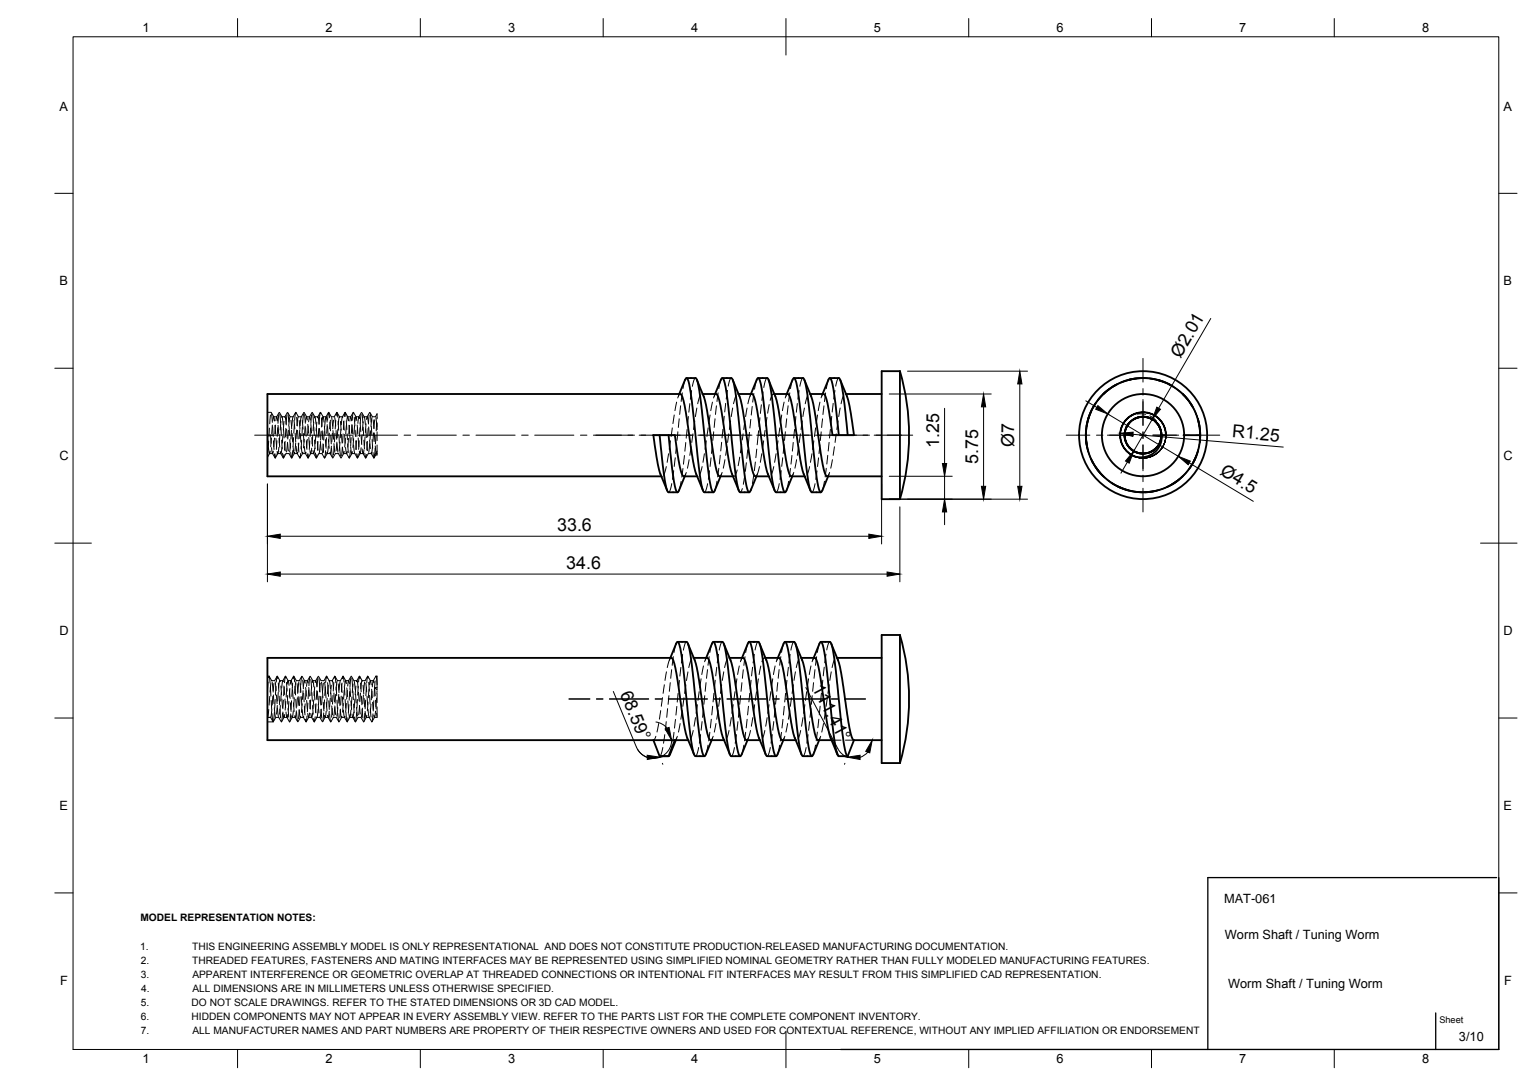
ISO-10303-21;
HEADER;
/* Generated by software containing ST-Developer
 * from STEP Tools, Inc. (www.steptools.com) 
 */

FILE_DESCRIPTION(
/* description */ ('', 'CAx-IF Rec.Pracs.---Representation and Presentation of Product Manufa
cturing Information (PMI)---4.0---2014-10-13'),
/* implementation_level */ '2;1');

FILE_NAME(
/* name */ 'Worm Shaft _ Tuning Worm.step',
/* time_stamp */ '2026-10-28T14:45:12+01:00',
/* author */ (''),
/* organization */ (''),
/* preprocessor_version */ 'ST-DEVELOPER v20.2',
/* originating_system */ 'Autodesk Translation Framework v15.17.0.0',
/* authorisation */ '');

FILE_SCHEMA (('AP242_MANAGED_MODEL_BASED_3D_ENGINEERING_MIM_LF { 1 0 10303 442 2 1 4 }'));
ENDSEC;

DATA;
#10=MECHANICAL_DESIGN_GEOMETRIC_PRESENTATION_REPRESENTATION('',(#258),#52164);
#232=SHAPE_REPRESENTATION_RELATIONSHIP('SRR','None',#52211,#245);
#245=ADVANCED_BREP_SHAPE_REPRESENTATION('',(#271),#52151);
#258=STYLED_ITEM('',(#52318),#271);
#271=MANIFOLD_SOLID_BREP('Body1',#9118);
#284=SPHERICAL_SURFACE('',#9300,12.5);
#288=FACE_BOUND('',#1072,.T.);
#289=FACE_BOUND('',#1091,.T.);
#323=B_SPLINE_SURFACE_WITH_KNOTS('',3,3,((#13144,#13145,#13146,#13147,#13148,
#13149,#13150,#13151,#13152,#13153,#13154,#13155,#13156,#13157,#13158,#13159,
#13160,#13161,#13162,#13163,#13164,#13165,#13166,#13167,#13168,#13169,#13170,
#13171,#13172,#13173,#13174,#13175,#13176,#13177,#13178),(#13179,#13180,
#13181,#13182,#13183,#13184,#13185,#13186,#13187,#13188,#13189,#13190,#13191,
#13192,#13193,#13194,#13195,#13196,#13197,#13198,#13199,#13200,#13201,#13202,
#13203,#13204,#13205,#13206,#13207,#13208,#13209,#13210,#13211,#13212,#13213),
(#13214,#13215,#13216,#13217,#13218,#13219,#13220,#13221,#13222,#13223,
#13224,#13225,#13226,#13227,#13228,#13229,#13230,#13231,#13232,#13233,#13234,
#13235,#13236,#13237,#13238,#13239,#13240,#13241,#13242,#13243,#13244,#13245,
#13246,#13247,#13248),(#13249,#13250,#13251,#13252,#13253,#13254,#13255,
#13256,#13257,#13258,#13259,#13260,#13261,#13262,#13263,#13264,#13265,#13266,
#13267,#13268,#13269,#13270,#13271,#13272,#13273,#13274,#13275,#13276,#13277,
#13278,#13279,#13280,#13281,#13282,#13283)),.UNSPECIFIED.,.F.,.F.,.F.,(4,
4),(4,1,1,1,1,1,1,1,1,1,1,1,1,1,1,1,1,1,1,1,1,1,1,1,1,1,1,1,1,1,1,1,4),
(0.3338579451982,1.029778418438),(-0.02,0.0125,0.045,0.0775,0.11,0.1425,
0.175,0.2075,0.24,0.2725,0.305,0.3375,0.37,0.4025,0.435,0.4675,0.5,0.5325,
0.565,0.5975,0.63,0.6625,0.695,0.7275,0.76,0.7925,0.825,0.8575,0.89,0.9225,
0.955,0.9875,1.02),.UNSPECIFIED.);
#324=B_SPLINE_SURFACE_WITH_KNOTS('',3,3,((#13372,#13373,#13374,#13375,#13376,
#13377,#13378,#13379,#13380,#13381,#13382,#13383,#13384,#13385,#13386,#13387,
#13388,#13389,#13390,#13391,#13392,#13393,#13394,#13395,#13396,#13397,#13398,
#13399,#13400,#13401,#13402,#13403,#13404,#13405,#13406),(#13407,#13408,
#13409,#13410,#13411,#13412,#13413,#13414,#13415,#13416,#13417,#13418,#13419,
#13420,#13421,#13422,#13423,#13424,#13425,#13426,#13427,#13428,#13429,#13430,
#13431,#13432,#13433,#13434,#13435,#13436,#13437,#13438,#13439,#13440,#13441),
(#13442,#13443,#13444,#13445,#13446,#13447,#13448,#13449,#13450,#13451,
#13452,#13453,#13454,#13455,#13456,#13457,#13458,#13459,#13460,#13461,#13462,
#13463,#13464,#13465,#13466,#13467,#13468,#13469,#13470,#13471,#13472,#13473,
#13474,#13475,#13476),(#13477,#13478,#13479,#13480,#13481,#13482,#13483,
#13484,#13485,#13486,#13487,#13488,#13489,#13490,#13491,#13492,#13493,#13494,
#13495,#13496,#13497,#13498,#13499,#13500,#13501,#13502,#13503,#13504,#13505,
#13506,#13507,#13508,#13509,#13510,#13511)),.UNSPECIFIED.,.F.,.F.,.F.,(4,
4),(4,1,1,1,1,1,1,1,1,1,1,1,1,1,1,1,1,1,1,1,1,1,1,1,1,1,1,1,1,1,1,1,4),
(0.3338579451982,1.029778418438),(-0.02,0.0125,0.045,0.0775,0.11,0.1425,
0.175,0.2075,0.24,0.2725,0.305,0.3375,0.37,0.4025,0.435,0.4675,0.5,0.5325,
0.565,0.5975,0.63,0.6625,0.695,0.7275,0.76,0.7925,0.825,0.8575,0.89,0.9225,
0.955,0.9875,1.02),.UNSPECIFIED.);
#325=B_SPLINE_SURFACE_WITH_KNOTS('',3,3,((#13626,#13627,#13628,#13629,#13630,
#13631,#13632,#13633,#13634,#13635,#13636,#13637,#13638,#13639,#13640,#13641,
#13642,#13643,#13644,#13645,#13646,#13647,#13648,#13649,#13650,#13651,#13652,
#13653,#13654,#13655,#13656,#13657,#13658,#13659,#13660),(#13661,#13662,
#13663,#13664,#13665,#13666,#13667,#13668,#13669,#13670,#13671,#13672,#13673,
#13674,#13675,#13676,#13677,#13678,#13679,#13680,#13681,#13682,#13683,#13684,
#13685,#13686,#13687,#13688,#13689,#13690,#13691,#13692,#13693,#13694,#13695),
(#13696,#13697,#13698,#13699,#13700,#13701,#13702,#13703,#13704,#13705,
#13706,#13707,#13708,#13709,#13710,#13711,#13712,#13713,#13714,#13715,#13716,
#13717,#13718,#13719,#13720,#13721,#13722,#13723,#13724,#13725,#13726,#13727,
#13728,#13729,#13730),(#13731,#13732,#13733,#13734,#13735,#13736,#13737,
#13738,#13739,#13740,#13741,#13742,#13743,#13744,#13745,#13746,#13747,#13748,
#13749,#13750,#13751,#13752,#13753,#13754,#13755,#13756,#13757,#13758,#13759,
#13760,#13761,#13762,#13763,#13764,#13765)),.UNSPECIFIED.,.F.,.F.,.F.,(4,
4),(4,1,1,1,1,1,1,1,1,1,1,1,1,1,1,1,1,1,1,1,1,1,1,1,1,1,1,1,1,1,1,1,4),
(-0.02977841843818,0.6661420548018),(-0.02,0.0125,0.045,0.0775,0.11,0.1425,
0.175,0.2075,0.24,0.2725,0.305,0.3375,0.37,0.4025,0.435,0.4675,0.5,0.5325,
0.565,0.5975,0.63,0.6625,0.695,0.7275,0.76,0.7925,0.825,0.8575,0.89,0.9225,
0.955,0.9875,1.02),.UNSPECIFIED.);
#326=B_SPLINE_SURFACE_WITH_KNOTS('',3,3,((#13854,#13855,#13856,#13857,#13858,
#13859,#13860,#13861,#13862,#13863,#13864,#13865,#13866,#13867,#13868,#13869,
#13870,#13871,#13872,#13873,#13874,#13875,#13876,#13877,#13878,#13879,#13880,
#13881,#13882,#13883,#13884,#13885,#13886,#13887,#13888),(#13889,#13890,
#13891,#13892,#13893,#13894,#13895,#13896,#13897,#13898,#13899,#13900,#13901,
#13902,#13903,#13904,#13905,#13906,#13907,#13908,#13909,#13910,#13911,#13912,
#13913,#13914,#13915,#13916,#13917,#13918,#13919,#13920,#13921,#13922,#13923),
(#13924,#13925,#13926,#13927,#13928,#13929,#13930,#13931,#13932,#13933,
#13934,#13935,#13936,#13937,#13938,#13939,#13940,#13941,#13942,#13943,#13944,
#13945,#13946,#13947,#13948,#13949,#13950,#13951,#13952,#13953,#13954,#13955,
#13956,#13957,#13958),(#13959,#13960,#13961,#13962,#13963,#13964,#13965,
#13966,#13967,#13968,#13969,#13970,#13971,#13972,#13973,#13974,#13975,#13976,
#13977,#13978,#13979,#13980,#13981,#13982,#13983,#13984,#13985,#13986,#13987,
#13988,#13989,#13990,#13991,#13992,#13993)),.UNSPECIFIED.,.F.,.F.,.F.,(4,
4),(4,1,1,1,1,1,1,1,1,1,1,1,1,1,1,1,1,1,1,1,1,1,1,1,1,1,1,1,1,1,1,1,4),
(-0.02977841843818,0.6661420548018),(-0.02,0.0125,0.045,0.0775,0.11,0.1425,
0.175,0.2075,0.24,0.2725,0.305,0.3375,0.37,0.4025,0.435,0.4675,0.5,0.5325,
0.565,0.5975,0.63,0.6625,0.695,0.7275,0.76,0.7925,0.825,0.8575,0.89,0.9225,
0.955,0.9875,1.02),.UNSPECIFIED.);
#327=B_SPLINE_SURFACE_WITH_KNOTS('',3,3,((#14080,#14081,#14082,#14083,#14084,
#14085,#14086,#14087,#14088,#14089,#14090,#14091,#14092,#14093,#14094,#14095,
#14096,#14097,#14098,#14099,#14100,#14101,#14102,#14103,#14104,#14105,#14106,
#14107,#14108,#14109,#14110,#14111,#14112,#14113,#14114),(#14115,#14116,
#14117,#14118,#14119,#14120,#14121,#14122,#14123,#14124,#14125,#14126,#14127,
#14128,#14129,#14130,#14131,#14132,#14133,#14134,#14135,#14136,#14137,#14138,
#14139,#14140,#14141,#14142,#14143,#14144,#14145,#14146,#14147,#14148,#14149),
(#14150,#14151,#14152,#14153,#14154,#14155,#14156,#14157,#14158,#14159,
#14160,#14161,#14162,#14163,#14164,#14165,#14166,#14167,#14168,#14169,#14170,
#14171,#14172,#14173,#14174,#14175,#14176,#14177,#14178,#14179,#14180,#14181,
#14182,#14183,#14184),(#14185,#14186,#14187,#14188,#14189,#14190,#14191,
#14192,#14193,#14194,#14195,#14196,#14197,#14198,#14199,#14200,#14201,#14202,
#14203,#14204,#14205,#14206,#14207,#14208,#14209,#14210,#14211,#14212,#14213,
#14214,#14215,#14216,#14217,#14218,#14219)),.UNSPECIFIED.,.F.,.F.,.F.,(4,
4),(4,1,1,1,1,1,1,1,1,1,1,1,1,1,1,1,1,1,1,1,1,1,1,1,1,1,1,1,1,1,1,1,4),
(-0.1795055630679,1.179505563068),(-0.02,0.0125,0.045,0.0775,0.11,0.1425,
0.175,0.2075,0.24,0.2725,0.305,0.3375,0.37,0.4025,0.435,0.4675,0.5,0.5325,
0.565,0.5975,0.63,0.6625,0.695,0.7275,0.76,0.7925,0.825,0.8575,0.89,0.9225,
0.955,0.9875,1.02),.UNSPECIFIED.);
#328=B_SPLINE_SURFACE_WITH_KNOTS('',3,3,((#14625,#14626,#14627,#14628,#14629,
#14630,#14631,#14632,#14633,#14634,#14635,#14636,#14637,#14638,#14639,#14640,
#14641,#14642,#14643,#14644,#14645,#14646,#14647,#14648,#14649,#14650,#14651,
#14652,#14653,#14654,#14655,#14656,#14657,#14658,#14659),(#14660,#14661,
#14662,#14663,#14664,#14665,#14666,#14667,#14668,#14669,#14670,#14671,#14672,
#14673,#14674,#14675,#14676,#14677,#14678,#14679,#14680,#14681,#14682,#14683,
#14684,#14685,#14686,#14687,#14688,#14689,#14690,#14691,#14692,#14693,#14694),
(#14695,#14696,#14697,#14698,#14699,#14700,#14701,#14702,#14703,#14704,
#14705,#14706,#14707,#14708,#14709,#14710,#14711,#14712,#14713,#14714,#14715,
#14716,#14717,#14718,#14719,#14720,#14721,#14722,#14723,#14724,#14725,#14726,
#14727,#14728,#14729),(#14730,#14731,#14732,#14733,#14734,#14735,#14736,
#14737,#14738,#14739,#14740,#14741,#14742,#14743,#14744,#14745,#14746,#14747,
#14748,#14749,#14750,#14751,#14752,#14753,#14754,#14755,#14756,#14757,#14758,
#14759,#14760,#14761,#14762,#14763,#14764)),.UNSPECIFIED.,.F.,.F.,.F.,(4,
4),(4,1,1,1,1,1,1,1,1,1,1,1,1,1,1,1,1,1,1,1,1,1,1,1,1,1,1,1,1,1,1,1,4),
(-0.1795055630679,1.179505563068),(-0.02,0.0125,0.045,0.0775,0.11,0.1425,
0.175,0.2075,0.24,0.2725,0.305,0.3375,0.37,0.4025,0.435,0.4675,0.5,0.5325,
0.565,0.5975,0.63,0.6625,0.695,0.7275,0.76,0.7925,0.825,0.8575,0.89,0.9225,
0.955,0.9875,1.02),.UNSPECIFIED.);
#329=B_SPLINE_SURFACE_WITH_KNOTS('',3,3,((#14766,#14767,#14768,#14769,#14770,
#14771,#14772,#14773,#14774,#14775,#14776,#14777,#14778,#14779,#14780,#14781,
#14782,#14783,#14784,#14785,#14786,#14787,#14788,#14789,#14790,#14791,#14792,
#14793,#14794,#14795,#14796,#14797,#14798,#14799,#14800),(#14801,#14802,
#14803,#14804,#14805,#14806,#14807,#14808,#14809,#14810,#14811,#14812,#14813,
#14814,#14815,#14816,#14817,#14818,#14819,#14820,#14821,#14822,#14823,#14824,
#14825,#14826,#14827,#14828,#14829,#14830,#14831,#14832,#14833,#14834,#14835),
(#14836,#14837,#14838,#14839,#14840,#14841,#14842,#14843,#14844,#14845,
#14846,#14847,#14848,#14849,#14850,#14851,#14852,#14853,#14854,#14855,#14856,
#14857,#14858,#14859,#14860,#14861,#14862,#14863,#14864,#14865,#14866,#14867,
#14868,#14869,#14870),(#14871,#14872,#14873,#14874,#14875,#14876,#14877,
#14878,#14879,#14880,#14881,#14882,#14883,#14884,#14885,#14886,#14887,#14888,
#14889,#14890,#14891,#14892,#14893,#14894,#14895,#14896,#14897,#14898,#14899,
#14900,#14901,#14902,#14903,#14904,#14905)),.UNSPECIFIED.,.F.,.F.,.F.,(4,
4),(4,1,1,1,1,1,1,1,1,1,1,1,1,1,1,1,1,1,1,1,1,1,1,1,1,1,1,1,1,1,1,1,4),
(-0.1795055630679,1.179505563068),(-0.02,0.0125,0.045,0.0775,0.11,0.1425,
0.175,0.2075,0.24,0.2725,0.305,0.3375,0.37,0.4025,0.435,0.4675,0.5,0.5325,
0.565,0.5975,0.63,0.6625,0.695,0.7275,0.76,0.7925,0.825,0.8575,0.89,0.9225,
0.955,0.9875,1.02),.UNSPECIFIED.);
#330=B_SPLINE_SURFACE_WITH_KNOTS('',3,3,((#15309,#15310,#15311,#15312,#15313,
#15314,#15315,#15316,#15317,#15318,#15319,#15320,#15321,#15322,#15323,#15324,
#15325,#15326,#15327,#15328,#15329,#15330,#15331,#15332,#15333,#15334,#15335,
#15336,#15337,#15338,#15339,#15340,#15341,#15342,#15343),(#15344,#15345,
#15346,#15347,#15348,#15349,#15350,#15351,#15352,#15353,#15354,#15355,#15356,
#15357,#15358,#15359,#15360,#15361,#15362,#15363,#15364,#15365,#15366,#15367,
#15368,#15369,#15370,#15371,#15372,#15373,#15374,#15375,#15376,#15377,#15378),
(#15379,#15380,#15381,#15382,#15383,#15384,#15385,#15386,#15387,#15388,
#15389,#15390,#15391,#15392,#15393,#15394,#15395,#15396,#15397,#15398,#15399,
#15400,#15401,#15402,#15403,#15404,#15405,#15406,#15407,#15408,#15409,#15410,
#15411,#15412,#15413),(#15414,#15415,#15416,#15417,#15418,#15419,#15420,
#15421,#15422,#15423,#15424,#15425,#15426,#15427,#15428,#15429,#15430,#15431,
#15432,#15433,#15434,#15435,#15436,#15437,#15438,#15439,#15440,#15441,#15442,
#15443,#15444,#15445,#15446,#15447,#15448)),.UNSPECIFIED.,.F.,.F.,.F.,(4,
4),(4,1,1,1,1,1,1,1,1,1,1,1,1,1,1,1,1,1,1,1,1,1,1,1,1,1,1,1,1,1,1,1,4),
(-0.1795055630679,1.179505563068),(-0.02,0.0125,0.045,0.0775,0.11,0.1425,
0.175,0.2075,0.24,0.2725,0.305,0.3375,0.37,0.4025,0.435,0.4675,0.5,0.5325,
0.565,0.5975,0.63,0.6625,0.695,0.7275,0.76,0.7925,0.825,0.8575,0.89,0.9225,
0.955,0.9875,1.02),.UNSPECIFIED.);
#331=B_SPLINE_SURFACE_WITH_KNOTS('',3,3,((#15538,#15539,#15540,#15541,#15542,
#15543,#15544,#15545,#15546,#15547,#15548,#15549,#15550,#15551,#15552,#15553,
#15554,#15555,#15556,#15557,#15558,#15559,#15560,#15561,#15562,#15563,#15564,
#15565,#15566,#15567,#15568,#15569,#15570,#15571,#15572),(#15573,#15574,
#15575,#15576,#15577,#15578,#15579,#15580,#15581,#15582,#15583,#15584,#15585,
#15586,#15587,#15588,#15589,#15590,#15591,#15592,#15593,#15594,#15595,#15596,
#15597,#15598,#15599,#15600,#15601,#15602,#15603,#15604,#15605,#15606,#15607),
(#15608,#15609,#15610,#15611,#15612,#15613,#15614,#15615,#15616,#15617,
#15618,#15619,#15620,#15621,#15622,#15623,#15624,#15625,#15626,#15627,#15628,
#15629,#15630,#15631,#15632,#15633,#15634,#15635,#15636,#15637,#15638,#15639,
#15640,#15641,#15642),(#15643,#15644,#15645,#15646,#15647,#15648,#15649,
#15650,#15651,#15652,#15653,#15654,#15655,#15656,#15657,#15658,#15659,#15660,
#15661,#15662,#15663,#15664,#15665,#15666,#15667,#15668,#15669,#15670,#15671,
#15672,#15673,#15674,#15675,#15676,#15677)),.UNSPECIFIED.,.F.,.F.,.F.,(4,
4),(4,1,1,1,1,1,1,1,1,1,1,1,1,1,1,1,1,1,1,1,1,1,1,1,1,1,1,1,1,1,1,1,4),
(-0.1560934940397,1.15609349404),(-0.02,0.0125,0.045,0.0775,0.11,0.1425,
0.175,0.2075,0.24,0.2725,0.305,0.3375,0.37,0.4025,0.435,0.4675,0.5,0.5325,
0.565,0.5975,0.63,0.6625,0.695,0.7275,0.76,0.7925,0.825,0.8575,0.89,0.9225,
0.955,0.9875,1.02),.UNSPECIFIED.);
#332=B_SPLINE_SURFACE_WITH_KNOTS('',3,3,((#15921,#15922,#15923,#15924,#15925,
#15926,#15927,#15928,#15929,#15930,#15931,#15932,#15933,#15934,#15935,#15936,
#15937,#15938,#15939,#15940,#15941,#15942,#15943,#15944,#15945,#15946,#15947,
#15948,#15949,#15950,#15951,#15952,#15953,#15954,#15955),(#15956,#15957,
#15958,#15959,#15960,#15961,#15962,#15963,#15964,#15965,#15966,#15967,#15968,
#15969,#15970,#15971,#15972,#15973,#15974,#15975,#15976,#15977,#15978,#15979,
#15980,#15981,#15982,#15983,#15984,#15985,#15986,#15987,#15988,#15989,#15990),
(#15991,#15992,#15993,#15994,#15995,#15996,#15997,#15998,#15999,#16000,
#16001,#16002,#16003,#16004,#16005,#16006,#16007,#16008,#16009,#16010,#16011,
#16012,#16013,#16014,#16015,#16016,#16017,#16018,#16019,#16020,#16021,#16022,
#16023,#16024,#16025),(#16026,#16027,#16028,#16029,#16030,#16031,#16032,
#16033,#16034,#16035,#16036,#16037,#16038,#16039,#16040,#16041,#16042,#16043,
#16044,#16045,#16046,#16047,#16048,#16049,#16050,#16051,#16052,#16053,#16054,
#16055,#16056,#16057,#16058,#16059,#16060)),.UNSPECIFIED.,.F.,.F.,.F.,(4,
4),(4,1,1,1,1,1,1,1,1,1,1,1,1,1,1,1,1,1,1,1,1,1,1,1,1,1,1,1,1,1,1,1,4),
(-0.1560934940397,1.15609349404),(-0.02,0.0125,0.045,0.0775,0.11,0.1425,
0.175,0.2075,0.24,0.2725,0.305,0.3375,0.37,0.4025,0.435,0.4675,0.5,0.5325,
0.565,0.5975,0.63,0.6625,0.695,0.7275,0.76,0.7925,0.825,0.8575,0.89,0.9225,
0.955,0.9875,1.02),.UNSPECIFIED.);
#333=B_SPLINE_SURFACE_WITH_KNOTS('',3,3,((#16228,#16229,#16230,#16231,#16232,
#16233,#16234,#16235,#16236,#16237,#16238,#16239,#16240,#16241,#16242,#16243,
#16244,#16245,#16246,#16247,#16248,#16249,#16250,#16251,#16252,#16253,#16254,
#16255,#16256,#16257,#16258,#16259,#16260,#16261,#16262),(#16263,#16264,
#16265,#16266,#16267,#16268,#16269,#16270,#16271,#16272,#16273,#16274,#16275,
#16276,#16277,#16278,#16279,#16280,#16281,#16282,#16283,#16284,#16285,#16286,
#16287,#16288,#16289,#16290,#16291,#16292,#16293,#16294,#16295,#16296,#16297),
(#16298,#16299,#16300,#16301,#16302,#16303,#16304,#16305,#16306,#16307,
#16308,#16309,#16310,#16311,#16312,#16313,#16314,#16315,#16316,#16317,#16318,
#16319,#16320,#16321,#16322,#16323,#16324,#16325,#16326,#16327,#16328,#16329,
#16330,#16331,#16332),(#16333,#16334,#16335,#16336,#16337,#16338,#16339,
#16340,#16341,#16342,#16343,#16344,#16345,#16346,#16347,#16348,#16349,#16350,
#16351,#16352,#16353,#16354,#16355,#16356,#16357,#16358,#16359,#16360,#16361,
#16362,#16363,#16364,#16365,#16366,#16367)),.UNSPECIFIED.,.F.,.F.,.F.,(4,
4),(4,1,1,1,1,1,1,1,1,1,1,1,1,1,1,1,1,1,1,1,1,1,1,1,1,1,1,1,1,1,1,1,4),
(-0.2613852056804,1.26138520568),(-0.02,0.0125,0.045,0.0775,0.11,0.1425,
0.175,0.2075,0.24,0.2725,0.305,0.3375,0.37,0.4025,0.435,0.4675,0.5,0.5325,
0.565,0.5975,0.63,0.6625,0.695,0.7275,0.76,0.7925,0.825,0.8575,0.89,0.9225,
0.955,0.9875,1.02),.UNSPECIFIED.);
#334=B_SPLINE_SURFACE_WITH_KNOTS('',3,3,((#16369,#16370,#16371,#16372,#16373,
#16374,#16375,#16376,#16377,#16378,#16379,#16380,#16381,#16382,#16383,#16384,
#16385,#16386,#16387,#16388,#16389,#16390,#16391,#16392,#16393,#16394,#16395,
#16396,#16397,#16398,#16399,#16400,#16401,#16402,#16403),(#16404,#16405,
#16406,#16407,#16408,#16409,#16410,#16411,#16412,#16413,#16414,#16415,#16416,
#16417,#16418,#16419,#16420,#16421,#16422,#16423,#16424,#16425,#16426,#16427,
#16428,#16429,#16430,#16431,#16432,#16433,#16434,#16435,#16436,#16437,#16438),
(#16439,#16440,#16441,#16442,#16443,#16444,#16445,#16446,#16447,#16448,
#16449,#16450,#16451,#16452,#16453,#16454,#16455,#16456,#16457,#16458,#16459,
#16460,#16461,#16462,#16463,#16464,#16465,#16466,#16467,#16468,#16469,#16470,
#16471,#16472,#16473),(#16474,#16475,#16476,#16477,#16478,#16479,#16480,
#16481,#16482,#16483,#16484,#16485,#16486,#16487,#16488,#16489,#16490,#16491,
#16492,#16493,#16494,#16495,#16496,#16497,#16498,#16499,#16500,#16501,#16502,
#16503,#16504,#16505,#16506,#16507,#16508)),.UNSPECIFIED.,.F.,.F.,.F.,(4,
4),(4,1,1,1,1,1,1,1,1,1,1,1,1,1,1,1,1,1,1,1,1,1,1,1,1,1,1,1,1,1,1,1,4),
(-0.2613852056804,1.26138520568),(-0.02,0.0125,0.045,0.0775,0.11,0.1425,
0.175,0.2075,0.24,0.2725,0.305,0.3375,0.37,0.4025,0.435,0.4675,0.5,0.5325,
0.565,0.5975,0.63,0.6625,0.695,0.7275,0.76,0.7925,0.825,0.8575,0.89,0.9225,
0.955,0.9875,1.02),.UNSPECIFIED.);
#335=B_SPLINE_SURFACE_WITH_KNOTS('',3,3,((#16732,#16733,#16734,#16735,#16736,
#16737,#16738,#16739,#16740,#16741,#16742,#16743,#16744,#16745,#16746,#16747,
#16748,#16749,#16750,#16751,#16752,#16753,#16754,#16755,#16756,#16757,#16758,
#16759,#16760,#16761,#16762,#16763,#16764,#16765,#16766),(#16767,#16768,
#16769,#16770,#16771,#16772,#16773,#16774,#16775,#16776,#16777,#16778,#16779,
#16780,#16781,#16782,#16783,#16784,#16785,#16786,#16787,#16788,#16789,#16790,
#16791,#16792,#16793,#16794,#16795,#16796,#16797,#16798,#16799,#16800,#16801),
(#16802,#16803,#16804,#16805,#16806,#16807,#16808,#16809,#16810,#16811,
#16812,#16813,#16814,#16815,#16816,#16817,#16818,#16819,#16820,#16821,#16822,
#16823,#16824,#16825,#16826,#16827,#16828,#16829,#16830,#16831,#16832,#16833,
#16834,#16835,#16836),(#16837,#16838,#16839,#16840,#16841,#16842,#16843,
#16844,#16845,#16846,#16847,#16848,#16849,#16850,#16851,#16852,#16853,#16854,
#16855,#16856,#16857,#16858,#16859,#16860,#16861,#16862,#16863,#16864,#16865,
#16866,#16867,#16868,#16869,#16870,#16871)),.UNSPECIFIED.,.F.,.F.,.F.,(4,
4),(4,1,1,1,1,1,1,1,1,1,1,1,1,1,1,1,1,1,1,1,1,1,1,1,1,1,1,1,1,1,1,1,4),
(-0.1560934940397,1.15609349404),(-0.02,0.0125,0.045,0.0775,0.11,0.1425,
0.175,0.2075,0.24,0.2725,0.305,0.3375,0.37,0.4025,0.435,0.4675,0.5,0.5325,
0.565,0.5975,0.63,0.6625,0.695,0.7275,0.76,0.7925,0.825,0.8575,0.89,0.9225,
0.955,0.9875,1.02),.UNSPECIFIED.);
#336=B_SPLINE_SURFACE_WITH_KNOTS('',3,3,((#17004,#17005,#17006,#17007,#17008,
#17009,#17010,#17011,#17012,#17013,#17014,#17015,#17016,#17017,#17018,#17019,
#17020,#17021,#17022,#17023,#17024,#17025,#17026,#17027,#17028,#17029,#17030,
#17031,#17032,#17033,#17034,#17035,#17036,#17037,#17038),(#17039,#17040,
#17041,#17042,#17043,#17044,#17045,#17046,#17047,#17048,#17049,#17050,#17051,
#17052,#17053,#17054,#17055,#17056,#17057,#17058,#17059,#17060,#17061,#17062,
#17063,#17064,#17065,#17066,#17067,#17068,#17069,#17070,#17071,#17072,#17073),
(#17074,#17075,#17076,#17077,#17078,#17079,#17080,#17081,#17082,#17083,
#17084,#17085,#17086,#17087,#17088,#17089,#17090,#17091,#17092,#17093,#17094,
#17095,#17096,#17097,#17098,#17099,#17100,#17101,#17102,#17103,#17104,#17105,
#17106,#17107,#17108),(#17109,#17110,#17111,#17112,#17113,#17114,#17115,
#17116,#17117,#17118,#17119,#17120,#17121,#17122,#17123,#17124,#17125,#17126,
#17127,#17128,#17129,#17130,#17131,#17132,#17133,#17134,#17135,#17136,#17137,
#17138,#17139,#17140,#17141,#17142,#17143)),.UNSPECIFIED.,.F.,.F.,.F.,(4,
4),(4,1,1,1,1,1,1,1,1,1,1,1,1,1,1,1,1,1,1,1,1,1,1,1,1,1,1,1,1,1,1,1,4),
(-0.1560934940397,1.15609349404),(-0.02,0.0125,0.045,0.0775,0.11,0.1425,
0.175,0.2075,0.24,0.2725,0.305,0.3375,0.37,0.4025,0.435,0.4675,0.5,0.5325,
0.565,0.5975,0.63,0.6625,0.695,0.7275,0.76,0.7925,0.825,0.8575,0.89,0.9225,
0.955,0.9875,1.02),.UNSPECIFIED.);
#337=B_SPLINE_SURFACE_WITH_KNOTS('',3,3,((#17202,#17203,#17204,#17205,#17206,
#17207,#17208,#17209,#17210,#17211,#17212,#17213,#17214,#17215,#17216,#17217,
#17218,#17219,#17220,#17221,#17222,#17223,#17224,#17225,#17226,#17227,#17228,
#17229,#17230,#17231,#17232,#17233,#17234,#17235,#17236),(#17237,#17238,
#17239,#17240,#17241,#17242,#17243,#17244,#17245,#17246,#17247,#17248,#17249,
#17250,#17251,#17252,#17253,#17254,#17255,#17256,#17257,#17258,#17259,#17260,
#17261,#17262,#17263,#17264,#17265,#17266,#17267,#17268,#17269,#17270,#17271),
(#17272,#17273,#17274,#17275,#17276,#17277,#17278,#17279,#17280,#17281,
#17282,#17283,#17284,#17285,#17286,#17287,#17288,#17289,#17290,#17291,#17292,
#17293,#17294,#17295,#17296,#17297,#17298,#17299,#17300,#17301,#17302,#17303,
#17304,#17305,#17306),(#17307,#17308,#17309,#17310,#17311,#17312,#17313,
#17314,#17315,#17316,#17317,#17318,#17319,#17320,#17321,#17322,#17323,#17324,
#17325,#17326,#17327,#17328,#17329,#17330,#17331,#17332,#17333,#17334,#17335,
#17336,#17337,#17338,#17339,#17340,#17341)),.UNSPECIFIED.,.F.,.F.,.F.,(4,
4),(4,1,1,1,1,1,1,1,1,1,1,1,1,1,1,1,1,1,1,1,1,1,1,1,1,1,1,1,1,1,1,1,4),
(-0.1560934940397,1.15609349404),(-0.02,0.0125,0.045,0.0775,0.11,0.1425,
0.175,0.2075,0.24,0.2725,0.305,0.3375,0.37,0.4025,0.435,0.4675,0.5,0.5325,
0.565,0.5975,0.63,0.6625,0.695,0.7275,0.76,0.7925,0.825,0.8575,0.89,0.9225,
0.955,0.9875,1.02),.UNSPECIFIED.);
#338=B_SPLINE_SURFACE_WITH_KNOTS('',3,3,((#17618,#17619,#17620,#17621,#17622,
#17623,#17624,#17625,#17626,#17627,#17628,#17629,#17630,#17631,#17632,#17633,
#17634,#17635,#17636,#17637,#17638,#17639,#17640,#17641,#17642,#17643,#17644,
#17645,#17646,#17647,#17648,#17649,#17650,#17651,#17652),(#17653,#17654,
#17655,#17656,#17657,#17658,#17659,#17660,#17661,#17662,#17663,#17664,#17665,
#17666,#17667,#17668,#17669,#17670,#17671,#17672,#17673,#17674,#17675,#17676,
#17677,#17678,#17679,#17680,#17681,#17682,#17683,#17684,#17685,#17686,#17687),
(#17688,#17689,#17690,#17691,#17692,#17693,#17694,#17695,#17696,#17697,
#17698,#17699,#17700,#17701,#17702,#17703,#17704,#17705,#17706,#17707,#17708,
#17709,#17710,#17711,#17712,#17713,#17714,#17715,#17716,#17717,#17718,#17719,
#17720,#17721,#17722),(#17723,#17724,#17725,#17726,#17727,#17728,#17729,
#17730,#17731,#17732,#17733,#17734,#17735,#17736,#17737,#17738,#17739,#17740,
#17741,#17742,#17743,#17744,#17745,#17746,#17747,#17748,#17749,#17750,#17751,
#17752,#17753,#17754,#17755,#17756,#17757)),.UNSPECIFIED.,.F.,.F.,.F.,(4,
4),(4,1,1,1,1,1,1,1,1,1,1,1,1,1,1,1,1,1,1,1,1,1,1,1,1,1,1,1,1,1,1,1,4),
(-0.1560934940397,1.15609349404),(-0.02,0.0125,0.045,0.0775,0.11,0.1425,
0.175,0.2075,0.24,0.2725,0.305,0.3375,0.37,0.4025,0.435,0.4675,0.5,0.5325,
0.565,0.5975,0.63,0.6625,0.695,0.7275,0.76,0.7925,0.825,0.8575,0.89,0.9225,
0.955,0.9875,1.02),.UNSPECIFIED.);
#339=B_SPLINE_SURFACE_WITH_KNOTS('',3,3,((#17870,#17871,#17872,#17873,#17874,
#17875,#17876,#17877,#17878,#17879,#17880,#17881,#17882,#17883,#17884,#17885,
#17886,#17887,#17888,#17889,#17890,#17891,#17892,#17893,#17894,#17895,#17896,
#17897,#17898,#17899,#17900,#17901,#17902,#17903,#17904),(#17905,#17906,
#17907,#17908,#17909,#17910,#17911,#17912,#17913,#17914,#17915,#17916,#17917,
#17918,#17919,#17920,#17921,#17922,#17923,#17924,#17925,#17926,#17927,#17928,
#17929,#17930,#17931,#17932,#17933,#17934,#17935,#17936,#17937,#17938,#17939),
(#17940,#17941,#17942,#17943,#17944,#17945,#17946,#17947,#17948,#17949,
#17950,#17951,#17952,#17953,#17954,#17955,#17956,#17957,#17958,#17959,#17960,
#17961,#17962,#17963,#17964,#17965,#17966,#17967,#17968,#17969,#17970,#17971,
#17972,#17973,#17974),(#17975,#17976,#17977,#17978,#17979,#17980,#17981,
#17982,#17983,#17984,#17985,#17986,#17987,#17988,#17989,#17990,#17991,#17992,
#17993,#17994,#17995,#17996,#17997,#17998,#17999,#18000,#18001,#18002,#18003,
#18004,#18005,#18006,#18007,#18008,#18009)),.UNSPECIFIED.,.F.,.F.,.F.,(4,
4),(4,1,1,1,1,1,1,1,1,1,1,1,1,1,1,1,1,1,1,1,1,1,1,1,1,1,1,1,1,1,1,1,4),
(-0.1560934940397,1.15609349404),(-0.02,0.0125,0.045,0.0775,0.11,0.1425,
0.175,0.2075,0.24,0.2725,0.305,0.3375,0.37,0.4025,0.435,0.4675,0.5,0.5325,
0.565,0.5975,0.63,0.6625,0.695,0.7275,0.76,0.7925,0.825,0.8575,0.89,0.9225,
0.955,0.9875,1.02),.UNSPECIFIED.);
#340=B_SPLINE_SURFACE_WITH_KNOTS('',3,3,((#18261,#18262,#18263,#18264,#18265,
#18266,#18267,#18268,#18269,#18270,#18271,#18272,#18273,#18274,#18275,#18276,
#18277,#18278,#18279,#18280,#18281,#18282,#18283,#18284,#18285,#18286,#18287,
#18288,#18289,#18290,#18291,#18292,#18293,#18294,#18295),(#18296,#18297,
#18298,#18299,#18300,#18301,#18302,#18303,#18304,#18305,#18306,#18307,#18308,
#18309,#18310,#18311,#18312,#18313,#18314,#18315,#18316,#18317,#18318,#18319,
#18320,#18321,#18322,#18323,#18324,#18325,#18326,#18327,#18328,#18329,#18330),
(#18331,#18332,#18333,#18334,#18335,#18336,#18337,#18338,#18339,#18340,
#18341,#18342,#18343,#18344,#18345,#18346,#18347,#18348,#18349,#18350,#18351,
#18352,#18353,#18354,#18355,#18356,#18357,#18358,#18359,#18360,#18361,#18362,
#18363,#18364,#18365),(#18366,#18367,#18368,#18369,#18370,#18371,#18372,
#18373,#18374,#18375,#18376,#18377,#18378,#18379,#18380,#18381,#18382,#18383,
#18384,#18385,#18386,#18387,#18388,#18389,#18390,#18391,#18392,#18393,#18394,
#18395,#18396,#18397,#18398,#18399,#18400)),.UNSPECIFIED.,.F.,.F.,.F.,(4,
4),(4,1,1,1,1,1,1,1,1,1,1,1,1,1,1,1,1,1,1,1,1,1,1,1,1,1,1,1,1,1,1,1,4),
(-0.1560934940397,1.15609349404),(-0.0177116462091,0.01106977888069,0.03985120397047,
0.06863262906025,0.09741405415003,0.1261954792398,0.1549769043296,0.1837583294194,
0.2125397545092,0.2413211795989,0.2701026046887,0.2988840297785,0.3276654548683,
0.3564468799581,0.3852283050479,0.4140097301376,0.4427911552274,0.4715725803172,
0.500354005407,0.5291354304968,0.5579168555866,0.5866982806763,0.6154797057661,
0.6442611308559,0.6730425559457,0.7018239810355,0.7306054061252,0.759386831215,
0.7881682563048,0.8169496813946,0.8457311064844,0.8745125315742,0.9032939566639),
 .UNSPECIFIED.);
#341=B_SPLINE_SURFACE_WITH_KNOTS('',3,3,((#18688,#18689,#18690,#18691,#18692,
#18693,#18694,#18695,#18696,#18697,#18698,#18699,#18700,#18701,#18702,#18703,
#18704,#18705,#18706,#18707,#18708,#18709,#18710,#18711,#18712,#18713,#18714,
#18715,#18716,#18717,#18718,#18719,#18720,#18721,#18722),(#18723,#18724,
#18725,#18726,#18727,#18728,#18729,#18730,#18731,#18732,#18733,#18734,#18735,
#18736,#18737,#18738,#18739,#18740,#18741,#18742,#18743,#18744,#18745,#18746,
#18747,#18748,#18749,#18750,#18751,#18752,#18753,#18754,#18755,#18756,#18757),
(#18758,#18759,#18760,#18761,#18762,#18763,#18764,#18765,#18766,#18767,
#18768,#18769,#18770,#18771,#18772,#18773,#18774,#18775,#18776,#18777,#18778,
#18779,#18780,#18781,#18782,#18783,#18784,#18785,#18786,#18787,#18788,#18789,
#18790,#18791,#18792),(#18793,#18794,#18795,#18796,#18797,#18798,#18799,
#18800,#18801,#18802,#18803,#18804,#18805,#18806,#18807,#18808,#18809,#18810,
#18811,#18812,#18813,#18814,#18815,#18816,#18817,#18818,#18819,#18820,#18821,
#18822,#18823,#18824,#18825,#18826,#18827)),.UNSPECIFIED.,.F.,.F.,.F.,(4,
4),(4,1,1,1,1,1,1,1,1,1,1,1,1,1,1,1,1,1,1,1,1,1,1,1,1,1,1,1,1,1,1,1,4),
(-0.2613852056804,1.26138520568),(-0.01995502045757,0.01247188778598,0.04489879602953,
0.07732570427308,0.1097526125166,0.1421795207602,0.1746064290037,0.2070333372473,
0.2394602454908,0.2718871537344,0.3043140619779,0.3367409702215,0.369167878465,
0.4015947867086,0.4340216949521,0.4664486031957,0.4988755114392,0.5313024196828,
0.5637293279263,0.5961562361699,0.6285831444134,0.661010052657,0.6934369609005,
0.7258638691441,0.7582907773876,0.7907176856312,0.8231445938748,0.8555715021183,
0.8879984103619,0.9204253186054,0.952852226849,0.9852791350925,1.017706043336),
 .UNSPECIFIED.);
#342=B_SPLINE_SURFACE_WITH_KNOTS('',3,3,((#18829,#18830,#18831,#18832,#18833,
#18834,#18835,#18836,#18837,#18838,#18839,#18840,#18841,#18842,#18843,#18844,
#18845,#18846,#18847,#18848,#18849,#18850,#18851,#18852,#18853,#18854,#18855,
#18856,#18857,#18858,#18859,#18860,#18861,#18862,#18863),(#18864,#18865,
#18866,#18867,#18868,#18869,#18870,#18871,#18872,#18873,#18874,#18875,#18876,
#18877,#18878,#18879,#18880,#18881,#18882,#18883,#18884,#18885,#18886,#18887,
#18888,#18889,#18890,#18891,#18892,#18893,#18894,#18895,#18896,#18897,#18898),
(#18899,#18900,#18901,#18902,#18903,#18904,#18905,#18906,#18907,#18908,
#18909,#18910,#18911,#18912,#18913,#18914,#18915,#18916,#18917,#18918,#18919,
#18920,#18921,#18922,#18923,#18924,#18925,#18926,#18927,#18928,#18929,#18930,
#18931,#18932,#18933),(#18934,#18935,#18936,#18937,#18938,#18939,#18940,
#18941,#18942,#18943,#18944,#18945,#18946,#18947,#18948,#18949,#18950,#18951,
#18952,#18953,#18954,#18955,#18956,#18957,#18958,#18959,#18960,#18961,#18962,
#18963,#18964,#18965,#18966,#18967,#18968)),.UNSPECIFIED.,.F.,.F.,.F.,(4,
4),(4,1,1,1,1,1,1,1,1,1,1,1,1,1,1,1,1,1,1,1,1,1,1,1,1,1,1,1,1,1,1,1,4),
(-0.2613852056804,1.26138520568),(-0.02,0.0125,0.045,0.0775,0.11,0.1425,
0.175,0.2075,0.24,0.2725,0.305,0.3375,0.37,0.4025,0.435,0.4675,0.5,0.5325,
0.565,0.5975,0.63,0.6625,0.695,0.7275,0.76,0.7925,0.825,0.8575,0.89,0.9225,
0.955,0.9875,1.02),.UNSPECIFIED.);
#409=PLANE('',#9283);
#410=PLANE('',#9286);
#411=PLANE('',#9287);
#412=PLANE('',#9290);
#413=PLANE('',#9291);
#414=PLANE('',#9293);
#415=PLANE('',#9295);
#518=FACE_OUTER_BOUND('',#1055,.T.);
#519=FACE_OUTER_BOUND('',#1056,.T.);
#520=FACE_OUTER_BOUND('',#1057,.T.);
#521=FACE_OUTER_BOUND('',#1058,.T.);
#522=FACE_OUTER_BOUND('',#1059,.T.);
#523=FACE_OUTER_BOUND('',#1060,.T.);
#524=FACE_OUTER_BOUND('',#1061,.T.);
#525=FACE_OUTER_BOUND('',#1062,.T.);
#526=FACE_OUTER_BOUND('',#1063,.T.);
#527=FACE_OUTER_BOUND('',#1064,.T.);
#528=FACE_OUTER_BOUND('',#1065,.T.);
#529=FACE_OUTER_BOUND('',#1066,.T.);
#530=FACE_OUTER_BOUND('',#1067,.T.);
#531=FACE_OUTER_BOUND('',#1068,.T.);
#532=FACE_OUTER_BOUND('',#1069,.T.);
#533=FACE_OUTER_BOUND('',#1070,.T.);
#534=FACE_OUTER_BOUND('',#1071,.T.);
#535=FACE_OUTER_BOUND('',#1073,.T.);
#536=FACE_OUTER_BOUND('',#1074,.T.);
#537=FACE_OUTER_BOUND('',#1075,.T.);
#538=FACE_OUTER_BOUND('',#1076,.T.);
#539=FACE_OUTER_BOUND('',#1077,.T.);
#540=FACE_OUTER_BOUND('',#1078,.T.);
#541=FACE_OUTER_BOUND('',#1079,.T.);
#542=FACE_OUTER_BOUND('',#1080,.T.);
#543=FACE_OUTER_BOUND('',#1081,.T.);
#544=FACE_OUTER_BOUND('',#1082,.T.);
#545=FACE_OUTER_BOUND('',#1083,.T.);
#546=FACE_OUTER_BOUND('',#1084,.T.);
#547=FACE_OUTER_BOUND('',#1085,.T.);
#548=FACE_OUTER_BOUND('',#1086,.T.);
#549=FACE_OUTER_BOUND('',#1087,.T.);
#550=FACE_OUTER_BOUND('',#1088,.T.);
#551=FACE_OUTER_BOUND('',#1089,.T.);
#552=FACE_OUTER_BOUND('',#1090,.T.);
#553=FACE_OUTER_BOUND('',#1092,.T.);
#554=FACE_OUTER_BOUND('',#1093,.T.);
#1055=EDGE_LOOP('',(#5620,#5621,#5622,#5623,#5624,#5625));
#1056=EDGE_LOOP('',(#5626,#5627,#5628,#5629));
#1057=EDGE_LOOP('',(#5630,#5631,#5632,#5633,#5634));
#1058=EDGE_LOOP('',(#5635,#5636,#5637,#5638,#5639));
#1059=EDGE_LOOP('',(#5640,#5641,#5642,#5643));
#1060=EDGE_LOOP('',(#5644,#5645,#5646,#5647,#5648));
#1061=EDGE_LOOP('',(#5649,#5650,#5651,#5652,#5653,#5654));
#1062=EDGE_LOOP('',(#5655,#5656,#5657,#5658,#5659,#5660));
#1063=EDGE_LOOP('',(#5661,#5662,#5663,#5664,#5665,#5666));
#1064=EDGE_LOOP('',(#5667,#5668,#5669,#5670,#5671));
#1065=EDGE_LOOP('',(#5672,#5673,#5674,#5675,#5676,#5677));
#1066=EDGE_LOOP('',(#5678,#5679,#5680,#5681,#5682,#5683));
#1067=EDGE_LOOP('',(#5684,#5685,#5686,#5687));
#1068=EDGE_LOOP('',(#5688,#5689,#5690,#5691));
#1069=EDGE_LOOP('',(#5692,#5693,#5694,#5695));
#1070=EDGE_LOOP('',(#5696,#5697,#5698,#5699));
#1071=EDGE_LOOP('',(#5700));
#1072=EDGE_LOOP('',(#5701,#5702,#5703,#5704));
#1073=EDGE_LOOP('',(#5705,#5706,#5707));
#1074=EDGE_LOOP('',(#5708,#5709,#5710,#5711,#5712));
#1075=EDGE_LOOP('',(#5713,#5714,#5715,#5716,#5717,#5718,#5719));
#1076=EDGE_LOOP('',(#5720,#5721,#5722,#5723,#5724));
#1077=EDGE_LOOP('',(#5725,#5726,#5727,#5728));
#1078=EDGE_LOOP('',(#5729,#5730,#5731,#5732));
#1079=EDGE_LOOP('',(#5733,#5734,#5735,#5736,#5737));
#1080=EDGE_LOOP('',(#5738,#5739,#5740,#5741,#5742));
#1081=EDGE_LOOP('',(#5743,#5744,#5745,#5746,#5747));
#1082=EDGE_LOOP('',(#5748,#5749,#5750,#5751,#5752));
#1083=EDGE_LOOP('',(#5753,#5754,#5755,#5756,#5757,#5758));
#1084=EDGE_LOOP('',(#5759,#5760,#5761,#5762,#5763));
#1085=EDGE_LOOP('',(#5764,#5765,#5766,#5767,#5768,#5769));
#1086=EDGE_LOOP('',(#5770,#5771,#5772));
#1087=EDGE_LOOP('',(#5773,#5774,#5775));
#1088=EDGE_LOOP('',(#5776,#5777,#5778,#5779,#5780));
#1089=EDGE_LOOP('',(#5781,#5782,#5783,#5784));
#1090=EDGE_LOOP('',(#5785));
#1091=EDGE_LOOP('',(#5786));
#1092=EDGE_LOOP('',(#5787,#5788,#5789,#5790,#5791));
#1093=EDGE_LOOP('',(#5792,#5793,#5794,#5795));
#1627=CIRCLE('',#9278,2.25);
#1628=CIRCLE('',#9285,2.25);
#1629=CIRCLE('',#9288,1.25);
#1630=CIRCLE('',#9292,1.25);
#1631=CIRCLE('',#9296,3.5);
#1632=CIRCLE('',#9298,3.5);
#1633=CIRCLE('',#9299,3.5);
#1634=CIRCLE('',#9301,12.5);
#2094=B_SPLINE_CURVE_WITH_KNOTS('',3,(#12552,#12553,#12554,#12555,#12556,
#12557,#12558,#12559,#12560,#12561,#12562,#12563,#12564,#12565,#12566,#12567,
#12568,#12569,#12570,#12571,#12572,#12573,#12574,#12575,#12576,#12577,#12578,
#12579,#12580,#12581,#12582,#12583,#12584,#12585,#12586,#12587,#12588,#12589,
#12590,#12591,#12592,#12593,#12594,#12595,#12596,#12597,#12598,#12599,#12600,
#12601,#12602,#12603),.UNSPECIFIED.,.F.,.F.,(4,2,2,2,2,2,2,2,2,2,2,2,2,
2,2,2,2,2,2,2,2,2,2,2,2,4),(2.14502562436384,2.18712156060152,2.27622566969401,
2.32089041959239,2.36538765547986,2.45376151983945,2.4982791356259,2.54277391955066,
2.58737028222014,2.67694633287528,2.72140315755377,2.76570334662978,2.85489268765083,
2.89952573822096,2.94404144281776,3.03280270260246,3.07729710502769,3.12175138462939,
3.16636646470874,3.25602651891706,3.30048521246139,3.34474880671133,3.43400504589525,
3.46917173238361,3.52205339439103,3.57498321837689),.UNSPECIFIED.);
#2095=B_SPLINE_CURVE_WITH_KNOTS('',3,(#12612,#12613,#12614,#12615,#12616,
#12617,#12618,#12619,#12620,#12621,#12622,#12623,#12624,#12625,#12626,#12627,
#12628,#12629,#12630,#12631,#12632,#12633,#12634,#12635,#12636,#12637,#12638,
#12639,#12640,#12641,#12642,#12643,#12644,#12645,#12646,#12647,#12648,#12649,
#12650,#12651,#12652,#12653,#12654,#12655,#12656,#12657,#12658,#12659,#12660,
#12661,#12662,#12663,#12664,#12665),.UNSPECIFIED.,.F.,.F.,(4,2,2,2,2,2,
2,2,2,2,2,2,2,2,2,2,2,2,2,2,2,2,2,2,2,2,4),(0.714866971049495,0.72011528738726,
0.809316049507178,0.853618221320616,0.898069747103448,0.987629225690559,
1.03222343976808,1.07672364266554,1.12123519646787,1.2096051565493,1.25409829695009,
1.29876912997362,1.3878844113741,1.43223900550291,1.47669632479167,1.56609535939874,
1.61066571850577,1.65521605463951,1.69976297657141,1.78749336285472,1.87522704043972,
1.91977971115659,1.96432372106055,2.00889621585214,2.09830830202093,2.14277057212069,
2.14502562436384),.UNSPECIFIED.);
#2096=B_SPLINE_CURVE_WITH_KNOTS('',3,(#12666,#12667,#12668,#12669,#12670,
#12671,#12672,#12673,#12674,#12675,#12676,#12677,#12678,#12679,#12680,#12681,
#12682,#12683,#12684,#12685,#12686,#12687,#12688,#12689,#12690,#12691,#12692,
#12693,#12694,#12695,#12696,#12697,#12698,#12699,#12700,#12701,#12702,#12703,
#12704,#12705,#12706,#12707,#12708,#12709,#12710,#12711,#12712,#12713,#12714,
#12715,#12716,#12717),.UNSPECIFIED.,.F.,.F.,(4,2,2,2,2,2,2,2,2,2,2,2,2,
2,2,2,2,2,2,2,2,2,2,2,2,4),(1.0000000638874E-6,0.0529432525790578,0.105836830109484,
0.141014199970554,0.230281459970461,0.274545373941572,0.318998103364306,
0.408638735078214,0.453251377644336,0.497709833041615,0.542197575952712,
0.630949700434586,0.675460895509643,0.720099378845943,0.809300087921693,
0.853602222275693,0.898053716322623,0.98761314604962,1.03220733122512,1.07670749657416,
1.12121901503127,1.20958897541431,1.25408208681528,1.29875288369215,1.3878681140945,
1.4299206384854),.UNSPECIFIED.);
#2097=B_SPLINE_CURVE_WITH_KNOTS('',3,(#12723,#12724,#12725,#12726,#12727,
#12728,#12729,#12730,#12731,#12732,#12733,#12734,#12735,#12736,#12737,#12738,
#12739,#12740,#12741,#12742,#12743,#12744,#12745,#12746,#12747,#12748,#12749,
#12750),.UNSPECIFIED.,.F.,.F.,(4,2,2,2,2,2,2,2,2,2,2,2,2,4),(2.86008561622508,
2.89952817344818,2.94404372203974,3.03280213002521,3.0772967112602,3.12175133798389,
3.1663662648552,3.25602576693473,3.30048442341296,3.34474833908933,3.4340039704133,
3.46917521608883,3.52206341792462,3.57496743915675),.UNSPECIFIED.);
#2098=B_SPLINE_CURVE_WITH_KNOTS('',3,(#12751,#12752,#12753,#12754,#12755,
#12756,#12757,#12758,#12759,#12760,#12761,#12762,#12763,#12764,#12765,#12766,
#12767,#12768,#12769,#12770,#12771,#12772,#12773,#12774,#12775,#12776,#12777,
#12778),.UNSPECIFIED.,.F.,.F.,(4,2,2,2,2,2,2,2,2,2,2,2,2,4),(1.94943175665867E-5,
0.0529485196822737,0.105848261883074,0.141029742242418,0.230297056939625,
0.274561007064076,0.319013767542678,0.408654455292159,0.453267127336578,
0.497725619328092,0.542213396377112,0.630965543886577,0.675476768340537,
0.714866971049495),.UNSPECIFIED.);
#2099=B_SPLINE_CURVE_WITH_KNOTS('',3,(#12779,#12780,#12781,#12782,#12783,
#12784,#12785,#12786,#12787,#12788,#12789,#12790,#12791,#12792,#12793,#12794,
#12795,#12796,#12797,#12798,#12799,#12800,#12801,#12802,#12803,#12804,#12805,
#12806,#12807,#12808,#12809,#12810,#12811,#12812,#12813,#12814,#12815,#12816,
#12817,#12818,#12819,#12820,#12821,#12822,#12823,#12824,#12825,#12826,#12827,
#12828,#12829,#12830,#12831,#12832),.UNSPECIFIED.,.F.,.F.,(4,2,2,2,2,2,
2,2,2,2,2,2,2,2,2,2,2,2,2,2,2,2,2,2,2,2,4),(1.4299206384854,1.43222267048901,
1.47667998786036,1.56607905094836,1.61064941319619,1.65519974160521,1.69974665739337,
1.78747715470346,1.87521086672082,1.91976354413251,1.96430756284278,2.0088800513862,
2.09829209315722,2.1427543640379,2.18710539147204,2.27620954348202,2.3208743295338,
2.36537159165582,2.45374542602367,2.49826307689474,2.54275789886887,2.58735428763111,
2.67693037733929,2.72138723206035,2.76568745901495,2.85487684558239,2.86008592505616),
 .UNSPECIFIED.);
#2100=B_SPLINE_CURVE_WITH_KNOTS('',3,(#12837,#12838,#12839,#12840,#12841,
#12842,#12843,#12844,#12845,#12846,#12847,#12848,#12849,#12850,#12851,#12852,
#12853,#12854,#12855,#12856,#12857,#12858,#12859,#12860,#12861,#12862,#12863,
#12864,#12865,#12866,#12867,#12868,#12869,#12870,#12871,#12872,#12873,#12874,
#12875,#12876,#12877,#12878,#12879,#12880,#12881,#12882,#12883,#12884,#12885,
#12886,#12887,#12888,#12889,#12890),.UNSPECIFIED.,.F.,.F.,(4,2,2,2,2,2,
2,2,2,2,2,2,2,2,2,2,2,2,2,2,2,2,2,2,2,2,4),(1.42992065923686,1.43223977969029,
1.47669703588382,1.56609757048888,1.61066812124717,1.65521810141441,1.69976474727003,
1.787500783217,1.87523625403487,1.91978929642496,1.9643337839075,2.00890599824737,
2.09831591280814,2.14277825682906,2.18712978796684,2.27623305258158,2.32089811540851,
2.36539517067194,2.45376453680926,2.49828241705732,2.54277761521628,2.58737378670215,
2.67694877874516,2.72140561612856,2.76570621753569,2.85489484220979,2.86008561622508),
 .UNSPECIFIED.);
#2101=B_SPLINE_CURVE_WITH_KNOTS('',3,(#12892,#12893,#12894,#12895,#12896,
#12897,#12898,#12899,#12900,#12901,#12902,#12903,#12904,#12905,#12906,#12907,
#12908,#12909,#12910,#12911,#12912,#12913,#12914,#12915,#12916,#12917,#12918,
#12919),.UNSPECIFIED.,.F.,.F.,(4,2,2,2,2,2,2,2,2,2,2,2,2,4),(2.86008592505616,
2.89950993164355,2.94402566297617,3.03278692566152,3.07728136145645,3.1217356777481,
3.16635078468632,3.2560108880428,3.30046961064402,3.3447332409437,3.43398952787311,
3.46916115583476,3.52205022597488,3.5749680558315),.UNSPECIFIED.);
#2102=B_SPLINE_CURVE_WITH_KNOTS('',3,(#12920,#12921,#12922,#12923,#12924,
#12925,#12926,#12927,#12928,#12929,#12930,#12931,#12932,#12933,#12934,#12935,
#12936,#12937,#12938,#12939,#12940,#12941,#12942,#12943,#12944,#12945,#12946,
#12947),.UNSPECIFIED.,.F.,.F.,(4,2,2,2,2,2,2,2,2,2,2,2,2,4),(3.26034835787405E-5,
0.0529536178204587,0.105858380107734,0.141043201484947,0.23031053022423,
0.274574474417073,0.319027236436972,0.408667936702993,0.453280612706133,
0.497739098337324,0.542226872563317,0.630979078799732,0.675490307249623,
0.714880126578297),.UNSPECIFIED.);
#2103=B_SPLINE_CURVE_WITH_KNOTS('',3,(#12952,#12953,#12954,#12955,#12956,
#12957,#12958,#12959,#12960,#12961,#12962,#12963,#12964,#12965,#12966,#12967,
#12968,#12969,#12970,#12971,#12972,#12973,#12974,#12975,#12976,#12977,#12978,
#12979,#12980,#12981,#12982,#12983,#12984,#12985,#12986,#12987,#12988,#12989,
#12990,#12991,#12992,#12993,#12994,#12995,#12996,#12997,#12998,#12999,#13000,
#13001,#13002,#13003),.UNSPECIFIED.,.F.,.F.,(4,2,2,2,2,2,2,2,2,2,2,2,2,
2,2,2,2,2,2,2,2,2,2,2,2,4),(1.00000006295758E-6,0.0529473084571401,0.105845005097466,
0.141024979753782,0.230292688622603,0.274556378984213,0.319009143379118,
0.408650170385479,0.453262931403543,0.497721148223992,0.542208775050986,
0.630962893371619,0.675474208251199,0.720112502998726,0.809313740248424,
0.853615587847759,0.898067083267914,0.987627259379836,1.03222159080723,
1.07672147192959,1.12123281554438,1.20960590707816,1.25409915637214,1.29876974423772,
1.38788560124205,1.42992065923686),.UNSPECIFIED.);
#2104=B_SPLINE_CURVE_WITH_KNOTS('',3,(#13004,#13005,#13006,#13007,#13008,
#13009,#13010,#13011,#13012,#13013,#13014,#13015,#13016,#13017,#13018,#13019,
#13020,#13021,#13022,#13023,#13024,#13025,#13026,#13027,#13028,#13029,#13030,
#13031,#13032,#13033,#13034,#13035,#13036,#13037,#13038,#13039,#13040,#13041,
#13042,#13043,#13044,#13045,#13046,#13047,#13048,#13049,#13050,#13051,#13052,
#13053,#13054,#13055,#13056,#13057),.UNSPECIFIED.,.F.,.F.,(4,2,2,2,2,2,
2,2,2,2,2,2,2,2,2,2,2,2,2,2,2,2,2,2,2,2,4),(0.714880126578297,0.720128821383708,
0.809329599837282,0.853631763893768,0.898083290245698,0.987642791510278,
1.03223701035026,1.0767372055681,1.12124875484821,1.20961880657035,1.25411195148966,
1.29878277901107,1.38789807957833,1.43225266331332,1.47670998136068,1.56610905963984,
1.61067942473116,1.65522975133509,1.69977666599439,1.78750721371321,1.87524094334269,
1.91979362512494,1.96433764910848,2.0089101364871,2.09832216229164,2.14278443501037,
2.14503879498624),.UNSPECIFIED.);
#2105=B_SPLINE_CURVE_WITH_KNOTS('',3,(#13060,#13061,#13062,#13063,#13064,
#13065),.UNSPECIFIED.,.F.,.F.,(4,2,4),(-0.0939490999539409,-0.0470050902016758,
-1.84510844862747E-5),.UNSPECIFIED.);
#2106=B_SPLINE_CURVE_WITH_KNOTS('',3,(#13067,#13068,#13069,#13070,#13071,
#13072),.UNSPECIFIED.,.F.,.F.,(4,2,4),(-0.0245511647397311,-0.012301164739731,
-4.98173261989365E-5),.UNSPECIFIED.);
#2107=B_SPLINE_CURVE_WITH_KNOTS('',3,(#13074,#13075,#13076,#13077,#13078,
#13079),.UNSPECIFIED.,.F.,.F.,(4,2,4),(-0.024549949138571,-0.0123012966393727,
-5.12966393727537E-5),.UNSPECIFIED.);
#2108=B_SPLINE_CURVE_WITH_KNOTS('',3,(#13080,#13081,#13082,#13083,#13084,
#13085),.UNSPECIFIED.,.F.,.F.,(4,2,4),(-0.0940281721018956,-0.0470425165176012,
-9.75232268322135E-5),.UNSPECIFIED.);
#2109=B_SPLINE_CURVE_WITH_KNOTS('',3,(#13088,#13089,#13090,#13091,#13092,
#13093,#13094,#13095,#13096,#13097,#13098,#13099,#13100,#13101,#13102,#13103,
#13104,#13105,#13106,#13107,#13108,#13109,#13110,#13111,#13112,#13113,#13114,
#13115,#13116,#13117,#13118,#13119,#13120,#13121,#13122,#13123,#13124,#13125,
#13126,#13127,#13128,#13129,#13130,#13131,#13132,#13133,#13134,#13135,#13136,
#13137,#13138,#13139),.UNSPECIFIED.,.F.,.F.,(4,2,2,2,2,2,2,2,2,2,2,2,2,
2,2,2,2,2,2,2,2,2,2,2,2,4),(2.14503879498624,2.1871354385732,2.27623952298521,
2.32090428141422,2.36540151183267,2.45377524812087,2.49829287105407,2.54278766638035,
2.58738402328276,2.67696004328402,2.72141686796932,2.76571706839078,2.85490638840218,
2.89953944658785,2.9440551464135,3.03281632471489,3.07731073186083,3.12176502096226,
3.16638009635026,3.25604013423686,3.30049882637889,3.3447624293985,3.43401865064795,
3.46918523193177,3.52206672757312,3.5749963877086),.UNSPECIFIED.);
#2110=B_SPLINE_CURVE_WITH_KNOTS('',3,(#13285,#13286,#13287,#13288,#13289,
#13290,#13291,#13292,#13293,#13294,#13295,#13296,#13297,#13298,#13299,#13300,
#13301,#13302,#13303,#13304,#13305,#13306,#13307,#13308,#13309,#13310,#13311,
#13312,#13313,#13314,#13315,#13316,#13317,#13318,#13319,#13320,#13321,#13322,
#13323,#13324,#13325,#13326,#13327,#13328,#13329,#13330,#13331,#13332,#13333,
#13334,#13335,#13336,#13337,#13338,#13339,#13340,#13341,#13342,#13343,#13344,
#13345,#13346,#13347,#13348,#13349,#13350,#13351,#13352,#13353,#13354,#13355,
#13356,#13357,#13358,#13359,#13360,#13361,#13362,#13363,#13364,#13365,#13366,
#13367,#13368,#13369,#13370),.UNSPECIFIED.,.F.,.F.,(4,2,2,2,2,2,2,2,2,2,
2,2,2,2,2,2,2,2,2,2,2,2,2,2,2,2,2,2,2,2,2,2,2,2,2,2,2,2,2,2,2,2,4),(-3.85123506044155,
-3.78487541403508,-3.71861843740112,-3.63108565202321,-3.56307062788875,
-3.48955351073223,-3.39011116153264,-3.28756064765323,-3.21142501850155,
-3.13819263854922,-3.04447171553351,-2.91317755199343,-2.82034930299588,
-2.74581519796329,-2.6482372951938,-2.50362504362689,-2.40302458529268,
-2.32466081344229,-2.23654291442963,-2.1160510015302,-2.00788420853694,
-1.92564309108704,-1.84340197363715,-1.73523518064389,-1.61474326774443,
-1.52662536873178,-1.44826159688142,-1.34766113854725,-1.20304888698038,
-1.10547098421093,-1.03093687917837,-0.938108630180896,-0.806814466640977,
-0.713093543625373,-0.63986116367313,-0.563725534521538,-0.461175020642281,
-0.361732671442888,-0.288215554286479,-0.220200530152141,-0.132667744774381,
-0.0664107174211822,-5.07026194194161E-5),.UNSPECIFIED.);
#2111=B_SPLINE_CURVE_WITH_KNOTS('',3,(#13513,#13514,#13515,#13516,#13517,
#13518,#13519,#13520,#13521,#13522,#13523,#13524,#13525,#13526,#13527,#13528,
#13529,#13530,#13531,#13532,#13533,#13534,#13535,#13536,#13537,#13538,#13539,
#13540,#13541,#13542,#13543,#13544,#13545,#13546,#13547,#13548,#13549,#13550,
#13551,#13552,#13553,#13554,#13555,#13556,#13557,#13558,#13559,#13560,#13561,
#13562,#13563,#13564,#13565,#13566,#13567,#13568,#13569,#13570,#13571,#13572,
#13573,#13574,#13575,#13576,#13577,#13578,#13579,#13580,#13581,#13582,#13583,
#13584,#13585,#13586,#13587,#13588,#13589,#13590,#13591,#13592,#13593,#13594,
#13595,#13596,#13597,#13598),.UNSPECIFIED.,.F.,.F.,(4,2,2,2,2,2,2,2,2,2,
2,2,2,2,2,2,2,2,2,2,2,2,2,2,2,2,2,2,2,2,2,2,2,2,2,2,2,2,2,2,2,2,4),(-3.85123405850883,
-3.78487517864781,-3.71861815415721,-3.63108537256124,-3.56307035136544,
-3.48955323738529,-3.39011089248222,-3.28756038303362,-3.21142475717148,
-3.13819238038325,-3.04447146141686,-2.91317730354951,-2.82034905856273,
-2.74581495675049,-2.64823705819698,-2.50362481287822,-2.40302435889057,
-2.32466059042599,-2.23654269522057,-2.11605078752714,-2.00788399920737,
-1.9256428853108,-1.84340177141424,-1.73523498309445,-1.61474307540097,
-1.52662518019554,-1.44826141173097,-1.34766095774334,-1.2030487124246,
-1.10547081387111,-1.03093671205888,-0.938108467072148,-0.806814309204971,
-0.713093390238713,-0.639861013450582,-0.563725387588521,-0.461174878140013,
-0.361732533237043,-0.288215419256955,-0.220200398061198,-0.132667616465267,
-0.066410653998432,-5.0998807349829E-5),.UNSPECIFIED.);
#2112=B_SPLINE_CURVE_WITH_KNOTS('',3,(#13599,#13600,#13601,#13602,#13603,
#13604),.UNSPECIFIED.,.F.,.F.,(4,2,4),(-0.0940291329153355,-0.0470424937982037,
-9.84840459302137E-5),.UNSPECIFIED.);
#2113=B_SPLINE_CURVE_WITH_KNOTS('',3,(#13607,#13608,#13609,#13610,#13611,
#13612),.UNSPECIFIED.,.F.,.F.,(4,2,4),(-0.024552644052882,-0.0123012966393732,
-5.12966393733071E-5),.UNSPECIFIED.);
#2114=B_SPLINE_CURVE_WITH_KNOTS('',3,(#13614,#13615,#13616,#13617,#13618,
#13619),.UNSPECIFIED.,.F.,.F.,(4,2,4),(-0.0245511874584252,-0.0123011874584247,
-5.25349590649871E-5),.UNSPECIFIED.);
#2115=B_SPLINE_CURVE_WITH_KNOTS('',3,(#13620,#13621,#13622,#13623,#13624,
#13625),.UNSPECIFIED.,.F.,.F.,(4,2,4),(-0.0939527595126648,-0.0470077662219547,
-2.21106376590829E-5),.UNSPECIFIED.);
#2116=B_SPLINE_CURVE_WITH_KNOTS('',3,(#13767,#13768,#13769,#13770,#13771,
#13772,#13773,#13774,#13775,#13776,#13777,#13778,#13779,#13780,#13781,#13782,
#13783,#13784,#13785,#13786,#13787,#13788,#13789,#13790,#13791,#13792,#13793,
#13794,#13795,#13796,#13797,#13798,#13799,#13800,#13801,#13802,#13803,#13804,
#13805,#13806,#13807,#13808,#13809,#13810,#13811,#13812,#13813,#13814,#13815,
#13816,#13817,#13818,#13819,#13820,#13821,#13822,#13823,#13824,#13825,#13826,
#13827,#13828,#13829,#13830,#13831,#13832,#13833,#13834,#13835,#13836,#13837,
#13838,#13839,#13840,#13841,#13842,#13843,#13844,#13845,#13846,#13847,#13848,
#13849,#13850,#13851,#13852),.UNSPECIFIED.,.F.,.F.,(4,2,2,2,2,2,2,2,2,2,
2,2,2,2,2,2,2,2,2,2,2,2,2,2,2,2,2,2,2,2,2,2,2,2,2,2,2,2,2,2,2,2,4),(5.07026194164673E-5,
0.0664107174211822,0.13266774477438,0.220200530152142,0.288215554286479,
0.361732671442871,0.461175020642267,0.563725534521481,0.639861163673004,
0.713093543625183,0.806814466640702,0.938108630180502,1.03093687917782,
1.10547098421022,1.20304888697946,1.34766113854594,1.44826159687985,1.52662536873,
1.61474326774239,1.73523518064143,1.84340197363434,1.92564309108396,2.00788420853358,
2.11605100152649,2.23654291442556,2.32466081343793,2.40302458528804,2.5036250436219,
2.64823729518831,2.74581519795744,2.82034930298975,2.91317755198693,3.04447171552645,
3.13819263854176,3.21142501849377,3.28756064764512,3.39011116152411,3.48955351072329,
3.56307062787951,3.63108565201366,3.71861843739117,3.78487541402478,3.85123506043089),
 .UNSPECIFIED.);
#2117=B_SPLINE_CURVE_WITH_KNOTS('',3,(#13994,#13995,#13996,#13997,#13998,
#13999,#14000,#14001,#14002,#14003,#14004,#14005,#14006,#14007,#14008,#14009,
#14010,#14011,#14012,#14013,#14014,#14015,#14016,#14017,#14018,#14019,#14020,
#14021,#14022,#14023,#14024,#14025,#14026,#14027,#14028,#14029,#14030,#14031,
#14032,#14033,#14034,#14035,#14036,#14037,#14038,#14039,#14040,#14041,#14042,
#14043,#14044,#14045,#14046,#14047,#14048,#14049,#14050,#14051,#14052,#14053,
#14054,#14055,#14056,#14057,#14058,#14059,#14060,#14061,#14062,#14063,#14064,
#14065,#14066,#14067,#14068,#14069,#14070,#14071,#14072,#14073,#14074,#14075,
#14076,#14077,#14078,#14079),.UNSPECIFIED.,.F.,.F.,(4,2,2,2,2,2,2,2,2,2,
2,2,2,2,2,2,2,2,2,2,2,2,2,2,2,2,2,2,2,2,2,2,2,2,2,2,2,2,2,2,2,2,4),(5.09988073474043E-5,
0.0664106539984153,0.132667616465238,0.220200398061176,0.288215419256946,
0.361732533237061,0.461174878140088,0.563725387588608,0.639861013450696,
0.713093390238879,0.806814309205198,0.938108467072451,1.03093671205917,
1.10547081387137,1.20304871242481,1.34766095774345,1.448261411731,1.52662518019551,
1.61474307540084,1.73523498309413,1.84340177141377,1.92564288531024,2.0078839992067,
2.11605078752635,2.23654269521968,2.324660590425,2.40302435888947,2.50362481287698,
2.64823705819555,2.74581495674892,2.82034905856104,2.91317730354766,3.04447146141472,
3.13819238038091,3.21142475716898,3.28756038303095,3.39011089247928,3.48955323738204,
3.56307035136197,3.63108537255756,3.71861815415326,3.78487517864366,3.85123405850448),
 .UNSPECIFIED.);
#2118=B_SPLINE_CURVE_WITH_KNOTS('',3,(#14222,#14223,#14224,#14225,#14226,
#14227,#14228,#14229,#14230,#14231,#14232,#14233,#14234,#14235,#14236,#14237,
#14238,#14239,#14240,#14241,#14242,#14243,#14244,#14245,#14246,#14247,#14248,
#14249,#14250,#14251,#14252,#14253,#14254,#14255,#14256,#14257,#14258,#14259,
#14260,#14261,#14262,#14263,#14264,#14265,#14266,#14267,#14268,#14269,#14270,
#14271,#14272,#14273,#14274,#14275,#14276,#14277,#14278,#14279,#14280,#14281,
#14282,#14283,#14284,#14285,#14286,#14287,#14288,#14289,#14290,#14291,#14292,
#14293,#14294,#14295,#14296,#14297,#14298,#14299,#14300,#14301,#14302,#14303,
#14304,#14305,#14306,#14307,#14308,#14309,#14310,#14311,#14312,#14313,#14314,
#14315,#14316,#14317,#14318,#14319,#14320,#14321,#14322,#14323,#14324,#14325,
#14326,#14327,#14328,#14329,#14330,#14331,#14332,#14333,#14334,#14335,#14336,
#14337,#14338,#14339,#14340,#14341,#14342,#14343,#14344,#14345,#14346,#14347,
#14348,#14349,#14350,#14351,#14352,#14353,#14354,#14355,#14356,#14357,#14358,
#14359,#14360,#14361,#14362,#14363,#14364,#14365,#14366,#14367,#14368,#14369,
#14370,#14371,#14372,#14373,#14374,#14375,#14376,#14377,#14378,#14379,#14380,
#14381,#14382,#14383,#14384,#14385,#14386,#14387,#14388,#14389,#14390,#14391,
#14392,#14393,#14394,#14395,#14396,#14397,#14398,#14399,#14400,#14401,#14402,
#14403,#14404,#14405,#14406,#14407,#14408,#14409,#14410,#14411,#14412,#14413,
#14414,#14415,#14416,#14417,#14418,#14419,#14420,#14421,#14422,#14423,#14424,
#14425,#14426,#14427,#14428,#14429,#14430,#14431,#14432,#14433,#14434,#14435,
#14436,#14437,#14438,#14439,#14440,#14441,#14442,#14443,#14444,#14445,#14446,
#14447,#14448,#14449,#14450,#14451,#14452,#14453,#14454,#14455,#14456,#14457,
#14458,#14459,#14460,#14461,#14462,#14463,#14464,#14465,#14466,#14467,#14468,
#14469,#14470,#14471,#14472,#14473,#14474,#14475,#14476,#14477,#14478,#14479,
#14480,#14481,#14482,#14483,#14484,#14485,#14486,#14487,#14488,#14489,#14490,
#14491,#14492,#14493,#14494,#14495,#14496,#14497,#14498,#14499,#14500,#14501,
#14502,#14503,#14504,#14505,#14506,#14507,#14508,#14509,#14510,#14511,#14512,
#14513,#14514,#14515,#14516,#14517,#14518,#14519,#14520,#14521,#14522,#14523,
#14524,#14525,#14526,#14527,#14528,#14529,#14530,#14531,#14532,#14533,#14534,
#14535,#14536,#14537,#14538,#14539,#14540,#14541,#14542,#14543,#14544,#14545,
#14546,#14547,#14548,#14549,#14550,#14551,#14552,#14553,#14554,#14555,#14556,
#14557,#14558,#14559,#14560,#14561,#14562,#14563,#14564,#14565,#14566,#14567,
#14568,#14569,#14570,#14571,#14572,#14573,#14574,#14575,#14576,#14577,#14578,
#14579,#14580,#14581,#14582,#14583,#14584,#14585,#14586,#14587,#14588,#14589,
#14590,#14591,#14592,#14593,#14594,#14595,#14596,#14597,#14598,#14599,#14600,
#14601,#14602,#14603,#14604,#14605,#14606,#14607,#14608,#14609,#14610,#14611,
#14612,#14613,#14614,#14615,#14616,#14617,#14618,#14619,#14620,#14621,#14622,
#14623,#14624),.UNSPECIFIED.,.F.,.F.,(4,3,3,3,3,3,3,3,3,3,3,3,3,3,3,3,3,
3,3,3,3,3,3,3,3,3,3,3,3,3,3,3,3,3,3,3,3,3,3,3,3,3,3,3,3,3,3,3,3,3,3,3,3,
3,3,3,3,3,3,3,3,3,3,3,3,3,3,3,3,3,3,3,3,3,3,3,3,3,3,3,3,3,3,3,3,3,3,3,3,
3,3,3,3,3,3,3,3,3,3,3,3,3,3,3,3,3,3,3,3,3,3,3,3,3,3,3,3,3,3,3,3,3,3,3,3,
3,3,3,3,3,3,3,3,3,4),(0.,0.009615384615385,0.0125000395761689,0.01923076923077,
0.02884615384615,0.03846153846154,0.0449999664041082,0.04807692307692,0.05769230769231,
0.06730769230769,0.07692307692308,0.0775000049929539,0.08653846153846,0.09615384615385,
0.1057692307692,0.110000014413493,0.1153846153846,0.125,0.1346153846154,
0.1424999755863,0.1442307692308,0.1538461538462,0.1634615384615,0.1730769230769,
0.175000027234005,0.1826923076923,0.1923076923077,0.2019230769231,0.207499981369673,
0.2115384615385,0.2211538461538,0.2307692307692,0.239999997337637,0.2403846153846,
0.25,0.2596153846154,0.2692307692308,0.272500030849891,0.2788461538462,
0.2884615384615,0.2980769230769,0.304999966725719,0.3076923076923,0.3173076923077,
0.3269230769231,0.3365384615385,0.337500011015578,0.3461538461538,0.3557692307692,
0.3653846153846,0.370000004926624,0.375,0.3846153846154,0.3942307692308,
0.402499982129091,0.4038461538462,0.4134615384615,0.4230769230769,0.4326923076923,
0.435000031453539,0.4423076923077,0.4519230769231,0.4615384615385,0.467499974129879,
0.4711538461538,0.4807692307692,0.4903846153846,0.5,0.5096153846154,0.5192307692308,
0.5288461538462,0.532500025870121,0.5384615384615,0.5480769230769,0.5576923076923,
0.564999968546461,0.5673076923077,0.5769230769231,0.5865384615385,0.5961538461538,
0.597500017870908,0.6057692307692,0.6153846153846,0.625,0.629999995073376,
0.6346153846154,0.6442307692308,0.6538461538462,0.662499988984422,0.6634615384615,
0.6730769230769,0.6826923076923,0.6923076923077,0.695000033274281,0.7019230769231,
0.7115384615385,0.7211538461538,0.727499969150109,0.7307692307692,0.7403846153846,
0.75,0.7596153846154,0.760000002662363,0.7692307692308,0.7788461538462,
0.7884615384615,0.792500018630328,0.7980769230769,0.8076923076923,0.8173076923077,
0.824999972765995,0.8269230769231,0.8365384615385,0.8461538461538,0.8557692307692,
0.8575000244137,0.8653846153846,0.875,0.8846153846154,0.889999985586514,
0.8942307692308,0.9038461538462,0.9134615384615,0.922499995007029,0.9230769230769,
0.9326923076923,0.9423076923077,0.9519230769231,0.955000033595907,0.9615384615385,
0.9711538461538,0.9807692307692,0.987499960423811,0.9903846153846,1.),
 .UNSPECIFIED.);
#2119=B_SPLINE_CURVE_WITH_KNOTS('',3,(#14906,#14907,#14908,#14909,#14910,
#14911,#14912,#14913,#14914,#14915,#14916,#14917,#14918,#14919,#14920,#14921,
#14922,#14923,#14924,#14925,#14926,#14927,#14928,#14929,#14930,#14931,#14932,
#14933,#14934,#14935,#14936,#14937,#14938,#14939,#14940,#14941,#14942,#14943,
#14944,#14945,#14946,#14947,#14948,#14949,#14950,#14951,#14952,#14953,#14954,
#14955,#14956,#14957,#14958,#14959,#14960,#14961,#14962,#14963,#14964,#14965,
#14966,#14967,#14968,#14969,#14970,#14971,#14972,#14973,#14974,#14975,#14976,
#14977,#14978,#14979,#14980,#14981,#14982,#14983,#14984,#14985,#14986,#14987,
#14988,#14989,#14990,#14991,#14992,#14993,#14994,#14995,#14996,#14997,#14998,
#14999,#15000,#15001,#15002,#15003,#15004,#15005,#15006,#15007,#15008,#15009,
#15010,#15011,#15012,#15013,#15014,#15015,#15016,#15017,#15018,#15019,#15020,
#15021,#15022,#15023,#15024,#15025,#15026,#15027,#15028,#15029,#15030,#15031,
#15032,#15033,#15034,#15035,#15036,#15037,#15038,#15039,#15040,#15041,#15042,
#15043,#15044,#15045,#15046,#15047,#15048,#15049,#15050,#15051,#15052,#15053,
#15054,#15055,#15056,#15057,#15058,#15059,#15060,#15061,#15062,#15063,#15064,
#15065,#15066,#15067,#15068,#15069,#15070,#15071,#15072,#15073,#15074,#15075,
#15076,#15077,#15078,#15079,#15080,#15081,#15082,#15083,#15084,#15085,#15086,
#15087,#15088,#15089,#15090,#15091,#15092,#15093,#15094,#15095,#15096,#15097,
#15098,#15099,#15100,#15101,#15102,#15103,#15104,#15105,#15106,#15107,#15108,
#15109,#15110,#15111,#15112,#15113,#15114,#15115,#15116,#15117,#15118,#15119,
#15120,#15121,#15122,#15123,#15124,#15125,#15126,#15127,#15128,#15129,#15130,
#15131,#15132,#15133,#15134,#15135,#15136,#15137,#15138,#15139,#15140,#15141,
#15142,#15143,#15144,#15145,#15146,#15147,#15148,#15149,#15150,#15151,#15152,
#15153,#15154,#15155,#15156,#15157,#15158,#15159,#15160,#15161,#15162,#15163,
#15164,#15165,#15166,#15167,#15168,#15169,#15170,#15171,#15172,#15173,#15174,
#15175,#15176,#15177,#15178,#15179,#15180,#15181,#15182,#15183,#15184,#15185,
#15186,#15187,#15188,#15189,#15190,#15191,#15192,#15193,#15194,#15195,#15196,
#15197,#15198,#15199,#15200,#15201,#15202,#15203,#15204,#15205,#15206,#15207,
#15208,#15209,#15210,#15211,#15212,#15213,#15214,#15215,#15216,#15217,#15218,
#15219,#15220,#15221,#15222,#15223,#15224,#15225,#15226,#15227,#15228,#15229,
#15230,#15231,#15232,#15233,#15234,#15235,#15236,#15237,#15238,#15239,#15240,
#15241,#15242,#15243,#15244,#15245,#15246,#15247,#15248,#15249,#15250,#15251,
#15252,#15253,#15254,#15255,#15256,#15257,#15258,#15259,#15260,#15261,#15262,
#15263,#15264,#15265,#15266,#15267,#15268,#15269,#15270,#15271,#15272,#15273,
#15274,#15275,#15276,#15277,#15278,#15279,#15280,#15281,#15282,#15283,#15284,
#15285,#15286,#15287,#15288,#15289,#15290,#15291,#15292,#15293,#15294,#15295,
#15296,#15297,#15298,#15299,#15300,#15301,#15302,#15303,#15304,#15305,#15306,
#15307,#15308),.UNSPECIFIED.,.F.,.F.,(4,3,3,3,3,3,3,3,3,3,3,3,3,3,3,3,3,
3,3,3,3,3,3,3,3,3,3,3,3,3,3,3,3,3,3,3,3,3,3,3,3,3,3,3,3,3,3,3,3,3,3,3,3,
3,3,3,3,3,3,3,3,3,3,3,3,3,3,3,3,3,3,3,3,3,3,3,3,3,3,3,3,3,3,3,3,3,3,3,3,
3,3,3,3,3,3,3,3,3,3,3,3,3,3,3,3,3,3,3,3,3,3,3,3,3,3,3,3,3,3,3,3,3,3,3,3,
3,3,3,3,3,3,3,3,3,4),(0.,0.009615384615385,0.0125000395761689,0.01923076923077,
0.02884615384615,0.03846153846154,0.0449999664041082,0.04807692307692,0.05769230769231,
0.06730769230769,0.07692307692308,0.0775000049929539,0.08653846153846,0.09615384615385,
0.1057692307692,0.110000014413493,0.1153846153846,0.125,0.1346153846154,
0.1424999755863,0.1442307692308,0.1538461538462,0.1634615384615,0.1730769230769,
0.175000027234005,0.1826923076923,0.1923076923077,0.2019230769231,0.207499981369672,
0.2115384615385,0.2211538461538,0.2307692307692,0.239999997337637,0.2403846153846,
0.25,0.2596153846154,0.2692307692308,0.272500030849891,0.2788461538462,
0.2884615384615,0.2980769230769,0.304999966725719,0.3076923076923,0.3173076923077,
0.3269230769231,0.3365384615385,0.337500011015578,0.3461538461538,0.3557692307692,
0.3653846153846,0.370000004926624,0.375,0.3846153846154,0.3942307692308,
0.402499982129091,0.4038461538462,0.4134615384615,0.4230769230769,0.4326923076923,
0.435000031453539,0.4423076923077,0.4519230769231,0.4615384615385,0.467499974129879,
0.4711538461538,0.4807692307692,0.4903846153846,0.5,0.5096153846154,0.5192307692308,
0.5288461538462,0.532500025870121,0.5384615384615,0.5480769230769,0.5576923076923,
0.564999968546461,0.5673076923077,0.5769230769231,0.5865384615385,0.5961538461538,
0.597500017870908,0.6057692307692,0.6153846153846,0.625,0.629999995073376,
0.6346153846154,0.6442307692308,0.6538461538462,0.662499988984422,0.6634615384615,
0.6730769230769,0.6826923076923,0.6923076923077,0.695000033274281,0.7019230769231,
0.7115384615385,0.7211538461538,0.727499969150109,0.7307692307692,0.7403846153846,
0.75,0.7596153846154,0.760000002662363,0.7692307692308,0.7788461538462,
0.7884615384615,0.792500018630328,0.7980769230769,0.8076923076923,0.8173076923077,
0.824999972765995,0.8269230769231,0.8365384615385,0.8461538461538,0.8557692307692,
0.8575000244137,0.8653846153846,0.875,0.8846153846154,0.889999985586515,
0.8942307692308,0.9038461538462,0.9134615384615,0.922499995007029,0.9230769230769,
0.9326923076923,0.9423076923077,0.9519230769231,0.955000033595907,0.9615384615385,
0.9711538461538,0.9807692307692,0.987499960423811,0.9903846153846,1.),
 .UNSPECIFIED.);
#2120=B_SPLINE_CURVE_WITH_KNOTS('',3,(#15456,#15457,#15458,#15459,#15460,
#15461,#15462,#15463,#15464,#15465,#15466,#15467,#15468,#15469),
 .UNSPECIFIED.,.F.,.F.,(4,2,2,2,2,2,4),(0.,0.0355906395315414,0.0702494491909799,
0.11384356616058,0.162348717043925,0.207260502710314,0.250804429192007),
 .UNSPECIFIED.);
#2121=B_SPLINE_CURVE_WITH_KNOTS('',3,(#15470,#15471,#15472,#15473),
 .UNSPECIFIED.,.F.,.F.,(4,4),(-0.00591028098960205,0.),.UNSPECIFIED.);
#2122=B_SPLINE_CURVE_WITH_KNOTS('',3,(#15476,#15477,#15478,#15479,#15480,
#15481,#15482,#15483,#15484,#15485,#15486,#15487,#15488,#15489,#15490,#15491,
#15492,#15493,#15494,#15495,#15496,#15497,#15498,#15499,#15500,#15501,#15502,
#15503,#15504,#15505,#15506,#15507,#15508,#15509,#15510,#15511,#15512,#15513,
#15514,#15515),.UNSPECIFIED.,.F.,.F.,(4,2,2,2,2,2,2,2,2,2,2,2,2,2,2,2,2,
2,2,4),(2.29225165853828E-5,0.0305122189456786,0.0532101150017384,0.0754571497564381,
0.104584917568519,0.142377147502123,0.162368429143501,0.191693310195574,
0.235517239689987,0.256050511622218,0.273508318076584,0.309278902134493,
0.335525645153663,0.379178507747342,0.40831102858237,0.429059497093713,
0.466876471116825,0.496068764353867,0.519112614876548,0.546227663897249),
 .UNSPECIFIED.);
#2123=B_SPLINE_CURVE_WITH_KNOTS('',3,(#15519,#15520,#15521,#15522,#15523,
#15524),.UNSPECIFIED.,.F.,.F.,(4,2,4),(-0.02824401145014,-0.0141111268813085,
-3.50485731018317E-5),.UNSPECIFIED.);
#2124=B_SPLINE_CURVE_WITH_KNOTS('',3,(#15526,#15527,#15528,#15529,#15530,
#15531),.UNSPECIFIED.,.F.,.F.,(4,2,4),(-0.0168790919016364,-0.00846513155472639,
-5.37848794413334E-5),.UNSPECIFIED.);
#2125=B_SPLINE_CURVE_WITH_KNOTS('',3,(#15532,#15533,#15534,#15535,#15536,
#15537),.UNSPECIFIED.,.F.,.F.,(4,2,4),(-0.000680132893780016,-0.00038988449192367,
-8.31318019695661E-6),.UNSPECIFIED.);
#2126=B_SPLINE_CURVE_WITH_KNOTS('',3,(#15679,#15680,#15681,#15682,#15683,
#15684,#15685,#15686,#15687,#15688,#15689,#15690,#15691,#15692,#15693,#15694,
#15695,#15696,#15697,#15698,#15699,#15700,#15701,#15702,#15703,#15704,#15705,
#15706,#15707,#15708,#15709,#15710,#15711,#15712,#15713,#15714,#15715,#15716,
#15717,#15718,#15719,#15720,#15721,#15722,#15723,#15724,#15725,#15726,#15727,
#15728,#15729,#15730,#15731,#15732,#15733,#15734,#15735,#15736,#15737,#15738,
#15739,#15740,#15741,#15742,#15743,#15744,#15745,#15746,#15747,#15748,#15749,
#15750,#15751,#15752,#15753,#15754,#15755,#15756,#15757,#15758,#15759,#15760,
#15761,#15762,#15763,#15764,#15765,#15766,#15767,#15768,#15769,#15770,#15771,
#15772,#15773,#15774,#15775,#15776,#15777,#15778,#15779,#15780,#15781,#15782,
#15783,#15784,#15785,#15786,#15787,#15788),.UNSPECIFIED.,.F.,.F.,(4,2,2,
2,2,2,2,2,2,2,2,2,2,2,2,2,2,2,2,2,2,2,2,2,2,2,2,2,2,2,2,2,2,2,2,2,2,2,2,
2,2,2,2,2,2,2,2,2,2,2,2,2,2,2,4),(-2.00382109951475,-1.97201129963151,-1.94433184367343,
-1.91464419504192,-1.88574115922005,-1.8514353042413,-1.81215756543003,
-1.76810090312334,-1.73023771802479,-1.69702662693861,-1.66354234713588,
-1.63101628430078,-1.59227967169984,-1.54786154099023,-1.50076256763616,
-1.46248270955476,-1.42893305519558,-1.39502934556627,-1.36214098153558,
-1.32284042358914,-1.27770158583834,-1.22982980708018,-1.19078386840074,
-1.1565906087955,-1.12196725706052,-1.08841938389405,-1.04820281978587,
-1.00193682403998,-0.955670828294093,-0.915454264185968,-0.881906391019558,
-0.847283039284548,-0.813089779679285,-0.774043840999812,-0.726172062241663,
-0.681033224490963,-0.641732666544431,-0.608844302513661,-0.574940592884397,
-0.541390938525295,-0.503111080443882,-0.456012107089795,-0.411593976380191,
-0.372857363779306,-0.340331300944244,-0.306847021141525,-0.27363593005535,
-0.235772744956746,-0.191716082650139,-0.152438343839065,-0.118132488860489,
-0.0892294530387735,-0.0595418044073706,-0.0318622560493046,-5.2727048378802E-5),
 .UNSPECIFIED.);
#2127=B_SPLINE_CURVE_WITH_KNOTS('',3,(#15791,#15792,#15793,#15794,#15795,
#15796,#15797,#15798,#15799,#15800,#15801,#15802,#15803,#15804,#15805,#15806,
#15807,#15808,#15809,#15810,#15811,#15812,#15813,#15814,#15815,#15816,#15817,
#15818,#15819,#15820,#15821,#15822,#15823,#15824,#15825,#15826,#15827,#15828,
#15829,#15830,#15831,#15832,#15833,#15834,#15835,#15836,#15837,#15838,#15839,
#15840,#15841,#15842,#15843,#15844,#15845,#15846,#15847,#15848,#15849,#15850,
#15851,#15852,#15853,#15854,#15855,#15856,#15857,#15858,#15859,#15860,#15861,
#15862,#15863,#15864,#15865,#15866,#15867,#15868,#15869,#15870,#15871,#15872,
#15873,#15874,#15875,#15876,#15877,#15878,#15879,#15880,#15881,#15882,#15883,
#15884,#15885,#15886,#15887,#15888,#15889,#15890,#15891,#15892,#15893,#15894,
#15895,#15896,#15897,#15898,#15899,#15900,#15901,#15902,#15903,#15904,#15905,
#15906,#15907,#15908,#15909,#15910,#15911,#15912,#15913,#15914,#15915,#15916,
#15917,#15918,#15919,#15920),.UNSPECIFIED.,.F.,.F.,(4,2,2,2,2,2,2,2,2,2,
2,2,2,2,2,2,2,2,2,2,2,2,2,2,2,2,2,2,2,2,2,2,2,2,2,2,2,2,2,2,2,2,2,2,2,2,
2,2,2,2,2,2,2,2,2,2,2,2,2,2,2,2,2,2,4),(-1.83625218848691,-1.80296123674716,
-1.77086825671766,-1.74211560059189,-1.71132774506505,-1.68640831841803,
-1.65714693616734,-1.62573150567781,-1.6008288419873,-1.57169238758313,
-1.54043408083162,-1.51554173836869,-1.48641103644225,-1.45515341445188,
-1.43027181930539,-1.40114891263515,-1.36990016990591,-1.34502960035837,
-1.31592204656361,-1.28468995316566,-1.25983025562054,-1.23073475026148,
-1.19951547514314,-1.17466668644213,-1.1455840541214,-1.11437869335724,
-1.08954080030501,-1.06047089597884,-1.02928577264449,-1.00445860133142,
-0.975398493160497,-0.943872179557161,-0.919064909412312,-0.894330101305452,
-0.861223437174857,-0.831260641947789,-0.806445883428347,-0.776752862964708,
-0.74718293112293,-0.722378895769069,-0.69153771031895,-0.661875784697552,
-0.637052233202022,-0.606408673955306,-0.576747969275706,-0.551910624025682,
-0.521194048999722,-0.491511324641091,-0.46665874037071,-0.435933945603862,
-0.406231981669284,-0.381364362589519,-0.350625227764694,-0.320911832012579,
-0.296029475423969,-0.265274334711648,-0.235538639512187,-0.210641308945321,
-0.179751853223789,-0.149928219526715,-0.125011810480556,-0.0947418078748108,
-0.0653387434889213,-0.0333024489493881,-2.53469989805008E-5),
 .UNSPECIFIED.);
#2128=B_SPLINE_CURVE_WITH_KNOTS('',3,(#16062,#16063,#16064,#16065,#16066,
#16067,#16068,#16069,#16070,#16071,#16072,#16073,#16074,#16075,#16076,#16077,
#16078,#16079,#16080,#16081,#16082,#16083,#16084,#16085,#16086,#16087,#16088,
#16089,#16090,#16091,#16092,#16093,#16094,#16095,#16096,#16097,#16098,#16099,
#16100,#16101,#16102,#16103,#16104,#16105,#16106,#16107,#16108,#16109,#16110,
#16111,#16112,#16113,#16114,#16115),.UNSPECIFIED.,.F.,.F.,(4,2,2,2,2,2,
2,2,2,2,2,2,2,2,2,2,2,2,2,2,2,2,2,2,2,2,4),(-0.750965113696085,-0.730368370240615,
-0.71363612769438,-0.694601232270837,-0.678242635614603,-0.66697556480159,
-0.637553682137494,-0.598436505921655,-0.565880747199001,-0.537592228302624,
-0.513432405865943,-0.480425777050235,-0.453424707065712,-0.437641522032812,
-0.41506346284529,-0.392734840588027,-0.340675533275673,-0.299351930108356,
-0.266313368147915,-0.237984909868301,-0.204824868419376,-0.16592819889631,
-0.137532920243293,-0.104590291383952,-0.0681247457833163,-0.0142696103655463,
-3.42971879727152E-5),.UNSPECIFIED.);
#2129=B_SPLINE_CURVE_WITH_KNOTS('',3,(#16118,#16119,#16120,#16121,#16122,
#16123,#16124,#16125,#16126,#16127,#16128,#16129,#16130,#16131,#16132,#16133,
#16134,#16135,#16136,#16137,#16138,#16139,#16140,#16141,#16142,#16143,#16144,
#16145,#16146,#16147,#16148,#16149,#16150,#16151,#16152,#16153,#16154,#16155,
#16156,#16157,#16158,#16159,#16160,#16161,#16162,#16163,#16164,#16165,#16166,
#16167,#16168,#16169,#16170,#16171,#16172,#16173,#16174,#16175,#16176,#16177,
#16178,#16179,#16180,#16181,#16182,#16183,#16184,#16185,#16186,#16187,#16188,
#16189,#16190,#16191,#16192,#16193,#16194,#16195,#16196,#16197,#16198,#16199,
#16200,#16201,#16202,#16203,#16204,#16205,#16206,#16207,#16208,#16209,#16210,
#16211,#16212,#16213,#16214,#16215,#16216,#16217,#16218,#16219,#16220,#16221,
#16222,#16223,#16224,#16225,#16226,#16227),.UNSPECIFIED.,.F.,.F.,(4,2,2,
2,2,2,2,2,2,2,2,2,2,2,2,2,2,2,2,2,2,2,2,2,2,2,2,2,2,2,2,2,2,2,2,2,2,2,2,
2,2,2,2,2,2,2,2,2,2,2,2,2,2,2,4),(5.22888875136238E-5,0.0318621331467355,
0.0595415760152274,0.0892292343844242,0.118132279686624,0.152438145917861,
0.191715897612406,0.235772574369891,0.273635771887746,0.306846873867313,
0.34033116465303,0.372857238156833,0.411593863463561,0.456012008742521,
0.503110997545273,0.541390868182636,0.574940533546252,0.608844254296138,
0.641732629114365,0.681033199951567,0.726172052508122,0.774043846968444,
0.813089798455132,0.847283069275912,0.881906432367515,0.915454316537837,
0.955670893837234,1.00193690475858,1.04820291567993,1.08841949297927,1.12196737714953,
1.15659074024116,1.19078401106196,1.22982996254868,1.27770175700899,1.32284060956542,
1.36214118040271,1.39502955522101,1.42893327597085,1.46248294133439,1.50076281197177,
1.54786180077453,1.59227994605348,1.63101657136015,1.6635426448639,1.69702693564962,
1.73023803762918,1.76810123514708,1.81215791190446,1.8514356635988,1.88574152982984,
1.91464457513187,1.94433223350095,1.97201179093797,2.00382132191843),
 .UNSPECIFIED.);
#2130=B_SPLINE_CURVE_WITH_KNOTS('',3,(#16510,#16511,#16512,#16513,#16514,
#16515,#16516,#16517,#16518,#16519,#16520,#16521,#16522,#16523,#16524,#16525,
#16526,#16527,#16528,#16529,#16530,#16531,#16532,#16533,#16534,#16535,#16536,
#16537,#16538,#16539,#16540,#16541,#16542,#16543,#16544,#16545,#16546,#16547,
#16548,#16549,#16550,#16551,#16552,#16553,#16554,#16555,#16556,#16557,#16558,
#16559,#16560,#16561,#16562,#16563,#16564,#16565,#16566,#16567,#16568,#16569,
#16570,#16571,#16572,#16573,#16574,#16575,#16576,#16577,#16578,#16579,#16580,
#16581,#16582,#16583,#16584,#16585,#16586,#16587,#16588,#16589,#16590,#16591,
#16592,#16593,#16594,#16595,#16596,#16597,#16598,#16599,#16600,#16601,#16602,
#16603,#16604,#16605,#16606,#16607,#16608,#16609,#16610,#16611,#16612,#16613,
#16614,#16615,#16616,#16617,#16618,#16619),.UNSPECIFIED.,.F.,.F.,(4,2,2,
2,2,2,2,2,2,2,2,2,2,2,2,2,2,2,2,2,2,2,2,2,2,2,2,2,2,2,2,2,2,2,2,2,2,2,2,
2,2,2,2,2,2,2,2,2,2,2,2,2,2,2,4),(5.27270482666441E-5,0.0318622560492564,
0.0595418044072771,0.0892294530387053,0.118132488860395,0.152438343838929,
0.191716082650089,0.235772744956499,0.273635930054719,0.306847021140621,
0.340331300943069,0.37285736377788,0.411593976378467,0.456012107087719,
0.503111080441407,0.541390938522476,0.574940592881332,0.608844302510329,
0.641732666540797,0.68103322448698,0.726172062237338,0.774043840995097,
0.813089779674242,0.847283039279203,0.881906391013914,0.91545426418006,
0.955670828287863,1.0019368240334,1.04820281977893,1.08841938388673,1.12196725705288,
1.15659060878759,1.19078386839256,1.22982980707169,1.27770158582945,1.32284042357981,
1.36214098152599,1.39502934555647,1.42893305518547,1.46248270954433,1.50076256762539,
1.54786154097908,1.59227967168835,1.63101628428893,1.66354234712375,1.6970266269262,
1.73023771801211,1.76810090311033,1.81215756541673,1.85143530422787,1.88574115920639,
1.91464419502807,1.94433184365948,1.97201139201748,2.00382091256426),
 .UNSPECIFIED.);
#2131=B_SPLINE_CURVE_WITH_KNOTS('',3,(#16622,#16623,#16624,#16625,#16626,
#16627,#16628,#16629,#16630,#16631,#16632,#16633,#16634,#16635,#16636,#16637,
#16638,#16639,#16640,#16641,#16642,#16643,#16644,#16645,#16646,#16647,#16648,
#16649,#16650,#16651,#16652,#16653,#16654,#16655,#16656,#16657,#16658,#16659,
#16660,#16661,#16662,#16663,#16664,#16665,#16666,#16667,#16668,#16669,#16670,
#16671,#16672,#16673,#16674,#16675,#16676,#16677,#16678,#16679,#16680,#16681,
#16682,#16683,#16684,#16685,#16686,#16687,#16688,#16689,#16690,#16691,#16692,
#16693,#16694,#16695,#16696,#16697,#16698,#16699,#16700,#16701,#16702,#16703,
#16704,#16705,#16706,#16707,#16708,#16709,#16710,#16711,#16712,#16713,#16714,
#16715,#16716,#16717,#16718,#16719,#16720,#16721,#16722,#16723,#16724,#16725,
#16726,#16727,#16728,#16729,#16730,#16731),.UNSPECIFIED.,.F.,.F.,(4,2,2,
2,2,2,2,2,2,2,2,2,2,2,2,2,2,2,2,2,2,2,2,2,2,2,2,2,2,2,2,2,2,2,2,2,2,2,2,
2,2,2,2,2,2,2,2,2,2,2,2,2,2,2,4),(-2.00382091256489,-1.97201139201814,-1.94433184366008,
-1.91464419502864,-1.88574115920694,-1.85143530422839,-1.81215756541722,
-1.76810090311079,-1.73023771801257,-1.69702662692665,-1.6635423471242,
-1.63101628428938,-1.59227967168878,-1.54786154097952,-1.50076256762582,
-1.46248270954475,-1.42893305518588,-1.39502934555687,-1.3621409815264,
-1.3228404235802,-1.27770158582984,-1.22982980707207,-1.19078386839291,
-1.15659060878794,-1.12196725705323,-1.08841938388707,-1.04820281977926,
-1.00193682403371,-0.955670828288167,-0.915454264180356,-0.8819063910142,
-0.847283039279479,-0.813089779674504,-0.774043840995357,-0.726172062237589,
-0.681033224487208,-0.641732666541015,-0.608844302510536,-0.574940592881528,
-0.541390938522659,-0.503111080441583,-0.456012107087879,-0.4115939763786,
-0.372857363778004,-0.340331300943183,-0.306847021140722,-0.273635930054805,
-0.235772744956571,-0.191716082650154,-0.152438343838999,-0.11813248886047,
-0.0892294530387833,-0.0595418044073568,-0.0318622560492987,-5.27270483708445E-5),
 .UNSPECIFIED.);
#2132=B_SPLINE_CURVE_WITH_KNOTS('',3,(#16873,#16874,#16875,#16876,#16877,
#16878,#16879,#16880,#16881,#16882,#16883,#16884,#16885,#16886,#16887,#16888,
#16889,#16890,#16891,#16892,#16893,#16894,#16895,#16896,#16897,#16898,#16899,
#16900,#16901,#16902,#16903,#16904,#16905,#16906,#16907,#16908,#16909,#16910,
#16911,#16912,#16913,#16914,#16915,#16916,#16917,#16918,#16919,#16920,#16921,
#16922,#16923,#16924,#16925,#16926,#16927,#16928,#16929,#16930,#16931,#16932,
#16933,#16934,#16935,#16936,#16937,#16938,#16939,#16940,#16941,#16942,#16943,
#16944,#16945,#16946,#16947,#16948,#16949,#16950,#16951,#16952,#16953,#16954,
#16955,#16956,#16957,#16958,#16959,#16960,#16961,#16962,#16963,#16964,#16965,
#16966,#16967,#16968,#16969,#16970,#16971,#16972,#16973,#16974,#16975,#16976,
#16977,#16978,#16979,#16980,#16981,#16982,#16983,#16984,#16985,#16986,#16987,
#16988,#16989,#16990,#16991,#16992,#16993,#16994,#16995,#16996,#16997,#16998,
#16999,#17000,#17001,#17002),.UNSPECIFIED.,.F.,.F.,(4,2,2,2,2,2,2,2,2,2,
2,2,2,2,2,2,2,2,2,2,2,2,2,2,2,2,2,2,2,2,2,2,2,2,2,2,2,2,2,2,2,2,2,2,2,2,
2,2,2,2,2,2,2,2,2,2,2,2,2,2,2,2,2,2,4),(-1.83561951873259,-1.80235844975814,
-1.77029427716558,-1.74156743012038,-1.71080721051427,-1.68591015214814,
-1.65667503562308,-1.62528780438682,-1.60040749393025,-1.57129719311318,
-1.54006694457515,-1.51519694608158,-1.48609239257846,-1.45486282824274,
-1.43000356741716,-1.40090680214813,-1.36968611497522,-1.34483786969891,
-1.31575644088785,-1.28455297753445,-1.25971557915402,-1.23064592334211,
-1.19949870357013,-1.17467106965797,-1.1455947194486,-1.11507291396498,
-1.09023936697185,-1.06088794575343,-1.02660547905822,-1.00186644644199,
-0.973997323135063,-0.948862180594986,-0.920459596649707,-0.895744960446151,
-0.860670082843373,-0.830239044945616,-0.805393512545119,-0.776808789940427,
-0.747243163128625,-0.722439176252239,-0.691584141646649,-0.66192066238225,
-0.637096800111612,-0.606456628004131,-0.576795951846665,-0.551958393276278,
-0.521240644871582,-0.491557566857789,-0.466704745602487,-0.435979884286414,
-0.406277661599022,-0.381409811250468,-0.35067033454635,-0.320956656424519,
-0.296074066980763,-0.26531865226729,-0.235582680284637,-0.210685117079743,
-0.179795369294768,-0.149971456539647,-0.125054814588245,-0.0947845298923839,
-0.0653811907334665,-0.0333252066690533,-6.53684496053783E-5),
 .UNSPECIFIED.);
#2133=B_SPLINE_CURVE_WITH_KNOTS('',3,(#17145,#17146,#17147,#17148,#17149,
#17150,#17151,#17152,#17153,#17154,#17155,#17156,#17157,#17158,#17159,#17160,
#17161,#17162,#17163,#17164,#17165,#17166,#17167,#17168,#17169,#17170,#17171,
#17172,#17173,#17174,#17175,#17176,#17177,#17178,#17179,#17180,#17181,#17182,
#17183,#17184,#17185,#17186,#17187,#17188,#17189,#17190,#17191,#17192,#17193,
#17194,#17195,#17196,#17197,#17198,#17199,#17200),.UNSPECIFIED.,.F.,.F.,
(4,2,2,2,2,2,2,2,2,2,2,2,2,2,2,2,2,2,2,2,2,2,2,2,2,2,2,4),(-1.0462023949558,
-1.02770916434491,-0.963207867413976,-0.91312002222191,-0.88354318731338,
-0.842015496578868,-0.791686095343267,-0.76026436767404,-0.719495385836737,
-0.668995568553684,-0.638516311726255,-0.597094721113933,-0.54650375020668,
-0.514711112380782,-0.47382163868678,-0.432772015023298,-0.402277229521919,
-0.371443744672249,-0.323513899110614,-0.258717091288244,-0.237510669203495,
-0.206526557725729,-0.166517534835296,-0.138197809313294,-0.104591110020813,
-0.0681236581910849,-0.0142648413735641,-3.42971879826158E-5),
 .UNSPECIFIED.);
#2134=B_SPLINE_CURVE_WITH_KNOTS('',3,(#17343,#17344,#17345,#17346,#17347,
#17348,#17349,#17350,#17351,#17352,#17353,#17354,#17355,#17356,#17357,#17358,
#17359,#17360,#17361,#17362,#17363,#17364,#17365,#17366,#17367,#17368,#17369,
#17370,#17371,#17372,#17373,#17374,#17375,#17376,#17377,#17378,#17379,#17380,
#17381,#17382,#17383,#17384,#17385,#17386,#17387,#17388,#17389,#17390,#17391,
#17392,#17393,#17394,#17395,#17396,#17397,#17398,#17399,#17400,#17401,#17402,
#17403,#17404,#17405,#17406,#17407,#17408,#17409,#17410,#17411,#17412,#17413,
#17414,#17415,#17416,#17417,#17418,#17419,#17420,#17421,#17422,#17423,#17424,
#17425,#17426,#17427,#17428,#17429,#17430,#17431,#17432,#17433,#17434,#17435,
#17436,#17437,#17438,#17439,#17440,#17441,#17442,#17443,#17444,#17445,#17446,
#17447,#17448,#17449,#17450,#17451,#17452,#17453,#17454),.UNSPECIFIED.,
 .F.,.F.,(4,2,2,2,2,2,2,2,2,2,2,2,2,2,2,2,2,2,2,2,2,2,2,2,2,2,2,2,2,2,2,
2,2,2,2,2,2,2,2,2,2,2,2,2,2,2,2,2,2,2,2,2,2,2,2,4),(-1.74231738659323,-1.71272813854196,
-1.68417838271532,-1.65861170299748,-1.63123533686212,-1.60907714051855,
-1.58305810475277,-1.55512370293588,-1.53298041210706,-1.50707246139104,
-1.47927777300709,-1.45714365974848,-1.43124082409921,-1.40344674460942,
-1.38132218779627,-1.35542628363528,-1.32764010052686,-1.3055253475805,
-1.27964309465111,-1.2518718165722,-1.2297667283235,-1.20389514364682,-1.17614465541501,
-1.15404902253465,-1.12818466554023,-1.10070401616129,-1.07861121041395,
-1.05264017735879,-1.02306666941232,-1.0010322038119,-0.975921411019613,
-0.954332580969174,-0.932111573457994,-0.903636393356442,-0.883192092893937,
-0.838253102959002,-0.812582949517684,-0.781618122961311,-0.742546052526065,
-0.695158920459714,-0.657943517604473,-0.607098500578842,-0.569371545127974,
-0.518888680069456,-0.479979748859535,-0.43362258666965,-0.397223341127724,
-0.346657163261735,-0.310296328919488,-0.259971486866278,-0.223517021715003,
-0.173445822844544,-0.136570721100847,-0.086863575551722,-0.0496665678786331,
-6.53688914877267E-5),.UNSPECIFIED.);
#2135=B_SPLINE_CURVE_WITH_KNOTS('',3,(#17456,#17457,#17458,#17459,#17460,
#17461,#17462,#17463,#17464,#17465,#17466,#17467,#17468,#17469,#17470,#17471,
#17472,#17473,#17474,#17475,#17476,#17477,#17478,#17479,#17480,#17481,#17482,
#17483,#17484,#17485,#17486,#17487,#17488,#17489,#17490,#17491,#17492,#17493,
#17494,#17495,#17496,#17497,#17498,#17499,#17500,#17501,#17502,#17503,#17504,
#17505),.UNSPECIFIED.,.F.,.F.,(4,2,2,2,2,2,2,2,2,2,2,2,2,2,2,2,2,2,2,2,
2,2,2,2,4),(-1.15405318984419,-1.13700531982188,-1.07753998041418,-1.03134662925519,
-0.959427083652358,-0.903949051282896,-0.818092854923278,-0.752201951754484,
-0.710444097003286,-0.657297506880136,-0.591014894046436,-0.555925429665672,
-0.521099070865684,-0.46097016602311,-0.376614638147581,-0.324415207912168,
-0.262381146764866,-0.237997672332685,-0.203720015827636,-0.165639244416124,
-0.13727850827765,-0.104604576414893,-0.0681040508243425,-0.0141799990057525,
-3.4421973892809E-5),.UNSPECIFIED.);
#2136=B_SPLINE_CURVE_WITH_KNOTS('',3,(#17508,#17509,#17510,#17511,#17512,
#17513,#17514,#17515,#17516,#17517,#17518,#17519,#17520,#17521,#17522,#17523,
#17524,#17525,#17526,#17527,#17528,#17529,#17530,#17531,#17532,#17533,#17534,
#17535,#17536,#17537,#17538,#17539,#17540,#17541,#17542,#17543,#17544,#17545,
#17546,#17547,#17548,#17549,#17550,#17551,#17552,#17553,#17554,#17555,#17556,
#17557,#17558,#17559,#17560,#17561,#17562,#17563,#17564,#17565,#17566,#17567,
#17568,#17569,#17570,#17571,#17572,#17573,#17574,#17575,#17576,#17577,#17578,
#17579,#17580,#17581,#17582,#17583,#17584,#17585,#17586,#17587,#17588,#17589,
#17590,#17591,#17592,#17593,#17594,#17595,#17596,#17597,#17598,#17599,#17600,
#17601,#17602,#17603,#17604,#17605,#17606,#17607,#17608,#17609,#17610,#17611,
#17612,#17613,#17614,#17615,#17616,#17617),.UNSPECIFIED.,.F.,.F.,(4,2,2,
2,2,2,2,2,2,2,2,2,2,2,2,2,2,2,2,2,2,2,2,2,2,2,2,2,2,2,2,2,2,2,2,2,2,2,2,
2,2,2,2,2,2,2,2,2,2,2,2,2,2,2,4),(5.27270482716431E-5,0.0318622560492676,
0.0595418044073026,0.089229453038713,0.118132488860435,0.152438343839018,
0.191716082650095,0.235772744956718,0.273635930055335,0.306847021141509,
0.340331300944227,0.372857363779289,0.41159397638018,0.456012107089798,
0.503111080443886,0.541390938525302,0.574940592884411,0.608844302513673,
0.641732666544447,0.681033224490987,0.726172062241692,0.774043840999849,
0.813089779679324,0.847283039284585,0.881906391019603,0.915454264186023,
0.955670828294158,1.00193682404004,1.04820281978592,1.08841938389412,1.12196725706059,
1.15659060879558,1.19078386840081,1.22982980708026,1.27770158583843,1.32284042358924,
1.36214098153568,1.39502934556638,1.42893305519569,1.46248270955487,1.50076256763627,
1.54786154099035,1.59227967169997,1.63101628430091,1.66354234713601,1.69702662693874,
1.73023771802493,1.76810090312348,1.81215756543019,1.85143530424147,1.88574115922024,
1.91464419504213,1.94433184367366,1.97201140238705,2.00382079698849),
 .UNSPECIFIED.);
#2137=B_SPLINE_CURVE_WITH_KNOTS('',3,(#17759,#17760,#17761,#17762,#17763,
#17764,#17765,#17766,#17767,#17768,#17769,#17770,#17771,#17772,#17773,#17774,
#17775,#17776,#17777,#17778,#17779,#17780,#17781,#17782,#17783,#17784,#17785,
#17786,#17787,#17788,#17789,#17790,#17791,#17792,#17793,#17794,#17795,#17796,
#17797,#17798,#17799,#17800,#17801,#17802,#17803,#17804,#17805,#17806,#17807,
#17808,#17809,#17810,#17811,#17812,#17813,#17814,#17815,#17816,#17817,#17818,
#17819,#17820,#17821,#17822,#17823,#17824,#17825,#17826,#17827,#17828,#17829,
#17830,#17831,#17832,#17833,#17834,#17835,#17836,#17837,#17838,#17839,#17840,
#17841,#17842,#17843,#17844,#17845,#17846,#17847,#17848,#17849,#17850,#17851,
#17852,#17853,#17854,#17855,#17856,#17857,#17858,#17859,#17860,#17861,#17862,
#17863,#17864,#17865,#17866,#17867,#17868),.UNSPECIFIED.,.F.,.F.,(4,2,2,
2,2,2,2,2,2,2,2,2,2,2,2,2,2,2,2,2,2,2,2,2,2,2,2,2,2,2,2,2,2,2,2,2,2,2,2,
2,2,2,2,2,2,2,2,2,2,2,2,2,2,2,4),(-2.00382122385324,-1.97201169537238,-1.94433214011032,
-1.91464448407403,-1.88574144104314,-1.85143557750779,-1.81215782889982,
-1.76810115560431,-1.73023796106162,-1.69702686169173,-1.66354257353715,
-1.63101650258923,-1.59227988032641,-1.54786173853774,-1.50076275343594,
-1.46248288580652,-1.42893322307924,-1.3950295049935,-1.3621411327595,-1.32284056501037,
-1.27770171600086,-1.22982992530222,-1.19078397688366,-1.1565907087497,
-1.12196734837871,-1.08841946684456,-1.04820289270536,-1.00193688541952,
-0.955670878133678,-0.915454303994412,-0.881906422460213,-0.84728306208925,
-0.813089793955311,-0.774043845536778,-0.72617205483812,-0.681033205828492,
-0.641732638079455,-0.60884426584553,-0.57494054775973,-0.541390885032382,
-0.503111017402976,-0.456012032301171,-0.411593890512498,-0.372857268249625,
-0.340331197301665,-0.306846909147073,-0.273635809777168,-0.235772615234533,
-0.191715941938926,-0.152438193330733,-0.118132329795171,-0.0892292867641046,
-0.0595416307276913,-0.0318621625886586,-5.24944897148018E-5),
 .UNSPECIFIED.);
#2138=B_SPLINE_CURVE_WITH_KNOTS('',3,(#18011,#18012,#18013,#18014,#18015,
#18016,#18017,#18018,#18019,#18020,#18021,#18022,#18023,#18024,#18025,#18026,
#18027,#18028,#18029,#18030,#18031,#18032,#18033,#18034,#18035,#18036,#18037,
#18038,#18039,#18040,#18041,#18042,#18043,#18044,#18045,#18046,#18047,#18048,
#18049,#18050,#18051,#18052,#18053,#18054,#18055,#18056,#18057,#18058,#18059,
#18060,#18061,#18062,#18063,#18064,#18065,#18066,#18067,#18068,#18069,#18070,
#18071,#18072,#18073,#18074,#18075,#18076,#18077,#18078,#18079,#18080,#18081,
#18082,#18083,#18084,#18085,#18086,#18087,#18088,#18089,#18090,#18091,#18092,
#18093,#18094,#18095,#18096,#18097,#18098,#18099,#18100,#18101,#18102,#18103,
#18104,#18105,#18106,#18107,#18108,#18109,#18110,#18111,#18112,#18113,#18114,
#18115,#18116,#18117,#18118,#18119,#18120,#18121,#18122,#18123,#18124,#18125,
#18126,#18127,#18128,#18129,#18130,#18131,#18132,#18133,#18134,#18135,#18136,
#18137,#18138),.UNSPECIFIED.,.F.,.F.,(4,2,2,2,2,2,2,2,2,2,2,2,2,2,2,2,2,
2,2,2,2,2,2,2,2,2,2,2,2,2,2,2,2,2,2,2,2,2,2,2,2,2,2,2,2,2,2,2,2,2,2,2,2,
2,2,2,2,2,2,2,2,2,2,4),(-0.724209442048021,-0.712012419228065,-0.699774873077863,
-0.681616457852927,-0.657341985081789,-0.629929009821504,-0.605852526236518,
-0.588109932419774,-0.574000009703252,-0.567069686309773,-0.552823216848468,
-0.541467982710213,-0.532126067407773,-0.527510625181189,-0.518055019712594,
-0.508582461845211,-0.499343005773517,-0.494751846095525,-0.48537530451312,
-0.475940089247624,-0.46676365554951,-0.462178749472849,-0.452841775748094,
-0.443408651260855,-0.434256693627476,-0.429661699527251,-0.420326774943473,
-0.410864213717641,-0.40170027949673,-0.397080753977129,-0.392376911709479,
-0.383407884051634,-0.378959110293847,-0.36958100457871,-0.364962404238539,
-0.35576581741293,-0.346284065020516,-0.336915288463779,-0.332312667618732,
-0.32310011095919,-0.313621704271534,-0.304228734377309,-0.299627376680961,
-0.290366677380499,-0.280861125252255,-0.271412143331777,-0.266796755617985,
-0.257458230849559,-0.247894532506044,-0.238360581007524,-0.233717042817114,
-0.22427442650142,-0.212771689213361,-0.198340223892403,-0.19133056640038,
-0.177011525952808,-0.15915412450686,-0.135775818155052,-0.124447490718968,
-0.101217094808881,-0.0719670763949736,-0.0361476301246094,-0.0180607317449348,
-0.000136180809809842),.UNSPECIFIED.);
#2139=B_SPLINE_CURVE_WITH_KNOTS('',3,(#18140,#18141,#18142,#18143,#18144,
#18145),.UNSPECIFIED.,.F.,.F.,(4,2,4),(-0.00483247580106661,-0.00242691911098953,
-3.7601910332494E-5),.UNSPECIFIED.);
#2140=B_SPLINE_CURVE_WITH_KNOTS('',3,(#18147,#18148,#18149,#18150,#18151,
#18152),.UNSPECIFIED.,.F.,.F.,(4,2,4),(-0.0275281976707898,-0.0137825502036224,
0.),.UNSPECIFIED.);
#2141=B_SPLINE_CURVE_WITH_KNOTS('',3,(#18153,#18154,#18155,#18156,#18157,
#18158,#18159,#18160,#18161,#18162,#18163,#18164,#18165,#18166,#18167,#18168,
#18169,#18170,#18171,#18172,#18173,#18174,#18175,#18176,#18177,#18178,#18179,
#18180,#18181,#18182,#18183,#18184,#18185,#18186,#18187,#18188,#18189,#18190,
#18191,#18192,#18193,#18194,#18195,#18196,#18197,#18198,#18199,#18200,#18201,
#18202,#18203,#18204,#18205,#18206,#18207,#18208,#18209,#18210,#18211,#18212,
#18213,#18214,#18215,#18216,#18217,#18218,#18219,#18220,#18221,#18222,#18223,
#18224,#18225,#18226,#18227,#18228,#18229,#18230,#18231,#18232,#18233,#18234,
#18235,#18236,#18237,#18238,#18239,#18240,#18241,#18242,#18243,#18244,#18245,
#18246,#18247,#18248,#18249,#18250,#18251,#18252,#18253,#18254,#18255,#18256,
#18257,#18258,#18259,#18260),.UNSPECIFIED.,.F.,.F.,(4,2,2,2,2,2,2,2,2,2,
2,2,2,2,2,2,2,2,2,2,2,2,2,2,2,2,2,2,2,2,2,2,2,2,2,2,2,2,2,2,2,2,2,2,2,2,
2,2,2,2,2,2,2,4),(-1.57864048508544,-1.54446598849513,-1.51282058354209,
-1.45635482471215,-1.38848776585317,-1.34517905219782,-1.29525802411295,
-1.25847858725278,-1.1746608395351,-1.0883691385114,-1.04485089132505,-0.983145009409519,
-0.934695536189604,-0.909958056093548,-0.863794529076489,-0.815460471775503,
-0.772619307001527,-0.754454882157872,-0.734069641642063,-0.713058389711127,
-0.676589030490018,-0.661713978186576,-0.645311909159579,-0.625653759340365,
-0.609503546676276,-0.593095359946264,-0.573586468342252,-0.558552932808393,
-0.526799939615536,-0.511275497870786,-0.479962305397725,-0.455344123339125,
-0.435814495644388,-0.426321102519358,-0.411609772310643,-0.391569769342903,
-0.380083028459815,-0.358611529716761,-0.34905248340869,-0.337758942861699,
-0.327260348971232,-0.302583518122225,-0.286919863682097,-0.273277943945509,
-0.2599164773094,-0.240329742861226,-0.22649402828818,-0.212635850179124,
-0.185447274727583,-0.1507298160219,-0.125935120495647,-0.0766598253180761,
-0.0387520613078884,-5.9346581474212E-5),.UNSPECIFIED.);
#2142=B_SPLINE_CURVE_WITH_KNOTS('',3,(#18403,#18404,#18405,#18406,#18407,
#18408,#18409,#18410,#18411,#18412,#18413,#18414,#18415,#18416),
 .UNSPECIFIED.,.F.,.F.,(4,2,2,2,2,2,4),(-0.129888666319633,-0.110958901973454,
-0.0925929637960144,-0.0673725322659813,-0.0429943158352172,-0.0236944798609603,
-0.000230509019371229),.UNSPECIFIED.);
#2143=B_SPLINE_CURVE_WITH_KNOTS('',3,(#18417,#18418,#18419,#18420,#18421,
#18422,#18423,#18424,#18425,#18426,#18427,#18428,#18429,#18430,#18431,#18432,
#18433,#18434,#18435,#18436,#18437,#18438,#18439,#18440,#18441,#18442,#18443,
#18444,#18445,#18446,#18447,#18448,#18449,#18450,#18451,#18452,#18453,#18454,
#18455,#18456,#18457,#18458,#18459,#18460,#18461,#18462,#18463,#18464,#18465,
#18466,#18467,#18468,#18469,#18470,#18471,#18472,#18473,#18474,#18475,#18476,
#18477,#18478,#18479,#18480,#18481,#18482,#18483,#18484,#18485,#18486,#18487,
#18488,#18489,#18490,#18491,#18492,#18493,#18494,#18495,#18496,#18497,#18498,
#18499,#18500,#18501,#18502,#18503,#18504,#18505,#18506,#18507,#18508,#18509,
#18510,#18511,#18512,#18513,#18514,#18515,#18516,#18517,#18518,#18519,#18520,
#18521,#18522,#18523,#18524,#18525,#18526,#18527,#18528,#18529,#18530,#18531,
#18532,#18533,#18534,#18535,#18536,#18537,#18538,#18539,#18540,#18541,#18542,
#18543,#18544,#18545,#18546,#18547,#18548,#18549,#18550,#18551,#18552,#18553,
#18554,#18555,#18556,#18557,#18558,#18559,#18560),.UNSPECIFIED.,.F.,.F.,
(4,2,2,2,2,2,2,2,2,2,2,2,2,2,2,2,2,2,2,2,2,2,2,2,2,2,2,2,2,2,2,2,2,2,2,
2,2,2,2,2,2,2,2,2,2,2,2,2,2,2,2,2,2,2,2,2,2,2,2,2,2,2,2,2,2,2,2,2,2,2,2,
4),(5.26474022382527E-5,0.0318393369807604,0.0592980128182023,0.0792979431064048,
0.0957672433172796,0.118106620244403,0.138323222401668,0.159239151214813,
0.181746335419478,0.203560881592912,0.214840885573553,0.232910739511272,
0.244852133659171,0.266091583097692,0.28355229855556,0.302089976658252,
0.3294942454828,0.366122471577819,0.415668980781027,0.44123794526359,0.492927603854394,
0.517600256378281,0.568883400921198,0.605742580438842,0.635198909934618,
0.64697236331899,0.661501095163747,0.679780743311896,0.700525486353231,
0.711127765381697,0.725195329375971,0.73194061555702,0.737998800367963,
0.743454178372273,0.749017259543572,0.755225752700343,0.761418999200457,
0.77459256360018,0.795106074764413,0.815670757121667,0.826809833565304,
0.837650332183119,0.858417228122364,0.880166564725393,0.900193699045498,
0.909908247699591,0.919128297180291,0.928151730327303,0.935176718718845,
0.949204304985769,0.955159083922506,0.962270981377388,0.971310099577727,
0.9783604628954,0.985155774681686,0.992653618211583,1.0012163312926,1.01209394806449,
1.0197719145481,1.02746363271032,1.04274408783163,1.06201238916331,1.07561766958023,
1.09557471449015,1.11100247230759,1.11680896979578,1.12470779989893,1.13261955506168,
1.14211456831916,1.1509639127575,1.15980968395025,1.16911313657596),
 .UNSPECIFIED.);
#2144=B_SPLINE_CURVE_WITH_KNOTS('',3,(#18561,#18562,#18563,#18564,#18565,
#18566,#18567,#18568,#18569,#18570,#18571,#18572,#18573,#18574,#18575,#18576,
#18577,#18578),.UNSPECIFIED.,.F.,.F.,(4,2,2,2,2,2,2,2,4),(2.08074705752938E-5,
0.0299251342462279,0.0593388741588997,0.0818316849232177,0.12040051455881,
0.158340949255542,0.182369650545949,0.211471464162904,0.240621100987305),
 .UNSPECIFIED.);
#2145=B_SPLINE_CURVE_WITH_KNOTS('',3,(#18583,#18584,#18585,#18586,#18587,
#18588,#18589,#18590,#18591,#18592,#18593,#18594,#18595,#18596,#18597,#18598,
#18599,#18600,#18601,#18602,#18603,#18604,#18605,#18606,#18607,#18608,#18609,
#18610,#18611,#18612,#18613,#18614,#18615,#18616,#18617,#18618,#18619,#18620,
#18621,#18622,#18623,#18624,#18625,#18626,#18627,#18628,#18629,#18630,#18631,
#18632,#18633,#18634,#18635,#18636,#18637,#18638,#18639,#18640,#18641,#18642,
#18643,#18644,#18645,#18646,#18647,#18648,#18649,#18650,#18651,#18652,#18653,
#18654,#18655,#18656,#18657,#18658,#18659,#18660,#18661,#18662,#18663,#18664,
#18665,#18666,#18667,#18668,#18669,#18670,#18671,#18672,#18673,#18674,#18675,
#18676,#18677,#18678,#18679),.UNSPECIFIED.,.F.,.F.,(4,3,3,3,3,3,3,3,3,3,
3,3,3,3,3,3,3,3,3,3,3,3,3,3,3,3,3,3,3,3,3,3,4),(0.,0.0258201387254787,0.0629152472513321,
0.0875674000511779,0.113912785737008,0.153702165597873,0.188336926200019,
0.224722540734876,0.260495064077292,0.28070605024531,0.322581006932306,
0.358158673070872,0.383171365469391,0.419466953457704,0.445774356425421,
0.469641907940648,0.520771786653062,0.545004609088268,0.57335363416754,
0.607202336040835,0.630053107004349,0.649602042372964,0.691474446019008,
0.724334403640295,0.779068317023684,0.809490011109605,0.830155841963515,
0.866649489803741,0.891096251784872,0.910952203144824,0.944692325772077,
0.978832779385412,0.999625753900943),.UNSPECIFIED.);
#2146=B_SPLINE_CURVE_WITH_KNOTS('',3,(#18680,#18681,#18682,#18683),
 .UNSPECIFIED.,.F.,.F.,(4,4),(0.,0.000550666282709742),.UNSPECIFIED.);
#2462=LINE('',#12550,#2927);
#2463=LINE('',#12605,#2928);
#2464=LINE('',#12607,#2929);
#2465=LINE('',#12611,#2930);
#2466=LINE('',#12721,#2931);
#2467=LINE('',#12836,#2932);
#2468=LINE('',#12951,#2933);
#2469=LINE('',#13141,#2934);
#2470=LINE('',#13143,#2935);
#2471=LINE('',#13371,#2936);
#2472=LINE('',#13853,#2937);
#2473=LINE('',#14221,#2938);
#2474=LINE('',#14765,#2939);
#2475=LINE('',#15454,#2940);
#2476=LINE('',#15516,#2941);
#2477=LINE('',#15790,#2942);
#2478=LINE('',#16117,#2943);
#2479=LINE('',#16368,#2944);
#2480=LINE('',#16621,#2945);
#2481=LINE('',#17003,#2946);
#2482=LINE('',#17201,#2947);
#2483=LINE('',#17507,#2948);
#2484=LINE('',#17869,#2949);
#2485=LINE('',#18581,#2950);
#2486=LINE('',#18686,#2951);
#2487=LINE('',#18828,#2952);
#2488=LINE('',#18977,#2953);
#2927=VECTOR('',#10216,2.25);
#2928=VECTOR('',#10217,2.25);
#2929=VECTOR('',#10220,1.176);
#2930=VECTOR('',#10223,2.25);
#2931=VECTOR('',#10226,2.25);
#2932=VECTOR('',#10229,2.25);
#2933=VECTOR('',#10232,2.25);
#2934=VECTOR('',#10237,2.25);
#2935=VECTOR('',#10240,1.176);
#2936=VECTOR('',#10241,0.939826579747624);
#2937=VECTOR('',#10244,0.939826579747624);
#2938=VECTOR('',#10245,0.245);
#2939=VECTOR('',#10246,0.245);
#2940=VECTOR('',#10251,0.2381569860407);
#2941=VECTOR('',#10254,0.3125);
#2942=VECTOR('',#10257,0.281746931364498);
#2943=VECTOR('',#10258,0.281746931364498);
#2944=VECTOR('',#10259,0.1682530686355);
#2945=VECTOR('',#10260,0.1682530686355);
#2946=VECTOR('',#10261,0.281746931364498);
#2947=VECTOR('',#10262,0.281746931364498);
#2948=VECTOR('',#10263,0.281746931364491);
#2949=VECTOR('',#10264,0.281746931364491);
#2950=VECTOR('',#10267,0.238156986040692);
#2951=VECTOR('',#10272,0.1375);
#2952=VECTOR('',#10275,0.1682530686355);
#2953=VECTOR('',#10286,3.5);
#3392=VERTEX_POINT('',#12548);
#3393=VERTEX_POINT('',#12549);
#3394=VERTEX_POINT('',#12551);
#3395=VERTEX_POINT('',#12604);
#3396=VERTEX_POINT('',#12609);
#3397=VERTEX_POINT('',#12610);
#3398=VERTEX_POINT('',#12719);
#3399=VERTEX_POINT('',#12720);
#3400=VERTEX_POINT('',#12722);
#3401=VERTEX_POINT('',#12834);
#3402=VERTEX_POINT('',#12835);
#3403=VERTEX_POINT('',#12891);
#3404=VERTEX_POINT('',#12949);
#3405=VERTEX_POINT('',#12950);
#3406=VERTEX_POINT('',#13059);
#3407=VERTEX_POINT('',#13066);
#3408=VERTEX_POINT('',#13073);
#3409=VERTEX_POINT('',#13087);
#3410=VERTEX_POINT('',#13140);
#3411=VERTEX_POINT('',#13284);
#3412=VERTEX_POINT('',#13512);
#3413=VERTEX_POINT('',#13606);
#3414=VERTEX_POINT('',#13613);
#3415=VERTEX_POINT('',#13766);
#3416=VERTEX_POINT('',#14220);
#3417=VERTEX_POINT('',#15450);
#3418=VERTEX_POINT('',#15451);
#3419=VERTEX_POINT('',#15453);
#3420=VERTEX_POINT('',#15455);
#3421=VERTEX_POINT('',#15475);
#3422=VERTEX_POINT('',#15518);
#3423=VERTEX_POINT('',#15525);
#3424=VERTEX_POINT('',#15678);
#3425=VERTEX_POINT('',#15789);
#3426=VERTEX_POINT('',#16061);
#3427=VERTEX_POINT('',#16116);
#3428=VERTEX_POINT('',#16509);
#3429=VERTEX_POINT('',#16620);
#3430=VERTEX_POINT('',#16872);
#3431=VERTEX_POINT('',#17144);
#3432=VERTEX_POINT('',#17342);
#3433=VERTEX_POINT('',#17455);
#3434=VERTEX_POINT('',#17506);
#3435=VERTEX_POINT('',#17758);
#3436=VERTEX_POINT('',#18010);
#3437=VERTEX_POINT('',#18139);
#3438=VERTEX_POINT('',#18146);
#3439=VERTEX_POINT('',#18401);
#3440=VERTEX_POINT('',#18402);
#3441=VERTEX_POINT('',#18580);
#3442=VERTEX_POINT('',#18582);
#3443=VERTEX_POINT('',#18970);
#3444=VERTEX_POINT('',#18973);
#3445=VERTEX_POINT('',#18974);
#3446=VERTEX_POINT('',#18979);
#4256=EDGE_CURVE('',#3392,#3393,#2462,.T.);
#4257=EDGE_CURVE('',#3392,#3394,#2094,.T.);
#4258=EDGE_CURVE('',#3394,#3395,#2463,.T.);
#4259=EDGE_CURVE('',#3395,#3395,#1627,.T.);
#4260=EDGE_CURVE('',#3394,#3393,#2464,.T.);
#4261=EDGE_CURVE('',#3396,#3397,#2465,.T.);
#4262=EDGE_CURVE('',#3396,#3392,#2095,.T.);
#4263=EDGE_CURVE('',#3393,#3397,#2096,.T.);
#4264=EDGE_CURVE('',#3398,#3399,#2466,.T.);
#4265=EDGE_CURVE('',#3398,#3400,#2097,.T.);
#4266=EDGE_CURVE('',#3400,#3396,#2098,.T.);
#4267=EDGE_CURVE('',#3397,#3399,#2099,.T.);
#4268=EDGE_CURVE('',#3401,#3402,#2467,.T.);
#4269=EDGE_CURVE('',#3401,#3398,#2100,.T.);
#4270=EDGE_CURVE('',#3399,#3403,#2101,.T.);
#4271=EDGE_CURVE('',#3403,#3402,#2102,.T.);
#4272=EDGE_CURVE('',#3404,#3405,#2468,.T.);
#4273=EDGE_CURVE('',#3404,#3401,#2103,.T.);
#4274=EDGE_CURVE('',#3402,#3405,#2104,.T.);
#4275=EDGE_CURVE('',#3406,#3394,#2105,.T.);
#4276=EDGE_CURVE('',#3407,#3406,#2106,.T.);
#4277=EDGE_CURVE('',#3408,#3407,#2107,.T.);
#4278=EDGE_CURVE('',#3393,#3408,#2108,.T.);
#4279=EDGE_CURVE('',#3405,#3409,#2109,.T.);
#4280=EDGE_CURVE('',#3410,#3409,#2469,.T.);
#4281=EDGE_CURVE('',#3410,#3410,#1628,.T.);
#4282=EDGE_CURVE('',#3404,#3409,#2470,.T.);
#4283=EDGE_CURVE('',#3408,#3411,#2110,.T.);
#4284=EDGE_CURVE('',#3403,#3411,#2471,.T.);
#4285=EDGE_CURVE('',#3411,#3412,#2111,.T.);
#4286=EDGE_CURVE('',#3409,#3412,#2112,.T.);
#4287=EDGE_CURVE('',#3412,#3413,#2113,.T.);
#4288=EDGE_CURVE('',#3413,#3414,#2114,.T.);
#4289=EDGE_CURVE('',#3414,#3404,#2115,.T.);
#4290=EDGE_CURVE('',#3415,#3414,#2116,.T.);
#4291=EDGE_CURVE('',#3415,#3400,#2472,.T.);
#4292=EDGE_CURVE('',#3406,#3415,#2117,.T.);
#4293=EDGE_CURVE('',#3416,#3415,#2473,.T.);
#4294=EDGE_CURVE('',#3407,#3416,#2118,.T.);
#4295=EDGE_CURVE('',#3411,#3416,#2474,.T.);
#4296=EDGE_CURVE('',#3416,#3413,#2119,.T.);
#4297=EDGE_CURVE('',#3417,#3418,#1629,.T.);
#4298=EDGE_CURVE('',#3418,#3419,#2475,.T.);
#4299=EDGE_CURVE('',#3420,#3419,#2120,.T.);
#4300=EDGE_CURVE('',#3420,#3417,#2121,.T.);
#4301=EDGE_CURVE('',#3421,#3417,#2122,.T.);
#4302=EDGE_CURVE('',#3418,#3421,#2476,.T.);
#4303=EDGE_CURVE('',#3422,#3421,#2123,.T.);
#4304=EDGE_CURVE('',#3423,#3422,#2124,.T.);
#4305=EDGE_CURVE('',#3419,#3423,#2125,.T.);
#4306=EDGE_CURVE('',#3423,#3424,#2126,.T.);
#4307=EDGE_CURVE('',#3425,#3424,#2477,.T.);
#4308=EDGE_CURVE('',#3421,#3425,#2127,.F.);
#4309=EDGE_CURVE('',#3425,#3426,#2128,.T.);
#4310=EDGE_CURVE('',#3427,#3426,#2478,.T.);
#4311=EDGE_CURVE('',#3422,#3427,#2129,.T.);
#4312=EDGE_CURVE('',#3424,#3427,#2479,.T.);
#4313=EDGE_CURVE('',#3427,#3428,#2130,.T.);
#4314=EDGE_CURVE('',#3429,#3428,#2480,.T.);
#4315=EDGE_CURVE('',#3424,#3429,#2131,.T.);
#4316=EDGE_CURVE('',#3426,#3430,#2132,.F.);
#4317=EDGE_CURVE('',#3430,#3429,#2481,.T.);
#4318=EDGE_CURVE('',#3430,#3431,#2133,.T.);
#4319=EDGE_CURVE('',#3428,#3431,#2482,.T.);
#4320=EDGE_CURVE('',#3431,#3432,#2134,.T.);
#4321=EDGE_CURVE('',#3432,#3433,#2135,.T.);
#4322=EDGE_CURVE('',#3434,#3433,#2483,.T.);
#4323=EDGE_CURVE('',#3428,#3434,#2136,.T.);
#4324=EDGE_CURVE('',#3429,#3435,#2137,.T.);
#4325=EDGE_CURVE('',#3432,#3435,#2484,.T.);
#4326=EDGE_CURVE('',#3435,#3436,#2138,.T.);
#4327=EDGE_CURVE('',#3436,#3437,#2139,.T.);
#4328=EDGE_CURVE('',#3438,#3437,#2140,.T.);
#4329=EDGE_CURVE('',#3433,#3438,#2141,.F.);
#4330=EDGE_CURVE('',#3439,#3440,#2142,.T.);
#4331=EDGE_CURVE('',#3434,#3440,#2143,.T.);
#4332=EDGE_CURVE('',#3438,#3439,#2144,.T.);
#4333=EDGE_CURVE('',#3441,#3437,#2485,.T.);
#4334=EDGE_CURVE('',#3442,#3436,#2145,.T.);
#4335=EDGE_CURVE('',#3440,#3442,#2146,.T.);
#4336=EDGE_CURVE('',#3439,#3441,#1630,.T.);
#4337=EDGE_CURVE('',#3441,#3438,#2486,.T.);
#4338=EDGE_CURVE('',#3435,#3434,#2487,.T.);
#4339=EDGE_CURVE('',#3443,#3443,#1631,.T.);
#4340=EDGE_CURVE('',#3444,#3445,#1632,.T.);
#4341=EDGE_CURVE('',#3445,#3444,#1633,.T.);
#4342=EDGE_CURVE('',#3445,#3443,#2488,.T.);
#4343=EDGE_CURVE('',#3446,#3444,#1634,.T.);
#5620=ORIENTED_EDGE('',*,*,#4256,.F.);
#5621=ORIENTED_EDGE('',*,*,#4257,.T.);
#5622=ORIENTED_EDGE('',*,*,#4258,.T.);
#5623=ORIENTED_EDGE('',*,*,#4259,.T.);
#5624=ORIENTED_EDGE('',*,*,#4258,.F.);
#5625=ORIENTED_EDGE('',*,*,#4260,.T.);
#5626=ORIENTED_EDGE('',*,*,#4261,.F.);
#5627=ORIENTED_EDGE('',*,*,#4262,.T.);
#5628=ORIENTED_EDGE('',*,*,#4256,.T.);
#5629=ORIENTED_EDGE('',*,*,#4263,.T.);
#5630=ORIENTED_EDGE('',*,*,#4264,.F.);
#5631=ORIENTED_EDGE('',*,*,#4265,.T.);
#5632=ORIENTED_EDGE('',*,*,#4266,.T.);
#5633=ORIENTED_EDGE('',*,*,#4261,.T.);
#5634=ORIENTED_EDGE('',*,*,#4267,.T.);
#5635=ORIENTED_EDGE('',*,*,#4268,.F.);
#5636=ORIENTED_EDGE('',*,*,#4269,.T.);
#5637=ORIENTED_EDGE('',*,*,#4264,.T.);
#5638=ORIENTED_EDGE('',*,*,#4270,.T.);
#5639=ORIENTED_EDGE('',*,*,#4271,.T.);
#5640=ORIENTED_EDGE('',*,*,#4272,.F.);
#5641=ORIENTED_EDGE('',*,*,#4273,.T.);
#5642=ORIENTED_EDGE('',*,*,#4268,.T.);
#5643=ORIENTED_EDGE('',*,*,#4274,.T.);
#5644=ORIENTED_EDGE('',*,*,#4260,.F.);
#5645=ORIENTED_EDGE('',*,*,#4275,.F.);
#5646=ORIENTED_EDGE('',*,*,#4276,.F.);
#5647=ORIENTED_EDGE('',*,*,#4277,.F.);
#5648=ORIENTED_EDGE('',*,*,#4278,.F.);
#5649=ORIENTED_EDGE('',*,*,#4272,.T.);
#5650=ORIENTED_EDGE('',*,*,#4279,.T.);
#5651=ORIENTED_EDGE('',*,*,#4280,.F.);
#5652=ORIENTED_EDGE('',*,*,#4281,.F.);
#5653=ORIENTED_EDGE('',*,*,#4280,.T.);
#5654=ORIENTED_EDGE('',*,*,#4282,.F.);
#5655=ORIENTED_EDGE('',*,*,#4263,.F.);
#5656=ORIENTED_EDGE('',*,*,#4278,.T.);
#5657=ORIENTED_EDGE('',*,*,#4283,.T.);
#5658=ORIENTED_EDGE('',*,*,#4284,.F.);
#5659=ORIENTED_EDGE('',*,*,#4270,.F.);
#5660=ORIENTED_EDGE('',*,*,#4267,.F.);
#5661=ORIENTED_EDGE('',*,*,#4271,.F.);
#5662=ORIENTED_EDGE('',*,*,#4284,.T.);
#5663=ORIENTED_EDGE('',*,*,#4285,.T.);
#5664=ORIENTED_EDGE('',*,*,#4286,.F.);
#5665=ORIENTED_EDGE('',*,*,#4279,.F.);
#5666=ORIENTED_EDGE('',*,*,#4274,.F.);
#5667=ORIENTED_EDGE('',*,*,#4282,.T.);
#5668=ORIENTED_EDGE('',*,*,#4286,.T.);
#5669=ORIENTED_EDGE('',*,*,#4287,.T.);
#5670=ORIENTED_EDGE('',*,*,#4288,.T.);
#5671=ORIENTED_EDGE('',*,*,#4289,.T.);
#5672=ORIENTED_EDGE('',*,*,#4273,.F.);
#5673=ORIENTED_EDGE('',*,*,#4289,.F.);
#5674=ORIENTED_EDGE('',*,*,#4290,.F.);
#5675=ORIENTED_EDGE('',*,*,#4291,.T.);
#5676=ORIENTED_EDGE('',*,*,#4265,.F.);
#5677=ORIENTED_EDGE('',*,*,#4269,.F.);
#5678=ORIENTED_EDGE('',*,*,#4266,.F.);
#5679=ORIENTED_EDGE('',*,*,#4291,.F.);
#5680=ORIENTED_EDGE('',*,*,#4292,.F.);
#5681=ORIENTED_EDGE('',*,*,#4275,.T.);
#5682=ORIENTED_EDGE('',*,*,#4257,.F.);
#5683=ORIENTED_EDGE('',*,*,#4262,.F.);
#5684=ORIENTED_EDGE('',*,*,#4276,.T.);
#5685=ORIENTED_EDGE('',*,*,#4292,.T.);
#5686=ORIENTED_EDGE('',*,*,#4293,.F.);
#5687=ORIENTED_EDGE('',*,*,#4294,.F.);
#5688=ORIENTED_EDGE('',*,*,#4277,.T.);
#5689=ORIENTED_EDGE('',*,*,#4294,.T.);
#5690=ORIENTED_EDGE('',*,*,#4295,.F.);
#5691=ORIENTED_EDGE('',*,*,#4283,.F.);
#5692=ORIENTED_EDGE('',*,*,#4295,.T.);
#5693=ORIENTED_EDGE('',*,*,#4296,.T.);
#5694=ORIENTED_EDGE('',*,*,#4287,.F.);
#5695=ORIENTED_EDGE('',*,*,#4285,.F.);
#5696=ORIENTED_EDGE('',*,*,#4293,.T.);
#5697=ORIENTED_EDGE('',*,*,#4290,.T.);
#5698=ORIENTED_EDGE('',*,*,#4288,.F.);
#5699=ORIENTED_EDGE('',*,*,#4296,.F.);
#5700=ORIENTED_EDGE('',*,*,#4281,.T.);
#5701=ORIENTED_EDGE('',*,*,#4297,.T.);
#5702=ORIENTED_EDGE('',*,*,#4298,.T.);
#5703=ORIENTED_EDGE('',*,*,#4299,.F.);
#5704=ORIENTED_EDGE('',*,*,#4300,.T.);
#5705=ORIENTED_EDGE('',*,*,#4297,.F.);
#5706=ORIENTED_EDGE('',*,*,#4301,.F.);
#5707=ORIENTED_EDGE('',*,*,#4302,.F.);
#5708=ORIENTED_EDGE('',*,*,#4298,.F.);
#5709=ORIENTED_EDGE('',*,*,#4302,.T.);
#5710=ORIENTED_EDGE('',*,*,#4303,.F.);
#5711=ORIENTED_EDGE('',*,*,#4304,.F.);
#5712=ORIENTED_EDGE('',*,*,#4305,.F.);
#5713=ORIENTED_EDGE('',*,*,#4299,.T.);
#5714=ORIENTED_EDGE('',*,*,#4305,.T.);
#5715=ORIENTED_EDGE('',*,*,#4306,.T.);
#5716=ORIENTED_EDGE('',*,*,#4307,.F.);
#5717=ORIENTED_EDGE('',*,*,#4308,.F.);
#5718=ORIENTED_EDGE('',*,*,#4301,.T.);
#5719=ORIENTED_EDGE('',*,*,#4300,.F.);
#5720=ORIENTED_EDGE('',*,*,#4308,.T.);
#5721=ORIENTED_EDGE('',*,*,#4309,.T.);
#5722=ORIENTED_EDGE('',*,*,#4310,.F.);
#5723=ORIENTED_EDGE('',*,*,#4311,.F.);
#5724=ORIENTED_EDGE('',*,*,#4303,.T.);
#5725=ORIENTED_EDGE('',*,*,#4304,.T.);
#5726=ORIENTED_EDGE('',*,*,#4311,.T.);
#5727=ORIENTED_EDGE('',*,*,#4312,.F.);
#5728=ORIENTED_EDGE('',*,*,#4306,.F.);
#5729=ORIENTED_EDGE('',*,*,#4312,.T.);
#5730=ORIENTED_EDGE('',*,*,#4313,.T.);
#5731=ORIENTED_EDGE('',*,*,#4314,.F.);
#5732=ORIENTED_EDGE('',*,*,#4315,.F.);
#5733=ORIENTED_EDGE('',*,*,#4316,.F.);
#5734=ORIENTED_EDGE('',*,*,#4309,.F.);
#5735=ORIENTED_EDGE('',*,*,#4307,.T.);
#5736=ORIENTED_EDGE('',*,*,#4315,.T.);
#5737=ORIENTED_EDGE('',*,*,#4317,.F.);
#5738=ORIENTED_EDGE('',*,*,#4316,.T.);
#5739=ORIENTED_EDGE('',*,*,#4318,.T.);
#5740=ORIENTED_EDGE('',*,*,#4319,.F.);
#5741=ORIENTED_EDGE('',*,*,#4313,.F.);
#5742=ORIENTED_EDGE('',*,*,#4310,.T.);
#5743=ORIENTED_EDGE('',*,*,#4320,.T.);
#5744=ORIENTED_EDGE('',*,*,#4321,.T.);
#5745=ORIENTED_EDGE('',*,*,#4322,.F.);
#5746=ORIENTED_EDGE('',*,*,#4323,.F.);
#5747=ORIENTED_EDGE('',*,*,#4319,.T.);
#5748=ORIENTED_EDGE('',*,*,#4320,.F.);
#5749=ORIENTED_EDGE('',*,*,#4318,.F.);
#5750=ORIENTED_EDGE('',*,*,#4317,.T.);
#5751=ORIENTED_EDGE('',*,*,#4324,.T.);
#5752=ORIENTED_EDGE('',*,*,#4325,.F.);
#5753=ORIENTED_EDGE('',*,*,#4321,.F.);
#5754=ORIENTED_EDGE('',*,*,#4325,.T.);
#5755=ORIENTED_EDGE('',*,*,#4326,.T.);
#5756=ORIENTED_EDGE('',*,*,#4327,.T.);
#5757=ORIENTED_EDGE('',*,*,#4328,.F.);
#5758=ORIENTED_EDGE('',*,*,#4329,.F.);
#5759=ORIENTED_EDGE('',*,*,#4330,.T.);
#5760=ORIENTED_EDGE('',*,*,#4331,.F.);
#5761=ORIENTED_EDGE('',*,*,#4322,.T.);
#5762=ORIENTED_EDGE('',*,*,#4329,.T.);
#5763=ORIENTED_EDGE('',*,*,#4332,.T.);
#5764=ORIENTED_EDGE('',*,*,#4333,.T.);
#5765=ORIENTED_EDGE('',*,*,#4327,.F.);
#5766=ORIENTED_EDGE('',*,*,#4334,.F.);
#5767=ORIENTED_EDGE('',*,*,#4335,.F.);
#5768=ORIENTED_EDGE('',*,*,#4330,.F.);
#5769=ORIENTED_EDGE('',*,*,#4336,.T.);
#5770=ORIENTED_EDGE('',*,*,#4333,.F.);
#5771=ORIENTED_EDGE('',*,*,#4337,.T.);
#5772=ORIENTED_EDGE('',*,*,#4328,.T.);
#5773=ORIENTED_EDGE('',*,*,#4332,.F.);
#5774=ORIENTED_EDGE('',*,*,#4337,.F.);
#5775=ORIENTED_EDGE('',*,*,#4336,.F.);
#5776=ORIENTED_EDGE('',*,*,#4334,.T.);
#5777=ORIENTED_EDGE('',*,*,#4326,.F.);
#5778=ORIENTED_EDGE('',*,*,#4338,.T.);
#5779=ORIENTED_EDGE('',*,*,#4331,.T.);
#5780=ORIENTED_EDGE('',*,*,#4335,.T.);
#5781=ORIENTED_EDGE('',*,*,#4314,.T.);
#5782=ORIENTED_EDGE('',*,*,#4323,.T.);
#5783=ORIENTED_EDGE('',*,*,#4338,.F.);
#5784=ORIENTED_EDGE('',*,*,#4324,.F.);
#5785=ORIENTED_EDGE('',*,*,#4339,.F.);
#5786=ORIENTED_EDGE('',*,*,#4259,.F.);
#5787=ORIENTED_EDGE('',*,*,#4340,.F.);
#5788=ORIENTED_EDGE('',*,*,#4341,.F.);
#5789=ORIENTED_EDGE('',*,*,#4342,.T.);
#5790=ORIENTED_EDGE('',*,*,#4339,.T.);
#5791=ORIENTED_EDGE('',*,*,#4342,.F.);
#5792=ORIENTED_EDGE('',*,*,#4340,.T.);
#5793=ORIENTED_EDGE('',*,*,#4341,.T.);
#5794=ORIENTED_EDGE('',*,*,#4343,.F.);
#5795=ORIENTED_EDGE('',*,*,#4343,.T.);
#8348=CYLINDRICAL_SURFACE('',#9277,2.25);
#8349=CYLINDRICAL_SURFACE('',#9279,2.25);
#8350=CYLINDRICAL_SURFACE('',#9280,2.25);
#8351=CYLINDRICAL_SURFACE('',#9281,2.25);
#8352=CYLINDRICAL_SURFACE('',#9282,2.25);
#8353=CYLINDRICAL_SURFACE('',#9284,2.25);
#8354=CYLINDRICAL_SURFACE('',#9289,1.25);
#8355=CYLINDRICAL_SURFACE('',#9294,1.25);
#8356=CYLINDRICAL_SURFACE('',#9297,3.5);
#8581=ADVANCED_FACE('',(#518),#8348,.T.);
#8582=ADVANCED_FACE('',(#519),#8349,.T.);
#8583=ADVANCED_FACE('',(#520),#8350,.T.);
#8584=ADVANCED_FACE('',(#521),#8351,.T.);
#8585=ADVANCED_FACE('',(#522),#8352,.T.);
#8586=ADVANCED_FACE('',(#523),#409,.F.);
#8587=ADVANCED_FACE('',(#524),#8353,.T.);
#8588=ADVANCED_FACE('',(#525),#323,.T.);
#8589=ADVANCED_FACE('',(#526),#324,.T.);
#8590=ADVANCED_FACE('',(#527),#410,.T.);
#8591=ADVANCED_FACE('',(#528),#325,.T.);
#8592=ADVANCED_FACE('',(#529),#326,.T.);
#8593=ADVANCED_FACE('',(#530),#327,.T.);
#8594=ADVANCED_FACE('',(#531),#328,.T.);
#8595=ADVANCED_FACE('',(#532),#329,.T.);
#8596=ADVANCED_FACE('',(#533),#330,.T.);
#8597=ADVANCED_FACE('',(#534,#288),#411,.T.);
#8598=ADVANCED_FACE('',(#535),#8354,.F.);
#8599=ADVANCED_FACE('',(#536),#412,.F.);
#8600=ADVANCED_FACE('',(#537),#331,.T.);
#8601=ADVANCED_FACE('',(#538),#332,.T.);
#8602=ADVANCED_FACE('',(#539),#333,.T.);
#8603=ADVANCED_FACE('',(#540),#334,.T.);
#8604=ADVANCED_FACE('',(#541),#335,.T.);
#8605=ADVANCED_FACE('',(#542),#336,.T.);
#8606=ADVANCED_FACE('',(#543),#337,.T.);
#8607=ADVANCED_FACE('',(#544),#338,.T.);
#8608=ADVANCED_FACE('',(#545),#339,.T.);
#8609=ADVANCED_FACE('',(#546),#340,.T.);
#8610=ADVANCED_FACE('',(#547),#413,.T.);
#8611=ADVANCED_FACE('',(#548),#414,.T.);
#8612=ADVANCED_FACE('',(#549),#8355,.F.);
#8613=ADVANCED_FACE('',(#550),#341,.T.);
#8614=ADVANCED_FACE('',(#551),#342,.T.);
#8615=ADVANCED_FACE('',(#552,#289),#415,.F.);
#8616=ADVANCED_FACE('',(#553),#8356,.T.);
#8617=ADVANCED_FACE('',(#554),#284,.T.);
#9118=CLOSED_SHELL('',(#8581,#8582,#8583,#8584,#8585,#8586,#8587,#8588,
#8589,#8590,#8591,#8592,#8593,#8594,#8595,#8596,#8597,#8598,#8599,#8600,
#8601,#8602,#8603,#8604,#8605,#8606,#8607,#8608,#8609,#8610,#8611,#8612,
#8613,#8614,#8615,#8616,#8617));
#9276=AXIS2_PLACEMENT_3D('',#12546,#10212,#10213);
#9277=AXIS2_PLACEMENT_3D('',#12547,#10214,#10215);
#9278=AXIS2_PLACEMENT_3D('',#12606,#10218,#10219);
#9279=AXIS2_PLACEMENT_3D('',#12608,#10221,#10222);
#9280=AXIS2_PLACEMENT_3D('',#12718,#10224,#10225);
#9281=AXIS2_PLACEMENT_3D('',#12833,#10227,#10228);
#9282=AXIS2_PLACEMENT_3D('',#12948,#10230,#10231);
#9283=AXIS2_PLACEMENT_3D('',#13058,#10233,#10234);
#9284=AXIS2_PLACEMENT_3D('',#13086,#10235,#10236);
#9285=AXIS2_PLACEMENT_3D('',#13142,#10238,#10239);
#9286=AXIS2_PLACEMENT_3D('',#13605,#10242,#10243);
#9287=AXIS2_PLACEMENT_3D('',#15449,#10247,#10248);
#9288=AXIS2_PLACEMENT_3D('',#15452,#10249,#10250);
#9289=AXIS2_PLACEMENT_3D('',#15474,#10252,#10253);
#9290=AXIS2_PLACEMENT_3D('',#15517,#10255,#10256);
#9291=AXIS2_PLACEMENT_3D('',#18579,#10265,#10266);
#9292=AXIS2_PLACEMENT_3D('',#18684,#10268,#10269);
#9293=AXIS2_PLACEMENT_3D('',#18685,#10270,#10271);
#9294=AXIS2_PLACEMENT_3D('',#18687,#10273,#10274);
#9295=AXIS2_PLACEMENT_3D('',#18969,#10276,#10277);
#9296=AXIS2_PLACEMENT_3D('',#18971,#10278,#10279);
#9297=AXIS2_PLACEMENT_3D('',#18972,#10280,#10281);
#9298=AXIS2_PLACEMENT_3D('',#18975,#10282,#10283);
#9299=AXIS2_PLACEMENT_3D('',#18976,#10284,#10285);
#9300=AXIS2_PLACEMENT_3D('',#18978,#10287,#10288);
#9301=AXIS2_PLACEMENT_3D('',#18980,#10289,#10290);
#10212=DIRECTION('axis',(0.,0.,1.));
#10213=DIRECTION('refdir',(1.,0.,0.));
#10214=DIRECTION('center_axis',(1.,0.,0.));
#10215=DIRECTION('ref_axis',(0.,0.,1.));
#10216=DIRECTION('',(-1.,0.,0.));
#10217=DIRECTION('',(-1.,0.,0.));
#10218=DIRECTION('center_axis',(1.,0.,0.));
#10219=DIRECTION('ref_axis',(0.,0.,1.));
#10220=DIRECTION('',(1.,0.,0.));
#10221=DIRECTION('center_axis',(1.,0.,0.));
#10222=DIRECTION('ref_axis',(0.,0.,1.));
#10223=DIRECTION('',(-1.,0.,0.));
#10224=DIRECTION('center_axis',(1.,0.,0.));
#10225=DIRECTION('ref_axis',(0.,0.,1.));
#10226=DIRECTION('',(-1.,0.,0.));
#10227=DIRECTION('center_axis',(1.,0.,0.));
#10228=DIRECTION('ref_axis',(0.,0.,1.));
#10229=DIRECTION('',(-1.,0.,0.));
#10230=DIRECTION('center_axis',(1.,0.,0.));
#10231=DIRECTION('ref_axis',(0.,0.,1.));
#10232=DIRECTION('',(-1.,0.,0.));
#10233=DIRECTION('center_axis',(0.,1.,0.));
#10234=DIRECTION('ref_axis',(0.,0.,1.));
#10235=DIRECTION('center_axis',(1.,0.,0.));
#10236=DIRECTION('ref_axis',(0.,0.,1.));
#10237=DIRECTION('',(-1.,0.,0.));
#10238=DIRECTION('center_axis',(1.,0.,0.));
#10239=DIRECTION('ref_axis',(0.,0.,-1.));
#10240=DIRECTION('',(1.,0.,0.));
#10241=DIRECTION('',(-0.364960948531691,0.,0.931022827887076));
#10242=DIRECTION('center_axis',(0.,1.,0.));
#10243=DIRECTION('ref_axis',(0.,0.,1.));
#10244=DIRECTION('',(-0.364960948531691,0.,-0.931022827887076));
#10245=DIRECTION('',(-1.,0.,0.));
#10246=DIRECTION('',(-1.,0.,0.));
#10247=DIRECTION('center_axis',(1.,0.,0.));
#10248=DIRECTION('ref_axis',(0.,0.,1.));
#10249=DIRECTION('center_axis',(-1.,0.,0.));
#10250=DIRECTION('ref_axis',(0.,-0.939692620785897,0.342020143325699));
#10251=DIRECTION('',(0.,0.,1.));
#10252=DIRECTION('center_axis',(1.,0.,0.));
#10253=DIRECTION('ref_axis',(0.,0.820913047490338,0.571053209832609));
#10254=DIRECTION('',(-1.,0.,0.));
#10255=DIRECTION('center_axis',(0.,-1.,0.));
#10256=DIRECTION('ref_axis',(0.,0.,1.));
#10257=DIRECTION('',(-0.500000000000004,0.750000000000006,-0.433012701892204));
#10258=DIRECTION('',(-0.500000000000004,-0.750000000000006,0.433012701892204));
#10259=DIRECTION('',(-1.,0.,0.));
#10260=DIRECTION('',(-1.,0.,0.));
#10261=DIRECTION('',(-0.500000000000004,-0.750000000000006,-0.433012701892204));
#10262=DIRECTION('',(-0.500000000000004,0.750000000000006,0.433012701892204));
#10263=DIRECTION('',(-0.500000000000017,-3.68592187288512E-14,-0.866025403784429));
#10264=DIRECTION('',(-0.500000000000017,2.10167360932807E-14,0.866025403784429));
#10265=DIRECTION('center_axis',(1.,0.,0.));
#10266=DIRECTION('ref_axis',(0.,-1.,0.));
#10267=DIRECTION('',(0.,0.866025403784429,-0.500000000000017));
#10268=DIRECTION('center_axis',(1.,0.,0.));
#10269=DIRECTION('ref_axis',(0.,0.766044443118957,0.642787609686564));
#10270=DIRECTION('center_axis',(0.,0.500000000000017,0.866025403784429));
#10271=DIRECTION('ref_axis',(0.,0.866025403784429,-0.500000000000017));
#10272=DIRECTION('',(1.,1.9378438248E-14,-1.9378438248E-14));
#10273=DIRECTION('center_axis',(1.,0.,0.));
#10274=DIRECTION('ref_axis',(0.,-1.,0.));
#10275=DIRECTION('',(-1.,0.,0.));
#10276=DIRECTION('center_axis',(-1.,0.,0.));
#10277=DIRECTION('ref_axis',(0.,-1.,0.));
#10278=DIRECTION('center_axis',(-1.,0.,0.));
#10279=DIRECTION('ref_axis',(0.,-1.,0.));
#10280=DIRECTION('center_axis',(-1.,0.,0.));
#10281=DIRECTION('ref_axis',(0.,-1.,0.));
#10282=DIRECTION('center_axis',(-1.,0.,0.));
#10283=DIRECTION('ref_axis',(0.,0.,-1.));
#10284=DIRECTION('center_axis',(-1.,0.,0.));
#10285=DIRECTION('ref_axis',(0.,0.,-1.));
#10286=DIRECTION('',(1.,0.,0.));
#10287=DIRECTION('center_axis',(-1.,0.,-6.12323399573677E-17));
#10288=DIRECTION('ref_axis',(0.,0.,-1.));
#10289=DIRECTION('center_axis',(0.,1.,-1.22464679914735E-16));
#10290=DIRECTION('ref_axis',(0.,1.22464679914735E-16,1.));
#12546=CARTESIAN_POINT('',(0.,0.,0.));
#12547=CARTESIAN_POINT('Origin',(-1.62,0.,0.));
#12548=CARTESIAN_POINT('',(2.35200870842004,-6.73733496176535E-9,-2.25));
#12549=CARTESIAN_POINT('',(1.56784454507149,1.7551195425239E-10,-2.24999999965197));
#12550=CARTESIAN_POINT('',(-1.62,2.75545529808154E-16,-2.25));
#12551=CARTESIAN_POINT('',(0.392128505845514,-1.44267263157291E-10,-2.24999999971305));
#12552=CARTESIAN_POINT('Ctrl Pts',(2.35200870842004,-1.34746699562149E-8,
-2.25));
#12553=CARTESIAN_POINT('Ctrl Pts',(2.33277638732405,-0.138949662434125,
-2.24999999916787));
#12554=CARTESIAN_POINT('Ctrl Pts',(2.3136433948348,-0.277617289677986,-2.23712870695244));
#12555=CARTESIAN_POINT('Ctrl Pts',(2.25366806067718,-0.703379839167081,
-2.1573828637615));
#12556=CARTESIAN_POINT('Ctrl Pts',(2.2129900387638,-0.979129299035637,-2.04703573040602));
#12557=CARTESIAN_POINT('Ctrl Pts',(2.1519494185931,-1.34948810995398,-1.80641324461668));
#12558=CARTESIAN_POINT('Ctrl Pts',(2.13161296068056,-1.46494615839442,-1.71411097634091));
#12559=CARTESIAN_POINT('Ctrl Pts',(2.09075399170948,-1.67573316142329,-1.5086415298124));
#12560=CARTESIAN_POINT('Ctrl Pts',(2.07032661889744,-1.77063375674575,-1.39604313280329));
#12561=CARTESIAN_POINT('Ctrl Pts',(2.00943863336491,-2.01920756533226,-1.03461219332703));
#12562=CARTESIAN_POINT('Ctrl Pts',(1.96964374375012,-2.13620985812946,-0.764346996059495));
#12563=CARTESIAN_POINT('Ctrl Pts',(1.90863622394457,-2.22966512019371,-0.335697586507395));
#12564=CARTESIAN_POINT('Ctrl Pts',(1.88823238081986,-2.24682944376116,-0.189372254756062));
#12565=CARTESIAN_POINT('Ctrl Pts',(1.84758268312515,-2.25236953127332,0.104468846512095));
#12566=CARTESIAN_POINT('Ctrl Pts',(1.82735396185634,-2.2407466408021,0.251267624447377));
#12567=CARTESIAN_POINT('Ctrl Pts',(1.78658703445223,-2.18899287867358,0.540823217609736));
#12568=CARTESIAN_POINT('Ctrl Pts',(1.76614227354399,-2.14892212598486,0.682869172878815));
#12569=CARTESIAN_POINT('Ctrl Pts',(1.70455376263095,-1.98749481790983,1.09536189156463));
#12570=CARTESIAN_POINT('Ctrl Pts',(1.66426251715545,-1.82648095233547,1.34681950231116));
#12571=CARTESIAN_POINT('Ctrl Pts',(1.60278209700345,-1.51969407244708,1.66570454228107));
#12572=CARTESIAN_POINT('Ctrl Pts',(1.58236836207887,-1.40782894454456,1.76126713241198));
#12573=CARTESIAN_POINT('Ctrl Pts',(1.54176994137328,-1.16750131542141,1.92894618385223));
#12574=CARTESIAN_POINT('Ctrl Pts',(1.52164437281176,-1.03967309036386,2.00074327125064));
#12575=CARTESIAN_POINT('Ctrl Pts',(1.46063877929285,-0.636221828820066,
2.17817317037249));
#12576=CARTESIAN_POINT('Ctrl Pts',(1.41990733277731,-0.345990135231769,
2.24265729999344));
#12577=CARTESIAN_POINT('Ctrl Pts',(1.35883501404012,0.0957467405484846,
2.25278719152739));
#12578=CARTESIAN_POINT('Ctrl Pts',(1.33852020218053,0.24304733990133,2.24168299296819));
#12579=CARTESIAN_POINT('Ctrl Pts',(1.29767897011706,0.532963956491612,2.19090165010054));
#12580=CARTESIAN_POINT('Ctrl Pts',(1.27724738626119,0.674898225257669,2.15142088265007));
#12581=CARTESIAN_POINT('Ctrl Pts',(1.21614110621229,1.08525868713529,1.9926333773732));
#12582=CARTESIAN_POINT('Ctrl Pts',(1.17619137834493,1.33527754707148,1.83450427328792));
#12583=CARTESIAN_POINT('Ctrl Pts',(1.11502332698973,1.65455281674558,1.53183980918237));
#12584=CARTESIAN_POINT('Ctrl Pts',(1.09461843507782,1.75101288969669,1.42057620764718));
#12585=CARTESIAN_POINT('Ctrl Pts',(1.05398607569683,1.92079184507726,1.18093297112612));
#12586=CARTESIAN_POINT('Ctrl Pts',(1.03377939642206,1.99371911206047,1.05315109711181));
#12587=CARTESIAN_POINT('Ctrl Pts',(0.993032597292335,2.11385925129569,0.784728189120789));
#12588=CARTESIAN_POINT('Ctrl Pts',(0.972585546096863,2.16068641849123,0.644693860742182));
#12589=CARTESIAN_POINT('Ctrl Pts',(0.910938101623354,2.2594151089232,0.212521738300102));
#12590=CARTESIAN_POINT('Ctrl Pts',(0.870603876065813,2.26774929129372,-0.0862475998130358));
#12591=CARTESIAN_POINT('Ctrl Pts',(0.809095780672101,2.19334836312328,-0.522750349456467));
#12592=CARTESIAN_POINT('Ctrl Pts',(0.788678651829075,2.15458504182036,-0.664687866011266));
#12593=CARTESIAN_POINT('Ctrl Pts',(0.748076415375149,2.05019231544315,-0.938386614720418));
#12594=CARTESIAN_POINT('Ctrl Pts',(0.727967451926541,1.98492979001699,-1.06953883009641));
#12595=CARTESIAN_POINT('Ctrl Pts',(0.66695908632401,1.75109360472821,-1.44326800323482));
#12596=CARTESIAN_POINT('Ctrl Pts',(0.62618961791159,1.54720453400115,-1.65997389246564));
#12597=CARTESIAN_POINT('Ctrl Pts',(0.56940574368058,1.21284296473895,-1.89868238190458));
#12598=CARTESIAN_POINT('Ctrl Pts',(0.553392895611178,1.11326053025777,-1.95873245111983));
#12599=CARTESIAN_POINT('Ctrl Pts',(0.513121790218507,0.853450251020534,
-2.08916451042388));
#12600=CARTESIAN_POINT('Ctrl Pts',(0.488882293379238,0.688823957401331,
-2.14907018596128));
#12601=CARTESIAN_POINT('Ctrl Pts',(0.440333302359495,0.348906643869198,
-2.2296414081572));
#12602=CARTESIAN_POINT('Ctrl Pts',(0.416310037109522,0.174759273682914,
-2.25000000001581));
#12603=CARTESIAN_POINT('Ctrl Pts',(0.392128506274274,-2.03592837033639E-10,
-2.25));
#12604=CARTESIAN_POINT('',(-1.12,0.,-2.25));
#12605=CARTESIAN_POINT('',(-1.62,2.75545529808154E-16,-2.25));
#12606=CARTESIAN_POINT('Origin',(-1.12,0.,0.));
#12607=CARTESIAN_POINT('',(0.392,0.,-2.25));
#12608=CARTESIAN_POINT('Origin',(-1.62,0.,0.));
#12609=CARTESIAN_POINT('',(4.31209250605754,-4.71354290851659E-8,-2.25));
#12610=CARTESIAN_POINT('',(3.52798225106248,1.06028063402371E-8,-2.25));
#12611=CARTESIAN_POINT('',(-1.62,2.75545529808154E-16,-2.25));
#12612=CARTESIAN_POINT('Ctrl Pts',(4.31209251248913,-4.8029842897669E-8,
-2.25));
#12613=CARTESIAN_POINT('Ctrl Pts',(4.3096836921749,-0.0173186732513607,
-2.24999999963031));
#12614=CARTESIAN_POINT('Ctrl Pts',(4.30727412907853,-0.0346409650931408,
-2.24980004305779));
#12615=CARTESIAN_POINT('Ctrl Pts',(4.26390032233211,-0.346378474343082,
-2.24259857970738));
#12616=CARTESIAN_POINT('Ctrl Pts',(4.22372857992966,-0.636620042927198,
-2.17806075975736));
#12617=CARTESIAN_POINT('Ctrl Pts',(4.16255591602526,-1.0400654841798,-2.00053948582208));
#12618=CARTESIAN_POINT('Ctrl Pts',(4.14221936692873,-1.16788321487765,-1.92871521092846));
#12619=CARTESIAN_POINT('Ctrl Pts',(4.10153463416861,-1.40816256393229,-1.76099865177231));
#12620=CARTESIAN_POINT('Ctrl Pts',(4.08133681215282,-1.52000051536649,-1.66542465736685));
#12621=CARTESIAN_POINT('Ctrl Pts',(4.02014872279012,-1.82670962668572,-1.34650379086338));
#12622=CARTESIAN_POINT('Ctrl Pts',(3.97923702176023,-1.98766869768262,-1.09504016666849));
#12623=CARTESIAN_POINT('Ctrl Pts',(3.91797084687114,-2.1490285267146,-0.682536143298372));
#12624=CARTESIAN_POINT('Ctrl Pts',(3.89769729492075,-2.18907646066102,-0.540483248301418));
#12625=CARTESIAN_POINT('Ctrl Pts',(3.85692869629777,-2.24078837892765,-0.250906415087508));
#12626=CARTESIAN_POINT('Ctrl Pts',(3.83652802221641,-2.25238725782488,-0.104092586806907));
#12627=CARTESIAN_POINT('Ctrl Pts',(3.79566850402458,-2.2467980137086,0.189719065307968));
#12628=CARTESIAN_POINT('Ctrl Pts',(3.77539635985123,-2.22961601599269,0.336022905307451));
#12629=CARTESIAN_POINT('Ctrl Pts',(3.71475827653615,-2.13609374147413,0.76468053512841));
#12630=CARTESIAN_POINT('Ctrl Pts',(3.67444889417311,-2.01903786410996,1.03494295741834));
#12631=CARTESIAN_POINT('Ctrl Pts',(3.61365957837694,-1.77041013913102,1.39632589673724));
#12632=CARTESIAN_POINT('Ctrl Pts',(3.59344857673001,-1.6754969521165,1.50890339956332));
#12633=CARTESIAN_POINT('Ctrl Pts',(3.55270646116513,-1.46466091956622,1.71435719882085));
#12634=CARTESIAN_POINT('Ctrl Pts',(3.53226843656,-1.34917295652032,1.80664890853136));
#12635=CARTESIAN_POINT('Ctrl Pts',(3.47083314749689,-0.978766159167189,
2.0472098780982));
#12636=CARTESIAN_POINT('Ctrl Pts',(3.43067952500035,-0.702981415412188,
2.15751642705047));
#12637=CARTESIAN_POINT('Ctrl Pts',(3.36954546604559,-0.269851280770565,
2.23855388857242));
#12638=CARTESIAN_POINT('Ctrl Pts',(3.34919136760675,-0.123629571159131,
2.25136791167734));
#12639=CARTESIAN_POINT('Ctrl Pts',(3.30846337269836,0.169554513911013,2.24839775051071));
#12640=CARTESIAN_POINT('Ctrl Pts',(3.28825578849117,0.315822445267529,2.23255470585241));
#12641=CARTESIAN_POINT('Ctrl Pts',(3.22715306326724,0.748446928600913,2.14229924286184));
#12642=CARTESIAN_POINT('Ctrl Pts',(3.18632278838618,1.02271595912037,2.02575126538499));
#12643=CARTESIAN_POINT('Ctrl Pts',(3.12512300392732,1.38827462433469,1.77675178903506));
#12644=CARTESIAN_POINT('Ctrl Pts',(3.10486681051267,1.5014717162221,1.68218171628064));
#12645=CARTESIAN_POINT('Ctrl Pts',(3.06410287513668,1.70772615377232,1.47234662177451));
#12646=CARTESIAN_POINT('Ctrl Pts',(3.04368915577137,1.80029296917859,1.35759899910148));
#12647=CARTESIAN_POINT('Ctrl Pts',(3.00278457893002,1.96169182729548,1.11170665051441));
#12648=CARTESIAN_POINT('Ctrl Pts',(2.98247979590209,2.03014491871399,0.981143626178216));
#12649=CARTESIAN_POINT('Ctrl Pts',(2.92212349573607,2.19412631916938,0.576373576555818));
#12650=CARTESIAN_POINT('Ctrl Pts',(2.88214235426619,2.25002453221374,0.289429263379427));
#12651=CARTESIAN_POINT('Ctrl Pts',(2.80180325462564,2.24997545071142,-0.289821426149872));
#12652=CARTESIAN_POINT('Ctrl Pts',(2.76226046746642,2.1940276179487,-0.576737472505687));
#12653=CARTESIAN_POINT('Ctrl Pts',(2.70152461771704,2.02999121891702,-0.981461835728237));
#12654=CARTESIAN_POINT('Ctrl Pts',(2.68112151868365,1.96150972560333,-1.11203260815236));
#12655=CARTESIAN_POINT('Ctrl Pts',(2.64044620380749,1.80004928023798,-1.35792161134074));
#12656=CARTESIAN_POINT('Ctrl Pts',(2.6201897172147,1.70747036178314,-1.47264103442275));
#12657=CARTESIAN_POINT('Ctrl Pts',(2.57939813892615,1.50119327929904,-1.68243069966521));
#12658=CARTESIAN_POINT('Ctrl Pts',(2.55895696088971,1.38797891913171,-1.77698237260967));
#12659=CARTESIAN_POINT('Ctrl Pts',(2.49747399935976,1.02236832477551,-2.02592944165093));
#12660=CARTESIAN_POINT('Ctrl Pts',(2.45725819439494,0.748063370721404,-2.14243526276714));
#12661=CARTESIAN_POINT('Ctrl Pts',(2.39583737585762,0.315405218933968,-2.23261384171523));
#12662=CARTESIAN_POINT('Ctrl Pts',(2.37542727449016,0.169119063455048,-2.24843215995123));
#12663=CARTESIAN_POINT('Ctrl Pts',(2.3540695508737,0.0148876676420556,-2.24996306357395));
#12664=CARTESIAN_POINT('Ctrl Pts',(2.35303897077726,0.0074434246915941,
-2.25000000004458));
#12665=CARTESIAN_POINT('Ctrl Pts',(2.35200870842004,-1.34746697823107E-8,
-2.25));
#12666=CARTESIAN_POINT('Ctrl Pts',(1.56784454455142,2.47754351756502E-10,
-2.25));
#12667=CARTESIAN_POINT('Ctrl Pts',(1.59211895035072,0.17479682892967,-2.24999999998075));
#12668=CARTESIAN_POINT('Ctrl Pts',(1.61641651664107,0.348995564145036,-2.22963234048382));
#12669=CARTESIAN_POINT('Ctrl Pts',(1.66478847007177,0.689026197844474,-2.1490102399816));
#12670=CARTESIAN_POINT('Ctrl Pts',(1.68879344734741,0.853692883134347,-2.08906901944099));
#12671=CARTESIAN_POINT('Ctrl Pts',(1.72911468700117,1.11355858179884,-1.95856528032236));
#12672=CARTESIAN_POINT('Ctrl Pts',(1.74524575915888,1.21315915341977,-1.89848197821454));
#12673=CARTESIAN_POINT('Ctrl Pts',(1.80239810265935,1.54751075606308,-1.65969083865729));
#12674=CARTESIAN_POINT('Ctrl Pts',(1.8425875741646,1.75137701442023,-1.44293043674562));
#12675=CARTESIAN_POINT('Ctrl Pts',(1.9037906929622,1.98515120720636,-1.06912759367124));
#12676=CARTESIAN_POINT('Ctrl Pts',(1.92411338573857,2.0503869387489,-0.937961715305248));
#12677=CARTESIAN_POINT('Ctrl Pts',(1.96476482028555,2.15471718118683,-0.664255413906532));
#12678=CARTESIAN_POINT('Ctrl Pts',(1.98495972725598,2.19345036446728,-0.522321200366432));
#12679=CARTESIAN_POINT('Ctrl Pts',(2.04619880723112,2.26776069914933,-0.0858385456680671));
#12680=CARTESIAN_POINT('Ctrl Pts',(2.08715131373674,2.25937622499644,0.212900405402588));
#12681=CARTESIAN_POINT('Ctrl Pts',(2.14845223284548,2.16058263016293,0.645044248508482));
#12682=CARTESIAN_POINT('Ctrl Pts',(2.16874000501105,2.11373097647935,0.785072614123205));
#12683=CARTESIAN_POINT('Ctrl Pts',(2.20951134791998,1.99354329671921,1.0534861431364));
#12684=CARTESIAN_POINT('Ctrl Pts',(2.22990026726523,1.9205878078923,1.18126534091795));
#12685=CARTESIAN_POINT('Ctrl Pts',(2.27072327240798,1.75078233631504,1.42085711461194));
#12686=CARTESIAN_POINT('Ctrl Pts',(2.29097278202136,1.65431840297454,1.53209280458974));
#12687=CARTESIAN_POINT('Ctrl Pts',(2.35178136990745,1.33499069778918,1.83471469093413));
#12688=CARTESIAN_POINT('Ctrl Pts',(2.39228770211503,1.08494074352961,1.99280530690906));
#12689=CARTESIAN_POINT('Ctrl Pts',(2.45323161358009,0.674566773852937,2.15152456699413));
#12690=CARTESIAN_POINT('Ctrl Pts',(2.47345385186549,0.532632319946515,2.1909819434057));
#12691=CARTESIAN_POINT('Ctrl Pts',(2.51420325307758,0.242686200374217,2.24172393096506));
#12692=CARTESIAN_POINT('Ctrl Pts',(2.53463709303976,0.0953672317794488,
2.25280354062975));
#12693=CARTESIAN_POINT('Ctrl Pts',(2.59610004747896,-0.346381125090515,
2.24259817496518));
#12694=CARTESIAN_POINT('Ctrl Pts',(2.63627179232953,-0.636622652438412,
2.17806000181052));
#12695=CARTESIAN_POINT('Ctrl Pts',(2.69744446087517,-1.04006789323018,2.00053823197433));
#12696=CARTESIAN_POINT('Ctrl Pts',(2.71778100791431,-1.16788552105996,1.92871381304625));
#12697=CARTESIAN_POINT('Ctrl Pts',(2.75846573572112,-1.40816465574277,1.76099697910864));
#12698=CARTESIAN_POINT('Ctrl Pts',(2.77866355700581,-1.52000249393371,1.66542285158641));
#12699=CARTESIAN_POINT('Ctrl Pts',(2.83985165482856,-1.82671126135403,1.34650158425958));
#12700=CARTESIAN_POINT('Ctrl Pts',(2.88076336322876,-1.98767005323287,1.09503771980515));
#12701=CARTESIAN_POINT('Ctrl Pts',(2.94202954427547,-2.14902938680981,0.682533437385133));
#12702=CARTESIAN_POINT('Ctrl Pts',(2.96230309827855,-2.18907714428284,0.540480482169972));
#12703=CARTESIAN_POINT('Ctrl Pts',(3.00307169736765,-2.24078869377107,0.250903592223416));
#12704=CARTESIAN_POINT('Ctrl Pts',(3.0234723698216,-2.25238738686191,0.104089768228522));
#12705=CARTESIAN_POINT('Ctrl Pts',(3.06433188272785,-2.24679777808941,-0.189721846837428));
#12706=CARTESIAN_POINT('Ctrl Pts',(3.08460402337628,-2.22961560096571,-0.336025654074097));
#12707=CARTESIAN_POINT('Ctrl Pts',(3.14524213459954,-2.13609275790457,-0.764683362701376));
#12708=CARTESIAN_POINT('Ctrl Pts',(3.18555154937213,-2.0190364256806,-1.03494582298224));
#12709=CARTESIAN_POINT('Ctrl Pts',(3.24634089062226,-1.77040803178236,-1.39632856968566));
#12710=CARTESIAN_POINT('Ctrl Pts',(3.26655189380965,-1.67549466831335,-1.50890593643214));
#12711=CARTESIAN_POINT('Ctrl Pts',(3.30729401050766,-1.46465832691475,-1.71435941266956));
#12712=CARTESIAN_POINT('Ctrl Pts',(3.32773203467332,-1.34917023535203,-1.80665093953558));
#12713=CARTESIAN_POINT('Ctrl Pts',(3.3891673279893,-0.978763052959974,-2.04721136927531));
#12714=CARTESIAN_POINT('Ctrl Pts',(3.42932095269871,-0.702978100313755,
-2.1575175129611));
#12715=CARTESIAN_POINT('Ctrl Pts',(3.48940060268209,-0.277318270540816,
-2.2371566154978));
#12716=CARTESIAN_POINT('Ctrl Pts',(3.50869452424106,-0.13879770411982,-2.25000000066645));
#12717=CARTESIAN_POINT('Ctrl Pts',(3.52798224961699,1.08036556437097E-8,
-2.25));
#12718=CARTESIAN_POINT('Origin',(-1.62,0.,0.));
#12719=CARTESIAN_POINT('',(6.27207431538479,-3.77424972188349E-8,-2.25));
#12720=CARTESIAN_POINT('',(5.48792568467742,3.79675638141282E-8,-2.25));
#12721=CARTESIAN_POINT('',(-1.62,2.75545529808154E-16,-2.25));
#12722=CARTESIAN_POINT('',(5.29204615187795,3.82768812034955E-6,2.2500376859885));
#12723=CARTESIAN_POINT('Ctrl Pts',(6.27207432050307,-3.84499440619912E-8,
-2.25));
#12724=CARTESIAN_POINT('Ctrl Pts',(6.25408532734062,-0.130165591604654,
-2.24999999777562));
#12725=CARTESIAN_POINT('Ctrl Pts',(6.23611633433344,-0.260113717555053,
-2.2387046819596));
#12726=CARTESIAN_POINT('Ctrl Pts',(6.19765297673759,-0.533145965110677,
-2.19085732779874));
#12727=CARTESIAN_POINT('Ctrl Pts',(6.17722142712748,-0.675076412010008,
-2.15136493955894));
#12728=CARTESIAN_POINT('Ctrl Pts',(6.11611677525103,-1.08541438319642,-1.99254717511697));
#12729=CARTESIAN_POINT('Ctrl Pts',(6.07616819926228,-1.33541291644883,-1.83440421567511));
#12730=CARTESIAN_POINT('Ctrl Pts',(6.01500131723825,-1.6546604838004,-1.53172356103907));
#12731=CARTESIAN_POINT('Ctrl Pts',(5.99459643609767,-1.75111308725479,-1.42045275172777));
#12732=CARTESIAN_POINT('Ctrl Pts',(5.95396394316539,-1.92087604585497,-1.18079614519214));
#12733=CARTESIAN_POINT('Ctrl Pts',(5.93375707907688,-1.99379472607352,-1.05300809263716));
#12734=CARTESIAN_POINT('Ctrl Pts',(5.89301010919162,-2.11391569789108,-0.784576015091131));
#12735=CARTESIAN_POINT('Ctrl Pts',(5.87256307521049,-2.1607326268593,-0.644538848405556));
#12736=CARTESIAN_POINT('Ctrl Pts',(5.81091604648748,-2.25942987283393,-0.212362060682051));
#12737=CARTESIAN_POINT('Ctrl Pts',(5.77058213474394,-2.26774301450112,0.0864058887794901));
#12738=CARTESIAN_POINT('Ctrl Pts',(5.70907421085162,-2.19331233614171,0.522901439395613));
#12739=CARTESIAN_POINT('Ctrl Pts',(5.68865711036259,-2.15453928606102,0.664836132781844));
#12740=CARTESIAN_POINT('Ctrl Pts',(5.64805491001764,-2.05012742522628,0.938528535781674));
#12741=CARTESIAN_POINT('Ctrl Pts',(5.62794579809253,-1.9848553301936,1.06967714620222));
#12742=CARTESIAN_POINT('Ctrl Pts',(5.56693746455699,-1.75099350503924,1.44338901773155));
#12743=CARTESIAN_POINT('Ctrl Pts',(5.52616833815168,-1.54709100449272,1.66007933403282));
#12744=CARTESIAN_POINT('Ctrl Pts',(5.46938273005178,-1.21270280996112,1.89877282192696));
#12745=CARTESIAN_POINT('Ctrl Pts',(5.45336778929448,-1.11310280591162,1.95882297685515));
#12746=CARTESIAN_POINT('Ctrl Pts',(5.41309150365977,-0.853248456719158,
2.08924873488907));
#12747=CARTESIAN_POINT('Ctrl Pts',(5.38884891316524,-0.688595612688673,
2.14914511344005));
#12748=CARTESIAN_POINT('Ctrl Pts',(5.34030897001841,-0.348730902642399,
2.22966222455927));
#12749=CARTESIAN_POINT('Ctrl Pts',(5.31629606784201,-0.174658290764173,
2.2500011638322));
#12750=CARTESIAN_POINT('Ctrl Pts',(5.29212643182535,1.49921888440568E-5,
2.24999999995005));
#12751=CARTESIAN_POINT('Ctrl Pts',(5.29215286593614,1.86469866857858E-5,
2.24999999992273));
#12752=CARTESIAN_POINT('Ctrl Pts',(5.26788459471967,0.174771258645414,2.24999855165179));
#12753=CARTESIAN_POINT('Ctrl Pts',(5.24359172922835,0.348936080922872,2.22963821621658));
#12754=CARTESIAN_POINT('Ctrl Pts',(5.19522294699834,0.688947458703098,2.1490371277111));
#12755=CARTESIAN_POINT('Ctrl Pts',(5.17121524420815,0.85363528418937,2.08909424764715));
#12756=CARTESIAN_POINT('Ctrl Pts',(5.13088935441657,1.11353358772044,1.95858029077967));
#12757=CARTESIAN_POINT('Ctrl Pts',(5.11475641692752,1.21314635881947,1.89849097930423));
#12758=CARTESIAN_POINT('Ctrl Pts',(5.05760220103249,1.54750914204975,1.65969233824127));
#12759=CARTESIAN_POINT('Ctrl Pts',(5.01741273190551,1.75137559127931,1.44293215801028));
#12760=CARTESIAN_POINT('Ctrl Pts',(4.956209617063,1.98515014899732,1.06912956060157));
#12761=CARTESIAN_POINT('Ctrl Pts',(4.93588692261656,2.05038601671524,0.937963733178924));
#12762=CARTESIAN_POINT('Ctrl Pts',(4.89523548415118,2.15471653107058,0.664257522211146));
#12763=CARTESIAN_POINT('Ctrl Pts',(4.87504057714961,2.19344985264303,0.522323349061616));
#12764=CARTESIAN_POINT('Ctrl Pts',(4.81380150253075,2.26776061051127,0.0858407957701425));
#12765=CARTESIAN_POINT('Ctrl Pts',(4.77284899967315,2.25937643530655,-0.212898136213141));
#12766=CARTESIAN_POINT('Ctrl Pts',(4.71154808385884,2.16058328727759,-0.645042045642452));
#12767=CARTESIAN_POINT('Ctrl Pts',(4.69126031340649,2.11373177917323,-0.785070451457586));
#12768=CARTESIAN_POINT('Ctrl Pts',(4.65048897078392,1.99354437168984,-1.05348411115453));
#12769=CARTESIAN_POINT('Ctrl Pts',(4.63010004997872,1.92058900476889,-1.18126339690632));
#12770=CARTESIAN_POINT('Ctrl Pts',(4.58927704048005,1.75078376058498,-1.42085536040784));
#12771=CARTESIAN_POINT('Ctrl Pts',(4.56902752837063,1.65431993345513,-1.53209115275161));
#12772=CARTESIAN_POINT('Ctrl Pts',(4.5082189584666,1.33499262069522,-1.83471327046107));
#12773=CARTESIAN_POINT('Ctrl Pts',(4.46771264686281,1.08494295367164,-1.99280408393575));
#12774=CARTESIAN_POINT('Ctrl Pts',(4.4067687515742,0.674569302753384,-2.15152377353736));
#12775=CARTESIAN_POINT('Ctrl Pts',(4.38654651469855,0.532634903269586,-2.19098131485047));
#12776=CARTESIAN_POINT('Ctrl Pts',(4.34819606392266,0.259758194840745,-2.23873640467835));
#12777=CARTESIAN_POINT('Ctrl Pts',(4.33017143806453,0.129981476370136,-2.25000000277466));
#12778=CARTESIAN_POINT('Ctrl Pts',(4.31209251248913,-4.80298429847426E-8,
-2.25));
#12779=CARTESIAN_POINT('Ctrl Pts',(3.52798224961699,1.08036555900686E-8,
-2.25));
#12780=CARTESIAN_POINT('Ctrl Pts',(3.52903809419908,0.00759804595041996,
-2.24999999996352));
#12781=CARTESIAN_POINT('Ctrl Pts',(3.53009386946379,0.0151969186709084,
-2.24996151317907));
#12782=CARTESIAN_POINT('Ctrl Pts',(3.55153710138858,0.169557933752482,-2.24839749237712));
#12783=CARTESIAN_POINT('Ctrl Pts',(3.57174468363663,0.315825837333526,-2.2325542257493));
#12784=CARTESIAN_POINT('Ctrl Pts',(3.63284742363824,0.748450276953202,-2.14229808671015));
#12785=CARTESIAN_POINT('Ctrl Pts',(3.67367771353097,1.02271921695567,-2.02574963515858));
#12786=CARTESIAN_POINT('Ctrl Pts',(3.73487751004098,1.38827756485256,-1.77674949253261));
#12787=CARTESIAN_POINT('Ctrl Pts',(3.75513370599362,1.50147451002373,-1.68217922372651));
#12788=CARTESIAN_POINT('Ctrl Pts',(3.79589764216434,1.70772859083133,-1.47234379280653));
#12789=CARTESIAN_POINT('Ctrl Pts',(3.81631135973467,1.80029520233142,-1.35759603527156));
#12790=CARTESIAN_POINT('Ctrl Pts',(3.8572159299359,1.96169363605914,-1.11170345647742));
#12791=CARTESIAN_POINT('Ctrl Pts',(3.87752070776928,2.03014650713162,-0.981140336813649));
#12792=CARTESIAN_POINT('Ctrl Pts',(3.93787705708652,2.19412738785583,-0.576369694984279));
#12793=CARTESIAN_POINT('Ctrl Pts',(3.97785825589419,2.2500251408795,-0.289424903347084));
#12794=CARTESIAN_POINT('Ctrl Pts',(4.05819741292109,2.24997484101667,0.289826277868796));
#12795=CARTESIAN_POINT('Ctrl Pts',(4.09774022238688,2.19402635884467,0.576742322258415));
#12796=CARTESIAN_POINT('Ctrl Pts',(4.15847609373613,2.02998899065074,0.981466448251175));
#12797=CARTESIAN_POINT('Ctrl Pts',(4.17887919265677,1.96150718828485,1.11203708702209));
#12798=CARTESIAN_POINT('Ctrl Pts',(4.21955451327411,1.80004614748845,1.35792576754677));
#12799=CARTESIAN_POINT('Ctrl Pts',(4.23981100566145,1.70746694325715,1.4726450012244));
#12800=CARTESIAN_POINT('Ctrl Pts',(4.28060258902202,1.50118936105739,1.68243419423437));
#12801=CARTESIAN_POINT('Ctrl Pts',(4.30104376623934,1.38797479489467,1.77698559252924));
#12802=CARTESIAN_POINT('Ctrl Pts',(4.36252670165228,1.02236375565302,2.02593172692336));
#12803=CARTESIAN_POINT('Ctrl Pts',(4.40274248808703,0.748058676427634,2.14243688239479));
#12804=CARTESIAN_POINT('Ctrl Pts',(4.46416329089555,0.315400465914695,2.23261451352336));
#12805=CARTESIAN_POINT('Ctrl Pts',(4.48457339157346,0.169114271160377,2.24843252078476));
#12806=CARTESIAN_POINT('Ctrl Pts',(4.52517609820414,-0.124091736174342,
2.25134226315683));
#12807=CARTESIAN_POINT('Ctrl Pts',(4.54532642928959,-0.270304179716033,
2.23849878605978));
#12808=CARTESIAN_POINT('Ctrl Pts',(4.60633261296772,-0.703384484216852,
2.15738134133833));
#12809=CARTESIAN_POINT('Ctrl Pts',(4.64701062369311,-0.979133652254152,
2.04703363983638));
#12810=CARTESIAN_POINT('Ctrl Pts',(4.70805123769189,-1.34949192457293,1.80641039645255));
#12811=CARTESIAN_POINT('Ctrl Pts',(4.72838769996192,-1.46494979275193,1.71410787190213));
#12812=CARTESIAN_POINT('Ctrl Pts',(4.76924667246394,-1.6757363624887,1.50863797289603));
#12813=CARTESIAN_POINT('Ctrl Pts',(4.78967404439193,-1.77063671067734,1.39603938489405));
#12814=CARTESIAN_POINT('Ctrl Pts',(4.8505619800633,-2.0192095809236,1.03460817590125));
#12815=CARTESIAN_POINT('Ctrl Pts',(4.89035683420762,-2.136211235017,0.764343034593591));
#12816=CARTESIAN_POINT('Ctrl Pts',(4.95136431657638,-2.22966570058694,0.335693738657983));
#12817=CARTESIAN_POINT('Ctrl Pts',(4.97176815953602,-2.24682977301417,0.189368360942901));
#12818=CARTESIAN_POINT('Ctrl Pts',(5.01241786106949,-2.25236934995637,-0.104472792493422));
#12819=CARTESIAN_POINT('Ctrl Pts',(5.03264658685133,-2.24074619937062,-0.251271576130403));
#12820=CARTESIAN_POINT('Ctrl Pts',(5.0734135183212,-2.18899192118144,-0.540827089300053));
#12821=CARTESIAN_POINT('Ctrl Pts',(5.09385827870535,-2.14892092142864,-0.682872960558762));
#12822=CARTESIAN_POINT('Ctrl Pts',(5.15544677542526,-1.98749291968624,-1.09536531654571));
#12823=CARTESIAN_POINT('Ctrl Pts',(5.19573801061881,-1.82647866393059,-1.34682258994401));
#12824=CARTESIAN_POINT('Ctrl Pts',(5.25721842344305,-1.51969130410301,-1.66570706791729));
#12825=CARTESIAN_POINT('Ctrl Pts',(5.27763215772858,-1.40782601752243,-1.76126947206421));
#12826=CARTESIAN_POINT('Ctrl Pts',(5.31823057856148,-1.16749808807915,-1.92894813920351));
#12827=CARTESIAN_POINT('Ctrl Pts',(5.3383561510158,-1.03966971950341,-2.0007450247888));
#12828=CARTESIAN_POINT('Ctrl Pts',(5.39936174428246,-0.636218178201016,
-2.17817423002739));
#12829=CARTESIAN_POINT('Ctrl Pts',(5.44009318222189,-0.34598642648124,-2.24265786574736));
#12830=CARTESIAN_POINT('Ctrl Pts',(5.48317363486213,-0.0343849350021253,
-2.24980298931542));
#12831=CARTESIAN_POINT('Ctrl Pts',(5.48554992285105,-0.0171905666706365,
-2.25000000029552));
#12832=CARTESIAN_POINT('Ctrl Pts',(5.48792567952862,3.86792288330504E-8,
-2.25));
#12833=CARTESIAN_POINT('Origin',(-1.62,0.,0.));
#12834=CARTESIAN_POINT('',(8.23201774889606,-1.07519836100082E-8,-2.25));
#12835=CARTESIAN_POINT('',(7.44790749394411,4.71413583506493E-8,-2.25));
#12836=CARTESIAN_POINT('',(-1.62,2.75545529808154E-16,-2.25));
#12837=CARTESIAN_POINT('Ctrl Pts',(8.23201775036189,-1.09556604927598E-8,
-2.25));
#12838=CARTESIAN_POINT('Ctrl Pts',(8.23095406960136,-0.0076544365601514,
-2.24999999996273));
#12839=CARTESIAN_POINT('Ctrl Pts',(8.22989045929263,-0.0153097114686535,
-2.24996093978238));
#12840=CARTESIAN_POINT('Ctrl Pts',(8.20843948292972,-0.169726843614622,
-2.24838473640397));
#12841=CARTESIAN_POINT('Ctrl Pts',(8.18823199726517,-0.31599337566833,-2.23253050637012));
#12842=CARTESIAN_POINT('Ctrl Pts',(8.1271285281988,-0.748615648616462,-2.14224097734124));
#12843=CARTESIAN_POINT('Ctrl Pts',(8.08629749799337,-1.0228801106048,-2.02566911458184));
#12844=CARTESIAN_POINT('Ctrl Pts',(8.0250971071162,-1.38842278055941,-1.77663607139859));
#12845=CARTESIAN_POINT('Ctrl Pts',(8.00484078578692,-1.50161247962248,-1.68205612062705));
#12846=CARTESIAN_POINT('Ctrl Pts',(7.96407681040092,-1.70784894142048,-1.47220407654263));
#12847=CARTESIAN_POINT('Ctrl Pts',(7.94366318154694,-1.80040548235535,-1.3574496594755));
#12848=CARTESIAN_POINT('Ctrl Pts',(7.90275893934824,-1.96178295692203,-1.1115457126321));
#12849=CARTESIAN_POINT('Ctrl Pts',(7.88245441796761,-2.03022494603235,-0.980977885241562));
#12850=CARTESIAN_POINT('Ctrl Pts',(7.82209564580445,-2.19418014489188,-0.57617802840078));
#12851=CARTESIAN_POINT('Ctrl Pts',(7.7821116220244,-2.25005518612483,-0.289209643824882));
#12852=CARTESIAN_POINT('Ctrl Pts',(7.70176962959587,-2.24994473140811,0.290065825880358));
#12853=CARTESIAN_POINT('Ctrl Pts',(7.66222571526396,-2.1939641725135,0.576981779026868));
#12854=CARTESIAN_POINT('Ctrl Pts',(7.60148878147473,-2.02987896698876,0.981694164661813));
#12855=CARTESIAN_POINT('Ctrl Pts',(7.58108568810569,-1.96138190649418,1.11225820465269));
#12856=CARTESIAN_POINT('Ctrl Pts',(7.54041008390259,-1.79989146956541,1.35813095322165));
#12857=CARTESIAN_POINT('Ctrl Pts',(7.52015330548745,-1.70729815730867,1.47284083444354));
#12858=CARTESIAN_POINT('Ctrl Pts',(7.47936147180096,-1.50099590571904,1.68260671123367));
#12859=CARTESIAN_POINT('Ctrl Pts',(7.45892033505228,-1.38777117021646,1.77714454947763));
#12860=CARTESIAN_POINT('Ctrl Pts',(7.39743869110616,-1.0221381803978,2.02604453173824));
#12861=CARTESIAN_POINT('Ctrl Pts',(7.35722382091421,-0.747826936732087,
2.14251682117079));
#12862=CARTESIAN_POINT('Ctrl Pts',(7.29580379636594,-0.315165842380389,
2.23264766329073));
#12863=CARTESIAN_POINT('Ctrl Pts',(7.2753937296875,-0.168877708232943,2.24845032000289));
#12864=CARTESIAN_POINT('Ctrl Pts',(7.23479094383233,0.124330601794713,2.25132919560883));
#12865=CARTESIAN_POINT('Ctrl Pts',(7.21464034989432,0.270543380370812,2.23846999940466));
#12866=CARTESIAN_POINT('Ctrl Pts',(7.15363413279597,0.703613780870449,2.15730617596627));
#12867=CARTESIAN_POINT('Ctrl Pts',(7.11295667378843,0.979348546673183,2.04693042658809));
#12868=CARTESIAN_POINT('Ctrl Pts',(7.05191636363925,1.3496802322424,1.80626978190683));
#12869=CARTESIAN_POINT('Ctrl Pts',(7.03157968634747,1.46512920013272,1.71395460692825));
#12870=CARTESIAN_POINT('Ctrl Pts',(6.99072053963046,1.67589437825013,1.50846237224991));
#12871=CARTESIAN_POINT('Ctrl Pts',(6.97029321134451,1.77078252607677,1.39585435600291));
#12872=CARTESIAN_POINT('Ctrl Pts',(6.90940773937468,2.01930906556166,1.03440985658292));
#12873=CARTESIAN_POINT('Ctrl Pts',(6.86961463792993,2.13627918649898,0.764147494529221));
#12874=CARTESIAN_POINT('Ctrl Pts',(6.80860900574881,2.22969433797703,0.335503824874883));
#12875=CARTESIAN_POINT('Ctrl Pts',(6.78820517091419,2.24684601517249,0.189176178485125));
#12876=CARTESIAN_POINT('Ctrl Pts',(6.74755527979027,2.2523603923114,-0.104667548958869));
#12877=CARTESIAN_POINT('Ctrl Pts',(6.72732633127926,2.24072440354504,-0.251466613113482));
#12878=CARTESIAN_POINT('Ctrl Pts',(6.68655919917942,2.18894465508701,-0.541018176731977));
#12879=CARTESIAN_POINT('Ctrl Pts',(6.66611446468501,2.14886146155801,-0.683059901069027));
#12880=CARTESIAN_POINT('Ctrl Pts',(6.60452666954551,1.98739922685157,-1.09553434819301));
#12881=CARTESIAN_POINT('Ctrl Pts',(6.56423594252792,1.82636571910927,-1.34697496578364));
#12882=CARTESIAN_POINT('Ctrl Pts',(6.50275589222393,1.51955467963752,-1.66583170377288));
#12883=CARTESIAN_POINT('Ctrl Pts',(6.48234218945987,1.40768156186358,-1.76138492976101));
#12884=CARTESIAN_POINT('Ctrl Pts',(6.44174376210382,1.16733881115099,-1.92904463122872));
#12885=CARTESIAN_POINT('Ctrl Pts',(6.4216179974731,1.03950335999851,-2.00083155686855));
#12886=CARTESIAN_POINT('Ctrl Pts',(6.36061241652338,0.636038013123998,-2.17822651786486));
#12887=CARTESIAN_POINT('Ctrl Pts',(6.31988140189253,0.345803393089197,-2.24268577897185));
#12888=CARTESIAN_POINT('Ctrl Pts',(6.27680967342241,0.0342641567769058,
-2.24980437079299));
#12889=CARTESIAN_POINT('Ctrl Pts',(6.27444173288307,0.017130188862149,-2.25000000029274));
#12890=CARTESIAN_POINT('Ctrl Pts',(6.27207432050307,-3.84499440678469E-8,
-2.25));
#12891=CARTESIAN_POINT('',(6.46795384919627,-3.82950037302251E-6,2.25003768627347));
#12892=CARTESIAN_POINT('Ctrl Pts',(5.48792567952862,3.86792289516769E-8,
-2.25));
#12893=CARTESIAN_POINT('Ctrl Pts',(5.50590617826707,0.130104127504668,-2.24999999776341));
#12894=CARTESIAN_POINT('Ctrl Pts',(5.52386671666605,0.259991227284445,-2.23871534675092));
#12895=CARTESIAN_POINT('Ctrl Pts',(5.5623215461235,0.532967571307075,-2.19090076998503));
#12896=CARTESIAN_POINT('Ctrl Pts',(5.5827531292993,0.674901764174861,-2.15141977173756));
#12897=CARTESIAN_POINT('Ctrl Pts',(5.64385937703691,1.08526177954693,-1.99263166541714));
#12898=CARTESIAN_POINT('Ctrl Pts',(5.6838090820455,1.3352802359164,-1.83450228602105));
#12899=CARTESIAN_POINT('Ctrl Pts',(5.74497711019981,1.65455495546337,-1.53183750016682));
#12900=CARTESIAN_POINT('Ctrl Pts',(5.76538200189739,1.75101488004341,-1.42057375546334));
#12901=CARTESIAN_POINT('Ctrl Pts',(5.80601436392908,1.920793517681,-1.18093025336458));
#12902=CARTESIAN_POINT('Ctrl Pts',(5.82622104687486,1.99372061410875,-1.05314825661555));
#12903=CARTESIAN_POINT('Ctrl Pts',(5.86696784939671,2.11386037262269,-0.784725166469402));
#12904=CARTESIAN_POINT('Ctrl Pts',(5.8874149002506,2.16068733645426,-0.644690781704316));
#12905=CARTESIAN_POINT('Ctrl Pts',(5.94906233647854,2.25941540231167,-0.212518566495218));
#12906=CARTESIAN_POINT('Ctrl Pts',(5.98939655581076,2.26774916672706,0.0862507441290902));
#12907=CARTESIAN_POINT('Ctrl Pts',(6.05090464780758,2.19334764755515,0.52275335085135));
#12908=CARTESIAN_POINT('Ctrl Pts',(6.07132177608726,2.15458413299376,0.66469081131897));
#12909=CARTESIAN_POINT('Ctrl Pts',(6.11192401182039,2.05019102651987,0.938389433970038));
#12910=CARTESIAN_POINT('Ctrl Pts',(6.13203297821732,1.98492831099768,1.06954157773761));
#12911=CARTESIAN_POINT('Ctrl Pts',(6.19304134318137,1.75109161637569,1.44327040719888));
#12912=CARTESIAN_POINT('Ctrl Pts',(6.23381080480159,1.54720227886157,1.6599759870873));
#12913=CARTESIAN_POINT('Ctrl Pts',(6.29059691656243,1.21282720819533,1.89869343989598));
#12914=CARTESIAN_POINT('Ctrl Pts',(6.30661199780199,1.11323007755143,1.958750721318));
#12915=CARTESIAN_POINT('Ctrl Pts',(6.34688875432011,0.853380541848131,2.08919502043973));
#12916=CARTESIAN_POINT('Ctrl Pts',(6.37113166383439,0.688728795534948,2.14910266292007));
#12917=CARTESIAN_POINT('Ctrl Pts',(6.4196784236978,0.348821980273698,2.22965154308787));
#12918=CARTESIAN_POINT('Ctrl Pts',(6.44369758253354,0.174704179448234,2.25000115879057));
#12919=CARTESIAN_POINT('Ctrl Pts',(6.46787355864607,-1.49233260668402E-5,
2.24999999995051));
#12920=CARTESIAN_POINT('Ctrl Pts',(6.46784713536575,-1.86563614583413E-5,
2.24999999992265));
#12921=CARTESIAN_POINT('Ctrl Pts',(6.49211169406068,-0.174744534622054,
2.24999855114526));
#12922=CARTESIAN_POINT('Ctrl Pts',(6.51640089120071,-0.34888303436543,2.22964444352667));
#12923=CARTESIAN_POINT('Ctrl Pts',(6.56476837632269,-0.688887635955652,
2.14905765169502));
#12924=CARTESIAN_POINT('Ctrl Pts',(6.5887783135975,-0.853592650180886,2.08911305388841));
#12925=CARTESIAN_POINT('Ctrl Pts',(6.62910801303975,-1.11351736209021,1.9585901699099));
#12926=CARTESIAN_POINT('Ctrl Pts',(6.64524247698548,-1.21313997953028,1.89849573053106));
#12927=CARTESIAN_POINT('Ctrl Pts',(6.70239823256866,-1.54751144648411,1.65969019718443));
#12928=CARTESIAN_POINT('Ctrl Pts',(6.74258770509127,-1.7513776231923,1.44292970044513));
#12929=CARTESIAN_POINT('Ctrl Pts',(6.80379082558073,-1.98515165987259,1.06912675228319));
#12930=CARTESIAN_POINT('Ctrl Pts',(6.8241135176427,-2.05038733316381,0.937960852125335));
#12931=CARTESIAN_POINT('Ctrl Pts',(6.86476495051354,-2.15471745928448,0.664254512043225));
#12932=CARTESIAN_POINT('Ctrl Pts',(6.88495985747066,-2.19345058340818,0.522320281225319));
#12933=CARTESIAN_POINT('Ctrl Pts',(6.946198939737,-2.267760737065,0.0858375831489372));
#12934=CARTESIAN_POINT('Ctrl Pts',(6.98715144780304,-2.25937613503204,-0.212901376086072));
#12935=CARTESIAN_POINT('Ctrl Pts',(7.04845236832096,-2.16058234907065,-0.645045190820419));
#12936=CARTESIAN_POINT('Ctrl Pts',(7.06874014121938,-2.11373063311318,-0.785073539238702));
#12937=CARTESIAN_POINT('Ctrl Pts',(7.1095114842508,-1.99354283688225,-1.05348701234965));
#12938=CARTESIAN_POINT('Ctrl Pts',(7.12990040297153,-1.92058729590811,-1.18126617250044));
#12939=CARTESIAN_POINT('Ctrl Pts',(7.17072340625096,-1.75078172705965,-1.42085786500112));
#12940=CARTESIAN_POINT('Ctrl Pts',(7.19097291479663,-1.65431774828579,-1.53209351119021));
#12941=CARTESIAN_POINT('Ctrl Pts',(7.2517815103747,-1.33498987523482,-1.83471529856348));
#12942=CARTESIAN_POINT('Ctrl Pts',(7.29228785139571,-1.08493979810649,-1.99280583005406));
#12943=CARTESIAN_POINT('Ctrl Pts',(7.35323176978037,-0.674565692077119,
-2.1515249064064));
#12944=CARTESIAN_POINT('Ctrl Pts',(7.37345400866882,-0.532631214890633,
-2.19098221227881));
#12945=CARTESIAN_POINT('Ctrl Pts',(7.4118042875143,-0.259755662775317,-2.23873662484747));
#12946=CARTESIAN_POINT('Ctrl Pts',(7.42982873863646,-0.12998020594816,-2.25000000277498));
#12947=CARTESIAN_POINT('Ctrl Pts',(7.44790748751171,4.80358836735251E-8,
-2.25));
#12948=CARTESIAN_POINT('Origin',(-1.62,0.,0.));
#12949=CARTESIAN_POINT('',(10.1921554549285,-1.75510464272513E-10,-2.24999999965197));
#12950=CARTESIAN_POINT('',(9.40799129157889,6.73348500120871E-9,-2.25));
#12951=CARTESIAN_POINT('',(-1.62,2.75545529808154E-16,-2.25));
#12952=CARTESIAN_POINT('Ctrl Pts',(10.1921554554485,-2.47752686421965E-10,
-2.25));
#12953=CARTESIAN_POINT('Ctrl Pts',(10.1678791899995,-0.174810220022603,
-2.24999999998075));
#12954=CARTESIAN_POINT('Ctrl Pts',(10.1435797764755,-0.34902221205559,-2.22962921949452));
#12955=CARTESIAN_POINT('Ctrl Pts',(10.095204122033,-0.689077681658914,-2.14899483794996));
#12956=CARTESIAN_POINT('Ctrl Pts',(10.0711972764174,-0.853755667884177,
-2.08904449831867));
#12957=CARTESIAN_POINT('Ctrl Pts',(10.0308729101271,-1.1136365201982,-1.95852147570092));
#12958=CARTESIAN_POINT('Ctrl Pts',(10.0147406223479,-1.2132419895112,-1.89842956834442));
#12959=CARTESIAN_POINT('Ctrl Pts',(9.95758689262062,-1.54759049910711,-1.65961674556115));
#12960=CARTESIAN_POINT('Ctrl Pts',(9.91739730356014,-1.75144732661182,-1.44284539106328));
#12961=CARTESIAN_POINT('Ctrl Pts',(9.85619398933669,-1.98520348866504,-1.06903041048806));
#12962=CARTESIAN_POINT('Ctrl Pts',(9.8358713790699,-2.05043249207215,-0.937862015186465));
#12963=CARTESIAN_POINT('Ctrl Pts',(9.7952201380992,-2.15474929967526,-0.664151245701674));
#12964=CARTESIAN_POINT('Ctrl Pts',(9.77502523258085,-2.19347565022966,-0.522215036382986));
#12965=CARTESIAN_POINT('Ctrl Pts',(9.71378588818094,-2.26776507549231,-0.0857273735488627));
#12966=CARTESIAN_POINT('Ctrl Pts',(9.67283320177061,-2.25936583118408,0.213012518120693));
#12967=CARTESIAN_POINT('Ctrl Pts',(9.6115321201354,-2.16055016212059,0.645153081928275));
#12968=CARTESIAN_POINT('Ctrl Pts',(9.59124426332106,-2.11369131603536,0.785179461201588));
#12969=CARTESIAN_POINT('Ctrl Pts',(9.55047290627762,-1.99349018446163,1.05358653325004));
#12970=CARTESIAN_POINT('Ctrl Pts',(9.53008405908172,-1.92052867295727,1.1813613845873));
#12971=CARTESIAN_POINT('Ctrl Pts',(9.48926126915408,-1.75071196702641,1.42094378060002));
#12972=CARTESIAN_POINT('Ctrl Pts',(9.46901188280145,-1.65424278622536,1.53217441317964));
#12973=CARTESIAN_POINT('Ctrl Pts',(9.4082024071065,-1.33489569641816,1.83478486492308));
#12974=CARTESIAN_POINT('Ctrl Pts',(9.36769505770934,-1.08483155590647,1.99286572080852));
#12975=CARTESIAN_POINT('Ctrl Pts',(9.30675034762537,-0.674441843775681,
2.15156376045152));
#12976=CARTESIAN_POINT('Ctrl Pts',(9.28652803966901,-0.532504701513786,
2.19101299057692));
#12977=CARTESIAN_POINT('Ctrl Pts',(9.24577859847646,-0.242555833700009,
2.24173799978252));
#12978=CARTESIAN_POINT('Ctrl Pts',(9.22534478964992,-0.0952368412224312,
2.25280901643769));
#12979=CARTESIAN_POINT('Ctrl Pts',(9.16388168375656,0.346512072377135,2.24257817668726));
#12980=CARTESIAN_POINT('Ctrl Pts',(9.12370981787615,0.636751562346658,2.17802255503517));
#12981=CARTESIAN_POINT('Ctrl Pts',(9.06253692001376,1.04018689981432,2.00047628757521));
#12982=CARTESIAN_POINT('Ctrl Pts',(9.04220047461225,1.16799944579107,1.92864475338737));
#12983=CARTESIAN_POINT('Ctrl Pts',(9.00151599147505,1.40826799044789,1.76091434507733));
#12984=CARTESIAN_POINT('Ctrl Pts',(8.98131820618637,1.52010023448917,1.66533364131775));
#12985=CARTESIAN_POINT('Ctrl Pts',(8.92012969082443,1.82679201010891,1.34639257552805));
#12986=CARTESIAN_POINT('Ctrl Pts',(8.87921761889866,1.98773701141072,1.09491684581422));
#12987=CARTESIAN_POINT('Ctrl Pts',(8.81795113408565,2.14907186905657,0.682399770891608));
#12988=CARTESIAN_POINT('Ctrl Pts',(8.79767747867094,2.18911090908818,0.540343841329279));
#12989=CARTESIAN_POINT('Ctrl Pts',(8.7569088565767,2.24080424176858,0.250764149690147));
#12990=CARTESIAN_POINT('Ctrl Pts',(8.73650826454768,2.25239375654172,0.103950537859746));
#12991=CARTESIAN_POINT('Ctrl Pts',(8.6956490127593,2.24678613485836,-0.189859246691785));
#12992=CARTESIAN_POINT('Ctrl Pts',(8.67537704616007,2.22959509548118,-0.33616143559126));
#12993=CARTESIAN_POINT('Ctrl Pts',(8.61473755750295,2.13604416922574,-0.764823027594284));
#12994=CARTESIAN_POINT('Ctrl Pts',(8.57442654317558,2.01896537293113,-1.03508735577817));
#12995=CARTESIAN_POINT('Ctrl Pts',(8.51363594566775,1.77030394547916,-1.39646058182148));
#12996=CARTESIAN_POINT('Ctrl Pts',(8.49342486634409,1.67538186709516,-1.50903122743432));
#12997=CARTESIAN_POINT('Ctrl Pts',(8.45268269369654,1.46453027254645,-1.71446874901185));
#12998=CARTESIAN_POINT('Ctrl Pts',(8.43224469130559,1.34903583430484,-1.80675124475737));
#12999=CARTESIAN_POINT('Ctrl Pts',(8.37080918781604,0.978609634814664,-2.04728501279938));
#13000=CARTESIAN_POINT('Ctrl Pts',(8.33065545347321,0.70281436392203,-2.15757114052607));
#13001=CARTESIAN_POINT('Ctrl Pts',(8.27058336091969,0.277203037255173,-2.23716731953718));
#13002=CARTESIAN_POINT('Ctrl Pts',(8.25129743618393,0.13873984998652,-2.25000000067555));
#13003=CARTESIAN_POINT('Ctrl Pts',(8.23201775036189,-1.0955660406653E-8,
-2.25));
#13004=CARTESIAN_POINT('Ctrl Pts',(7.44790748751171,4.80358838146612E-8,
-2.25));
#13005=CARTESIAN_POINT('Ctrl Pts',(7.45031648143266,0.0173199214325949,
-2.24999999963023));
#13006=CARTESIAN_POINT('Ctrl Pts',(7.45272621823156,0.0346434618927655,
-2.24980001423445));
#13007=CARTESIAN_POINT('Ctrl Pts',(7.49610020567124,0.346382258987719,-2.24259800182962));
#13008=CARTESIAN_POINT('Ctrl Pts',(7.53627195156904,0.636623768696126,-2.17805967758632));
#13009=CARTESIAN_POINT('Ctrl Pts',(7.59744462210005,1.04006892373761,-2.00053769562103));
#13010=CARTESIAN_POINT('Ctrl Pts',(7.61778116825911,1.16788650756399,-1.92871321508005));
#13011=CARTESIAN_POINT('Ctrl Pts',(7.65846589394708,1.40816555054601,-1.7609962636005));
#13012=CARTESIAN_POINT('Ctrl Pts',(7.67866371491907,1.52000334029545,-1.6654220791355));
#13013=CARTESIAN_POINT('Ctrl Pts',(7.73985181636063,1.82671196060705,-1.34650064035097));
#13014=CARTESIAN_POINT('Ctrl Pts',(7.78076352791346,1.98767063308841,-1.09503667312279));
#13015=CARTESIAN_POINT('Ctrl Pts',(7.84202971159407,2.1490297547269,-0.682532279891398));
#13016=CARTESIAN_POINT('Ctrl Pts',(7.86230326647522,2.18907743671087,-0.540479298917099));
#13017=CARTESIAN_POINT('Ctrl Pts',(7.90307186576371,2.2407888284488,-0.250902384702513));
#13018=CARTESIAN_POINT('Ctrl Pts',(7.9234725375215,2.25238744205827,-0.104088562540999));
#13019=CARTESIAN_POINT('Ctrl Pts',(7.96433204816676,2.24679767729886,0.189723036676631));
#13020=CARTESIAN_POINT('Ctrl Pts',(7.98460418730738,2.2296154234309,0.336026829898549));
#13021=CARTESIAN_POINT('Ctrl Pts',(8.04524231046848,2.13609233716781,0.764684572234052));
#13022=CARTESIAN_POINT('Ctrl Pts',(8.08555173910438,2.01903581037218,1.03494704876394));
#13023=CARTESIAN_POINT('Ctrl Pts',(8.14634109124253,1.77040713033635,1.39632971307185));
#13024=CARTESIAN_POINT('Ctrl Pts',(8.1665520950889,1.67549369138675,1.50890702160853));
#13025=CARTESIAN_POINT('Ctrl Pts',(8.20729421227161,1.46465721787459,1.71436035966986));
#13026=CARTESIAN_POINT('Ctrl Pts',(8.22773223624926,1.34916907133738,1.80665180832173));
#13027=CARTESIAN_POINT('Ctrl Pts',(8.2891675313845,0.978761724240049,2.04721200714371));
#13028=CARTESIAN_POINT('Ctrl Pts',(8.32932115704057,0.702976682237688,2.1575179774717));
#13029=CARTESIAN_POINT('Ctrl Pts',(8.39045522386414,0.269846343520668,2.23855448139628));
#13030=CARTESIAN_POINT('Ctrl Pts',(8.41080931861443,0.123624641426579,2.25136818007742));
#13031=CARTESIAN_POINT('Ctrl Pts',(8.45153730418538,-0.169559396633769,
2.24839738195556));
#13032=CARTESIAN_POINT('Ctrl Pts',(8.47174488559542,-0.315827288333582,
2.2325540203774));
#13033=CARTESIAN_POINT('Ctrl Pts',(8.53284763191817,-0.748451709252293,
2.14229759214995));
#13034=CARTESIAN_POINT('Ctrl Pts',(8.57367792823207,-1.02272061053316,2.02574893780776));
#13035=CARTESIAN_POINT('Ctrl Pts',(8.6348777298969,-1.38827882269214,1.77674851017548));
#13036=CARTESIAN_POINT('Ctrl Pts',(8.65513392693521,-1.50147570510363,1.68217815750605));
#13037=CARTESIAN_POINT('Ctrl Pts',(8.69589786344588,-1.7077296333102,1.47234258268137));
#13038=CARTESIAN_POINT('Ctrl Pts',(8.71631158024835,-1.80029615758694,1.35759476745783));
#13039=CARTESIAN_POINT('Ctrl Pts',(8.75721614760918,-1.96169440977718,1.11170209019017));
#13040=CARTESIAN_POINT('Ctrl Pts',(8.77752092322055,-2.03014718659409,0.981138929748954));
#13041=CARTESIAN_POINT('Ctrl Pts',(8.83787729354608,-2.1941278449513,0.576368034708614));
#13042=CARTESIAN_POINT('Ctrl Pts',(8.87785851684834,-2.25002540127477,0.289423038532547));
#13043=CARTESIAN_POINT('Ctrl Pts',(8.95819769845474,-2.24997458026347,-0.28982835325914));
#13044=CARTESIAN_POINT('Ctrl Pts',(8.99774051748962,-2.19402582019354,-0.576744396851616));
#13045=CARTESIAN_POINT('Ctrl Pts',(9.05847639803951,-2.0299880375715,-0.981468421122089));
#13046=CARTESIAN_POINT('Ctrl Pts',(9.07887949691193,-1.96150610301751,-1.11203900272667));
#13047=CARTESIAN_POINT('Ctrl Pts',(9.11955481998493,-1.80004480754295,-1.35792754524089));
#13048=CARTESIAN_POINT('Ctrl Pts',(9.13981131485071,-1.7074654810793,-1.47264669790595));
#13049=CARTESIAN_POINT('Ctrl Pts',(9.18060290038066,-1.50118768514118,-1.68243568893175));
#13050=CARTESIAN_POINT('Ctrl Pts',(9.20104407724762,-1.38797303087011,-1.77698696975314));
#13051=CARTESIAN_POINT('Ctrl Pts',(9.26252700148927,-1.022361801345,-2.02593270437716));
#13052=CARTESIAN_POINT('Ctrl Pts',(9.30274277999797,-0.748056668585006,
-2.14243757513772));
#13053=CARTESIAN_POINT('Ctrl Pts',(9.36416357607854,-0.315398432957757,
-2.23261480086537));
#13054=CARTESIAN_POINT('Ctrl Pts',(9.38457367646151,-0.169112221404442,
-2.24843267511704));
#13055=CARTESIAN_POINT('Ctrl Pts',(9.40593108173522,-0.0148830980846057,
-2.2499630862436));
#13056=CARTESIAN_POINT('Ctrl Pts',(9.4069613454312,-0.00744114014909166,
-2.25000000004454));
#13057=CARTESIAN_POINT('Ctrl Pts',(9.40799129157889,1.34669676642552E-8,
-2.25));
#13058=CARTESIAN_POINT('Origin',(0.,0.,-1.75));
#13059=CARTESIAN_POINT('',(0.734986525864679,1.12279801474381E-10,-3.12449703104719));
#13060=CARTESIAN_POINT('Ctrl Pts',(0.734986525570974,8.83388398624539E-17,
-3.12449703116234));
#13061=CARTESIAN_POINT('Ctrl Pts',(0.677869456040291,-1.78307850476143E-14,
-2.97881367266937));
#13062=CARTESIAN_POINT('Ctrl Pts',(0.620752386509192,-4.29751012965632E-12,
-2.83313031417656));
#13063=CARTESIAN_POINT('Ctrl Pts',(0.5064663800335,-4.29751012965632E-12,
-2.54163130365447));
#13064=CARTESIAN_POINT('Ctrl Pts',(0.449297443089002,-3.51393138104219E-15,
-2.39581565162515));
#13065=CARTESIAN_POINT('Ctrl Pts',(0.392128506144054,-1.42854491361204E-16,
-2.24999999959601));
#13066=CARTESIAN_POINT('',(0.98,1.07231970108979E-7,-3.12449703081926));
#13067=CARTESIAN_POINT('Ctrl Pts',(0.98,1.38777878078145E-16,-3.12449703075067));
#13068=CARTESIAN_POINT('Ctrl Pts',(0.939166666666667,1.38777878078145E-16,
-3.12449703075067));
#13069=CARTESIAN_POINT('Ctrl Pts',(0.898333333333334,1.38777878078145E-16,
-3.12449703075067));
#13070=CARTESIAN_POINT('Ctrl Pts',(0.816662175288226,1.38777878078145E-16,
-3.12449703075067));
#13071=CARTESIAN_POINT('Ctrl Pts',(0.775824350576453,1.38777878078145E-16,
-3.12449703075067));
#13072=CARTESIAN_POINT('Ctrl Pts',(0.734986525864679,1.38777878078145E-16,
-3.12449703075067));
#13073=CARTESIAN_POINT('',(1.22498652499198,-1.0227729590452E-10,-3.1244970310227));
#13074=CARTESIAN_POINT('Ctrl Pts',(1.22498652499198,-1.38762734240172E-16,
-3.12449703075067));
#13075=CARTESIAN_POINT('Ctrl Pts',(1.18415768332799,-1.36412213158615E-16,
-3.12449703075067));
#13076=CARTESIAN_POINT('Ctrl Pts',(1.14332884166399,1.38777878078145E-16,
-3.12449703075067));
#13077=CARTESIAN_POINT('Ctrl Pts',(1.06166666666667,1.38777878078145E-16,
-3.12449703075067));
#13078=CARTESIAN_POINT('Ctrl Pts',(1.02083333333333,1.38777878078145E-16,
-3.12449703075067));
#13079=CARTESIAN_POINT('Ctrl Pts',(0.98,1.38777878078145E-16,-3.12449703075067));
#13080=CARTESIAN_POINT('Ctrl Pts',(1.56784454470915,-9.35700253971563E-17,
-2.24999999950992));
#13081=CARTESIAN_POINT('Ctrl Pts',(1.51067680443466,5.09067919699466E-15,
-2.39581259929919));
#13082=CARTESIAN_POINT('Ctrl Pts',(1.45350906416085,5.51601214575205E-12,
-2.54162519908873));
#13083=CARTESIAN_POINT('Ctrl Pts',(1.33922305767831,5.51601214575205E-12,
-2.83312420962822));
#13084=CARTESIAN_POINT('Ctrl Pts',(1.2821047914697,2.2886891001175E-14,
-2.97881062037821));
#13085=CARTESIAN_POINT('Ctrl Pts',(1.22498652526162,1.11438500184582E-16,
-3.12449703112841));
#13086=CARTESIAN_POINT('Origin',(-1.62,0.,0.));
#13087=CARTESIAN_POINT('',(11.3678714941529,1.44267579994225E-10,-2.24999999971305));
#13088=CARTESIAN_POINT('Ctrl Pts',(9.40799129157889,1.34669670553977E-8,
-2.25));
#13089=CARTESIAN_POINT('Ctrl Pts',(9.42722393706556,0.138952006083732,-2.24999999916833));
#13090=CARTESIAN_POINT('Ctrl Pts',(9.44635724963363,0.277621957227089,-2.23712827275445));
#13091=CARTESIAN_POINT('Ctrl Pts',(9.50633290109874,0.703386470993788,-2.15738069016551));
#13092=CARTESIAN_POINT('Ctrl Pts',(9.54701090703894,0.979135514210064,-2.04703274565594));
#13093=CARTESIAN_POINT('Ctrl Pts',(9.60805151839805,1.34949355615953,-1.80640917823359));
#13094=CARTESIAN_POINT('Ctrl Pts',(9.62838798253185,1.46495134723679,-1.71410654406964));
#13095=CARTESIAN_POINT('Ctrl Pts',(9.66924695654409,1.67573773164555,-1.50863645153028));
#13096=CARTESIAN_POINT('Ctrl Pts',(9.68967432809396,1.7706379741301,-1.39603778183696));
#13097=CARTESIAN_POINT('Ctrl Pts',(9.75056224243817,2.0192104430276,-1.03460645757018));
#13098=CARTESIAN_POINT('Ctrl Pts',(9.79035708141066,2.13621182393407,-0.764341340201784));
#13099=CARTESIAN_POINT('Ctrl Pts',(9.85136454776663,2.22966594882906,-0.335692092866465));
#13100=CARTESIAN_POINT('Ctrl Pts',(9.87176839065577,2.2468299138393,-0.189366695491866));
#13101=CARTESIAN_POINT('Ctrl Pts',(9.91241809383145,2.25236927240188,0.104474480257507));
#13102=CARTESIAN_POINT('Ctrl Pts',(9.93264682154377,2.24074601056064,0.251273266333001));
#13103=CARTESIAN_POINT('Ctrl Pts',(9.97341375475298,2.1889915116435,0.540828745288069));
#13104=CARTESIAN_POINT('Ctrl Pts',(9.99385851491314,2.14892040621718,0.682874580613988));
#13105=CARTESIAN_POINT('Ctrl Pts',(10.0554470055626,1.98749210778212,1.09536678146656));
#13106=CARTESIAN_POINT('Ctrl Pts',(10.0957382363584,1.82647768514058,1.34682391057384));
#13107=CARTESIAN_POINT('Ctrl Pts',(10.1572186460484,1.51969012003666,1.66570814817095));
#13108=CARTESIAN_POINT('Ctrl Pts',(10.1776323800607,1.40782476558684,1.7612704727696));
#13109=CARTESIAN_POINT('Ctrl Pts',(10.2182308009482,1.16749670769175,1.92894897553718));
#13110=CARTESIAN_POINT('Ctrl Pts',(10.2383563750675,1.03966827773101,2.00074577480369));
#13111=CARTESIAN_POINT('Ctrl Pts',(10.2993619682263,0.636216616771537,2.17817468325712));
#13112=CARTESIAN_POINT('Ctrl Pts',(10.3400934024976,0.34598484018812,2.24265810772764));
#13113=CARTESIAN_POINT('Ctrl Pts',(10.4011657134897,-0.0957520143723365,
2.25278696900762));
#13114=CARTESIAN_POINT('Ctrl Pts',(10.4214805305554,-0.243052612565244,
2.24168242290984));
#13115=CARTESIAN_POINT('Ctrl Pts',(10.4623217669302,-0.532969117421723,
2.19090039354356));
#13116=CARTESIAN_POINT('Ctrl Pts',(10.4827533498151,-0.674903277826521,
2.15141929658051));
#13117=CARTESIAN_POINT('Ctrl Pts',(10.5438595837323,-1.08526310221882,1.99263093318505));
#13118=CARTESIAN_POINT('Ctrl Pts',(10.5838092789636,-1.33528138597463,1.83450143603576));
#13119=CARTESIAN_POINT('Ctrl Pts',(10.6449772971943,-1.65455587022264,1.53183651256687));
#13120=CARTESIAN_POINT('Ctrl Pts',(10.6653821888002,-1.75101573134227,1.42057270662821));
#13121=CARTESIAN_POINT('Ctrl Pts',(10.7060145519656,-1.92079423307653,1.18092909093811));
#13122=CARTESIAN_POINT('Ctrl Pts',(10.7262212364816,-1.99372125655518,1.05314704169378));
#13123=CARTESIAN_POINT('Ctrl Pts',(10.7669680404543,-2.11386085222904,0.784723873637474));
#13124=CARTESIAN_POINT('Ctrl Pts',(10.7874150911621,-2.16068772907889,0.644689464755181));
#13125=CARTESIAN_POINT('Ctrl Pts',(10.8490625238631,-2.25941552779656,0.212517209869512));
#13126=CARTESIAN_POINT('Ctrl Pts',(10.8893967405326,-2.26774911344673,-0.0862520889962616));
#13127=CARTESIAN_POINT('Ctrl Pts',(10.9509048310764,-2.19334734149575,-0.522754634588145));
#13128=CARTESIAN_POINT('Ctrl Pts',(10.9713219591151,-2.1545837442751,-0.664692071066582));
#13129=CARTESIAN_POINT('Ctrl Pts',(11.01192419454,-2.05019047522867,-0.938390639800923));
#13130=CARTESIAN_POINT('Ctrl Pts',(11.032033162198,-1.98492767839981,-1.06954275294056));
#13131=CARTESIAN_POINT('Ctrl Pts',(11.093041526889,-1.75109076592916,-1.44327143540629));
#13132=CARTESIAN_POINT('Ctrl Pts',(11.1338109856041,-1.54720131430671,-1.65997688298466));
#13133=CARTESIAN_POINT('Ctrl Pts',(11.190594802108,-1.21283961938079,-1.89868449761896));
#13134=CARTESIAN_POINT('Ctrl Pts',(11.2066076031856,-1.11325738277325,-1.95873421942164));
#13135=CARTESIAN_POINT('Ctrl Pts',(11.2468785862839,-0.853447715989413,
-2.08916550010555));
#13136=CARTESIAN_POINT('Ctrl Pts',(11.2711180082559,-0.688821878776564,
-2.14907080760077));
#13137=CARTESIAN_POINT('Ctrl Pts',(11.3196668465811,-0.348905567752826,
-2.22964153417314));
#13138=CARTESIAN_POINT('Ctrl Pts',(11.3436900377268,-0.174758732835044,
-2.25000000001581));
#13139=CARTESIAN_POINT('Ctrl Pts',(11.3678714937241,2.03596479952939E-10,
-2.25));
#13140=CARTESIAN_POINT('',(32.48,0.,-2.25));
#13141=CARTESIAN_POINT('',(-1.62,2.75545529808154E-16,-2.25));
#13142=CARTESIAN_POINT('Origin',(32.48,0.,0.));
#13143=CARTESIAN_POINT('',(10.192,0.,-2.25));
#13144=CARTESIAN_POINT('Ctrl Pts',(1.486050567538,-0.6826354359695,-2.100935843176));
#13145=CARTESIAN_POINT('Ctrl Pts',(1.539133900872,-0.3251200195628,-2.217099643673));
#13146=CARTESIAN_POINT('Ctrl Pts',(1.645300567538,0.4500302339061,-2.2627584625));
#13147=CARTESIAN_POINT('Ctrl Pts',(1.804550567538,1.498365337642,-1.754345766741));
#13148=CARTESIAN_POINT('Ctrl Pts',(1.963800567538,2.164505898152,-0.7985285881669));
#13149=CARTESIAN_POINT('Ctrl Pts',(2.123050567538,2.278706807749,0.3609111019353));
#13150=CARTESIAN_POINT('Ctrl Pts',(2.282300567538,1.811812146172,1.428317898065));
#13151=CARTESIAN_POINT('Ctrl Pts',(2.441550567538,0.8828928310149,2.13149160242));
#13152=CARTESIAN_POINT('Ctrl Pts',(2.600800567538,-0.271171719174,2.291118092888));
#13153=CARTESIAN_POINT('Ctrl Pts',(2.760050567538,-1.35608517812,1.866491128517));
#13154=CARTESIAN_POINT('Ctrl Pts',(2.919300567538,-2.09518612394,0.9658940328033));
#13155=CARTESIAN_POINT('Ctrl Pts',(3.078550567538,-2.299997866445,-0.1810137579678));
#13156=CARTESIAN_POINT('Ctrl Pts',(3.237800567538,-1.918291788201,-1.281761594049));
#13157=CARTESIAN_POINT('Ctrl Pts',(3.397050567538,-1.047405984058,-2.055649987917));
#13158=CARTESIAN_POINT('Ctrl Pts',(3.556300567538,0.09057671026141,-2.305331218682));
#13159=CARTESIAN_POINT('Ctrl Pts',(3.715550567538,1.205461620183,-1.967134578661));
#13160=CARTESIAN_POINT('Ctrl Pts',(3.874800567538,2.012944190303,-1.127302911826));
#13161=CARTESIAN_POINT('Ctrl Pts',(4.034050567538,2.30710991682,0.));
#13162=CARTESIAN_POINT('Ctrl Pts',(4.193300567538,2.012944190303,1.127302911826));
#13163=CARTESIAN_POINT('Ctrl Pts',(4.352550567538,1.205461620183,1.967134578661));
#13164=CARTESIAN_POINT('Ctrl Pts',(4.511800567538,0.09057671026142,2.305331218682));
#13165=CARTESIAN_POINT('Ctrl Pts',(4.671050567538,-1.047405984058,2.055649987917));
#13166=CARTESIAN_POINT('Ctrl Pts',(4.830300567538,-1.918291788201,1.281761594049));
#13167=CARTESIAN_POINT('Ctrl Pts',(4.989550567538,-2.299997866445,0.1810137579678));
#13168=CARTESIAN_POINT('Ctrl Pts',(5.148800567538,-2.09518612394,-0.9658940328033));
#13169=CARTESIAN_POINT('Ctrl Pts',(5.308050567538,-1.35608517812,-1.866491128517));
#13170=CARTESIAN_POINT('Ctrl Pts',(5.467300567538,-0.271171719174,-2.291118092888));
#13171=CARTESIAN_POINT('Ctrl Pts',(5.626550567538,0.8828928310149,-2.13149160242));
#13172=CARTESIAN_POINT('Ctrl Pts',(5.785800567538,1.811812146172,-1.428317898065));
#13173=CARTESIAN_POINT('Ctrl Pts',(5.945050567538,2.278706807749,-0.3609111019352));
#13174=CARTESIAN_POINT('Ctrl Pts',(6.104300567538,2.164505898152,0.7985285881669));
#13175=CARTESIAN_POINT('Ctrl Pts',(6.263550567538,1.498365337642,1.754345766741));
#13176=CARTESIAN_POINT('Ctrl Pts',(6.422800567538,0.4500302339061,2.2627584625));
#13177=CARTESIAN_POINT('Ctrl Pts',(6.528967234205,-0.3251200195628,2.217099643673));
#13178=CARTESIAN_POINT('Ctrl Pts',(6.582050567538,-0.6826354359695,2.100935843176));
#13179=CARTESIAN_POINT('Ctrl Pts',(1.361016855846,-0.7812005935783,-2.404288206087));
#13180=CARTESIAN_POINT('Ctrl Pts',(1.414100189179,-0.3720638262881,-2.537224800233));
#13181=CARTESIAN_POINT('Ctrl Pts',(1.520266855846,0.5150097216332,-2.589476257585));
#13182=CARTESIAN_POINT('Ctrl Pts',(1.679516855846,1.714713051046,-2.007654279437));
#13183=CARTESIAN_POINT('Ctrl Pts',(1.838766855846,2.477037087943,-0.9138274607431));
#13184=CARTESIAN_POINT('Ctrl Pts',(1.998016855846,2.607727371018,0.413022753002));
#13185=CARTESIAN_POINT('Ctrl Pts',(2.157266855846,2.073418181158,1.634551520464));
#13186=CARTESIAN_POINT('Ctrl Pts',(2.316516855846,1.010372985802,2.439255885761));
#13187=CARTESIAN_POINT('Ctrl Pts',(2.475766855846,-0.3103259760893,2.6219307112));
#13188=CARTESIAN_POINT('Ctrl Pts',(2.635016855846,-1.551889178717,2.135992215868));
#13189=CARTESIAN_POINT('Ctrl Pts',(2.794266855846,-2.397708289717,1.105358661447));
#13190=CARTESIAN_POINT('Ctrl Pts',(2.953516855846,-2.632092627808,-0.2071501825414));
#13191=CARTESIAN_POINT('Ctrl Pts',(3.112766855846,-2.195272329322,-1.466834074728));
#13192=CARTESIAN_POINT('Ctrl Pts',(3.272016855846,-1.198640054924,-2.3524635642));
#13193=CARTESIAN_POINT('Ctrl Pts',(3.431266855846,0.1036550054277,-2.638196058298));
#13194=CARTESIAN_POINT('Ctrl Pts',(3.590516855846,1.37951721168,-2.251167489299));
#13195=CARTESIAN_POINT('Ctrl Pts',(3.749766855846,2.303591512314,-1.290073233029));
#13196=CARTESIAN_POINT('Ctrl Pts',(3.909016855846,2.640231581167,0.));
#13197=CARTESIAN_POINT('Ctrl Pts',(4.068266855846,2.303591512314,1.290073233029));
#13198=CARTESIAN_POINT('Ctrl Pts',(4.227516855846,1.37951721168,2.251167489299));
#13199=CARTESIAN_POINT('Ctrl Pts',(4.386766855846,0.1036550054277,2.638196058298));
#13200=CARTESIAN_POINT('Ctrl Pts',(4.546016855846,-1.198640054924,2.3524635642));
#13201=CARTESIAN_POINT('Ctrl Pts',(4.705266855846,-2.195272329322,1.466834074728));
#13202=CARTESIAN_POINT('Ctrl Pts',(4.864516855846,-2.632092627808,0.2071501825414));
#13203=CARTESIAN_POINT('Ctrl Pts',(5.023766855846,-2.397708289717,-1.105358661447));
#13204=CARTESIAN_POINT('Ctrl Pts',(5.183016855846,-1.551889178717,-2.135992215868));
#13205=CARTESIAN_POINT('Ctrl Pts',(5.342266855846,-0.3103259760893,-2.6219307112));
#13206=CARTESIAN_POINT('Ctrl Pts',(5.501516855846,1.010372985802,-2.439255885761));
#13207=CARTESIAN_POINT('Ctrl Pts',(5.660766855846,2.073418181158,-1.634551520464));
#13208=CARTESIAN_POINT('Ctrl Pts',(5.820016855846,2.607727371018,-0.4130227530019));
#13209=CARTESIAN_POINT('Ctrl Pts',(5.979266855846,2.477037087943,0.913827460743));
#13210=CARTESIAN_POINT('Ctrl Pts',(6.138516855846,1.714713051046,2.007654279437));
#13211=CARTESIAN_POINT('Ctrl Pts',(6.297766855846,0.5150097216332,2.589476257585));
#13212=CARTESIAN_POINT('Ctrl Pts',(6.403933522513,-0.3720638262881,2.537224800233));
#13213=CARTESIAN_POINT('Ctrl Pts',(6.457016855846,-0.7812005935783,2.404288206087));
#13214=CARTESIAN_POINT('Ctrl Pts',(1.235983144154,-0.8797657511871,-2.707640568999));
#13215=CARTESIAN_POINT('Ctrl Pts',(1.289066477487,-0.4190076330134,-2.857349956793));
#13216=CARTESIAN_POINT('Ctrl Pts',(1.395233144154,0.5799892093603,-2.91619405267));
#13217=CARTESIAN_POINT('Ctrl Pts',(1.554483144154,1.931060764449,-2.260962792133));
#13218=CARTESIAN_POINT('Ctrl Pts',(1.713733144154,2.789568277733,-1.029126333319));
#13219=CARTESIAN_POINT('Ctrl Pts',(1.872983144154,2.936747934286,0.4651344040687));
#13220=CARTESIAN_POINT('Ctrl Pts',(2.032233144154,2.335024216144,1.840785142863));
#13221=CARTESIAN_POINT('Ctrl Pts',(2.191483144154,1.137853140589,2.747020169102));
#13222=CARTESIAN_POINT('Ctrl Pts',(2.350733144154,-0.3494802330045,2.952743329512));
#13223=CARTESIAN_POINT('Ctrl Pts',(2.509983144154,-1.747693179314,2.405493303218));
#13224=CARTESIAN_POINT('Ctrl Pts',(2.669233144154,-2.700230455495,1.244823290091));
#13225=CARTESIAN_POINT('Ctrl Pts',(2.828483144154,-2.964187389171,-0.2332866071149));
#13226=CARTESIAN_POINT('Ctrl Pts',(2.987733144154,-2.472252870444,-1.651906555408));
#13227=CARTESIAN_POINT('Ctrl Pts',(3.146983144154,-1.34987412579,-2.649277140482));
#13228=CARTESIAN_POINT('Ctrl Pts',(3.306233144154,0.1167333005941,-2.971060897913));
#13229=CARTESIAN_POINT('Ctrl Pts',(3.465483144154,1.553572803177,-2.535200399938));
#13230=CARTESIAN_POINT('Ctrl Pts',(3.624733144154,2.594238834326,-1.452843554231));
#13231=CARTESIAN_POINT('Ctrl Pts',(3.783983144154,2.973353245513,0.));
#13232=CARTESIAN_POINT('Ctrl Pts',(3.943233144154,2.594238834326,1.452843554231));
#13233=CARTESIAN_POINT('Ctrl Pts',(4.102483144154,1.553572803177,2.535200399938));
#13234=CARTESIAN_POINT('Ctrl Pts',(4.261733144154,0.1167333005941,2.971060897913));
#13235=CARTESIAN_POINT('Ctrl Pts',(4.420983144154,-1.34987412579,2.649277140482));
#13236=CARTESIAN_POINT('Ctrl Pts',(4.580233144154,-2.472252870444,1.651906555408));
#13237=CARTESIAN_POINT('Ctrl Pts',(4.739483144154,-2.964187389171,0.2332866071149));
#13238=CARTESIAN_POINT('Ctrl Pts',(4.898733144154,-2.700230455495,-1.244823290091));
#13239=CARTESIAN_POINT('Ctrl Pts',(5.057983144154,-1.747693179314,-2.405493303218));
#13240=CARTESIAN_POINT('Ctrl Pts',(5.217233144154,-0.3494802330045,-2.952743329512));
#13241=CARTESIAN_POINT('Ctrl Pts',(5.376483144154,1.137853140589,-2.747020169102));
#13242=CARTESIAN_POINT('Ctrl Pts',(5.535733144154,2.335024216144,-1.840785142863));
#13243=CARTESIAN_POINT('Ctrl Pts',(5.694983144154,2.936747934286,-0.4651344040687));
#13244=CARTESIAN_POINT('Ctrl Pts',(5.854233144154,2.789568277733,1.029126333319));
#13245=CARTESIAN_POINT('Ctrl Pts',(6.013483144154,1.931060764449,2.260962792133));
#13246=CARTESIAN_POINT('Ctrl Pts',(6.172733144154,0.5799892093604,2.91619405267));
#13247=CARTESIAN_POINT('Ctrl Pts',(6.278899810821,-0.4190076330134,2.857349956793));
#13248=CARTESIAN_POINT('Ctrl Pts',(6.331983144154,-0.8797657511871,2.707640568999));
#13249=CARTESIAN_POINT('Ctrl Pts',(1.110949432462,-0.9783309087958,-3.010992931911));
#13250=CARTESIAN_POINT('Ctrl Pts',(1.164032765795,-0.4659514397387,-3.177475113353));
#13251=CARTESIAN_POINT('Ctrl Pts',(1.270199432462,0.6449686970875,-3.242911847755));
#13252=CARTESIAN_POINT('Ctrl Pts',(1.429449432462,2.147408477853,-2.51427130483));
#13253=CARTESIAN_POINT('Ctrl Pts',(1.588699432462,3.102099467523,-1.144425205895));
#13254=CARTESIAN_POINT('Ctrl Pts',(1.747949432462,3.265768497555,0.5172460551354));
#13255=CARTESIAN_POINT('Ctrl Pts',(1.907199432462,2.59663025113,2.047018765263));
#13256=CARTESIAN_POINT('Ctrl Pts',(2.066449432462,1.265333295377,3.054784452443));
#13257=CARTESIAN_POINT('Ctrl Pts',(2.225699432462,-0.3886344899198,3.283555947824));
#13258=CARTESIAN_POINT('Ctrl Pts',(2.384949432462,-1.943497179912,2.674994390568));
#13259=CARTESIAN_POINT('Ctrl Pts',(2.544199432462,-3.002752621272,1.384287918735));
#13260=CARTESIAN_POINT('Ctrl Pts',(2.703449432462,-3.296282150534,-0.2594230316885));
#13261=CARTESIAN_POINT('Ctrl Pts',(2.862699432462,-2.749233411565,-1.836979036087));
#13262=CARTESIAN_POINT('Ctrl Pts',(3.021949432462,-1.501108196656,-2.946090716765));
#13263=CARTESIAN_POINT('Ctrl Pts',(3.181199432462,0.1298115957604,-3.303925737529));
#13264=CARTESIAN_POINT('Ctrl Pts',(3.340449432462,1.727628394674,-2.819233310576));
#13265=CARTESIAN_POINT('Ctrl Pts',(3.499699432462,2.884886156338,-1.615613875434));
#13266=CARTESIAN_POINT('Ctrl Pts',(3.658949432462,3.30647490986,0.));
#13267=CARTESIAN_POINT('Ctrl Pts',(3.818199432462,2.884886156338,1.615613875434));
#13268=CARTESIAN_POINT('Ctrl Pts',(3.977449432462,1.727628394674,2.819233310576));
#13269=CARTESIAN_POINT('Ctrl Pts',(4.136699432462,0.1298115957604,3.303925737529));
#13270=CARTESIAN_POINT('Ctrl Pts',(4.295949432462,-1.501108196656,2.946090716765));
#13271=CARTESIAN_POINT('Ctrl Pts',(4.455199432462,-2.749233411565,1.836979036087));
#13272=CARTESIAN_POINT('Ctrl Pts',(4.614449432462,-3.296282150534,0.2594230316885));
#13273=CARTESIAN_POINT('Ctrl Pts',(4.773699432462,-3.002752621272,-1.384287918735));
#13274=CARTESIAN_POINT('Ctrl Pts',(4.932949432462,-1.943497179912,-2.674994390568));
#13275=CARTESIAN_POINT('Ctrl Pts',(5.092199432462,-0.3886344899198,-3.283555947824));
#13276=CARTESIAN_POINT('Ctrl Pts',(5.251449432462,1.265333295377,-3.054784452443));
#13277=CARTESIAN_POINT('Ctrl Pts',(5.410699432462,2.59663025113,-2.047018765263));
#13278=CARTESIAN_POINT('Ctrl Pts',(5.569949432462,3.265768497555,-0.5172460551354));
#13279=CARTESIAN_POINT('Ctrl Pts',(5.729199432462,3.102099467523,1.144425205895));
#13280=CARTESIAN_POINT('Ctrl Pts',(5.888449432462,2.147408477853,2.51427130483));
#13281=CARTESIAN_POINT('Ctrl Pts',(6.047699432462,0.6449686970875,3.242911847755));
#13282=CARTESIAN_POINT('Ctrl Pts',(6.153866099128,-0.4659514397387,3.177475113353));
#13283=CARTESIAN_POINT('Ctrl Pts',(6.206949432462,-0.9783309087958,3.010992931911));
#13284=CARTESIAN_POINT('',(6.12500744527969,7.41993572688973E-7,3.12499989450239));
#13285=CARTESIAN_POINT('Ctrl Pts',(1.2249865253955,-1.42385617185603E-10,
-3.12449703075058));
#13286=CARTESIAN_POINT('Ctrl Pts',(1.2469582081062,0.220105501026209,-3.12463783133622));
#13287=CARTESIAN_POINT('Ctrl Pts',(1.26897679573541,0.440651235200038,-3.10173887397659));
#13288=CARTESIAN_POINT('Ctrl Pts',(1.31310572384028,0.872618743152088,-3.00870835952898));
#13289=CARTESIAN_POINT('Ctrl Pts',(1.33514657553483,1.08338871438441,-2.93893910181466));
#13290=CARTESIAN_POINT('Ctrl Pts',(1.38629053209713,1.55043320018979,-2.72810358228178));
#13291=CARTESIAN_POINT('Ctrl Pts',(1.42779283828223,1.92091911867349,-2.51858797774255));
#13292=CARTESIAN_POINT('Ctrl Pts',(1.5192164507904,2.54824617086084,-1.85148038354481));
#13293=CARTESIAN_POINT('Ctrl Pts',(1.55919669615488,2.76667000678541,-1.50682910689434));
#13294=CARTESIAN_POINT('Ctrl Pts',(1.64240102883077,3.06923750138773,-0.730496208269496));
#13295=CARTESIAN_POINT('Ctrl Pts',(1.68319131879263,3.13182588768285,-0.318472133625833));
#13296=CARTESIAN_POINT('Ctrl Pts',(1.77384690094005,3.11321199907849,0.589454969171755));
#13297=CARTESIAN_POINT('Ctrl Pts',(1.81566769599401,2.97612381593503,0.996047824886873));
#13298=CARTESIAN_POINT('Ctrl Pts',(1.87566680271497,2.73245626285589,1.54560310783317));
#13299=CARTESIAN_POINT('Ctrl Pts',(1.91705708412132,2.5223074836412,1.91404302998658));
#13300=CARTESIAN_POINT('Ctrl Pts',(2.00557929492136,1.87904024871205,2.52442476815786));
#13301=CARTESIAN_POINT('Ctrl Pts',(2.04549804777898,1.54078105288759,2.75166775493569));
#13302=CARTESIAN_POINT('Ctrl Pts',(2.1284307618169,0.768144592726455,3.05621103088524));
#13303=CARTESIAN_POINT('Ctrl Pts',(2.16908686746197,0.359581070464753,3.13013165576389));
#13304=CARTESIAN_POINT('Ctrl Pts',(2.26176471540898,-0.568604604223949,
3.11705696110185));
#13305=CARTESIAN_POINT('Ctrl Pts',(2.30373757339158,-0.977563840795589,
2.9820103808569));
#13306=CARTESIAN_POINT('Ctrl Pts',(2.37430055630902,-1.62585920990471,2.69999321328487));
#13307=CARTESIAN_POINT('Ctrl Pts',(2.41487067374851,-1.96613181358351,2.46385086322353));
#13308=CARTESIAN_POINT('Ctrl Pts',(2.48543046710326,-2.45553051679632,1.95376212132771));
#13309=CARTESIAN_POINT('Ctrl Pts',(2.52677217877916,-2.71875343764017,1.62181272348733));
#13310=CARTESIAN_POINT('Ctrl Pts',(2.61751008605416,-3.05336233804938,0.776946962299032));
#13311=CARTESIAN_POINT('Ctrl Pts',(2.65791907247006,-3.1286208842104,0.371271841828455));
#13312=CARTESIAN_POINT('Ctrl Pts',(2.75122878779405,-3.1195612174274,-0.563189413652714));
#13313=CARTESIAN_POINT('Ctrl Pts',(2.79352621934935,-2.9814101539477,-0.975053271184112));
#13314=CARTESIAN_POINT('Ctrl Pts',(2.86288521992931,-2.70782042248997,-1.61380337445919));
#13315=CARTESIAN_POINT('Ctrl Pts',(2.90352769034976,-2.47211612449971,-1.955325207837));
#13316=CARTESIAN_POINT('Ctrl Pts',(2.97355979919688,-1.96811675189464,-2.44349049201393));
#13317=CARTESIAN_POINT('Ctrl Pts',(3.01507806923606,-1.63734153359,-2.71166246485518));
#13318=CARTESIAN_POINT('Ctrl Pts',(3.10669238599482,-0.78471093229284,-3.05077446246927));
#13319=CARTESIAN_POINT('Ctrl Pts',(3.14681070224775,-0.382385740435305,
-3.12715191531059));
#13320=CARTESIAN_POINT('Ctrl Pts',(3.23204749336205,0.471183768083653,-3.12237996970145));
#13321=CARTESIAN_POINT('Ctrl Pts',(3.27300860642011,0.877409231626752,-3.02091407068733));
#13322=CARTESIAN_POINT('Ctrl Pts',(3.35984142912634,1.67903873524075,-2.68319768942736));
#13323=CARTESIAN_POINT('Ctrl Pts',(3.40138319477005,2.00874122018005,-2.41423377541334));
#13324=CARTESIAN_POINT('Ctrl Pts',(3.4616942874132,2.43162777346986,-1.98258700351926));
#13325=CARTESIAN_POINT('Ctrl Pts',(3.50323523064722,2.70311754303438,-1.65387788875614));
#13326=CARTESIAN_POINT('Ctrl Pts',(3.59538249933782,3.04697916736015,-0.79728039457302));
#13327=CARTESIAN_POINT('Ctrl Pts',(3.63518829630558,3.125,-0.398671791438241));
#13328=CARTESIAN_POINT('Ctrl Pts',(3.71481170369442,3.125,0.39867179143824));
#13329=CARTESIAN_POINT('Ctrl Pts',(3.75461750066256,3.04697916736015,0.797280394573017));
#13330=CARTESIAN_POINT('Ctrl Pts',(3.84676476935332,2.70311754303439,1.65387788875614));
#13331=CARTESIAN_POINT('Ctrl Pts',(3.88830571258727,2.43162777346986,1.98258700351927));
#13332=CARTESIAN_POINT('Ctrl Pts',(3.94861680523022,2.00874122018,2.4142337754134));
#13333=CARTESIAN_POINT('Ctrl Pts',(3.9901585708736,1.6790387352407,2.68319768942738));
#13334=CARTESIAN_POINT('Ctrl Pts',(4.07699139357983,0.877409231626905,3.02091407068727));
#13335=CARTESIAN_POINT('Ctrl Pts',(4.11795250663809,0.471183768083811,3.12237996970145));
#13336=CARTESIAN_POINT('Ctrl Pts',(4.20318929775232,-0.382385740435277,
3.12715191531059));
#13337=CARTESIAN_POINT('Ctrl Pts',(4.24330761400502,-0.78471093229281,3.05077446246928));
#13338=CARTESIAN_POINT('Ctrl Pts',(4.33492193076373,-1.63734153358998,2.71166246485519));
#13339=CARTESIAN_POINT('Ctrl Pts',(4.37644020080298,-1.96811675189461,2.44349049201395));
#13340=CARTESIAN_POINT('Ctrl Pts',(4.44647230965025,-2.4721161244997,1.95532520783702));
#13341=CARTESIAN_POINT('Ctrl Pts',(4.48711478007087,-2.70782042248996,1.6138033744592));
#13342=CARTESIAN_POINT('Ctrl Pts',(4.55647378065097,-2.98141015394769,0.97505327118414));
#13343=CARTESIAN_POINT('Ctrl Pts',(4.5987712122064,-3.1195612174274,0.563189413652733));
#13344=CARTESIAN_POINT('Ctrl Pts',(4.69208092753042,-3.1286208842104,-0.371271841828482));
#13345=CARTESIAN_POINT('Ctrl Pts',(4.73248991394627,-3.05336233804938,-0.776946962299062));
#13346=CARTESIAN_POINT('Ctrl Pts',(4.82322782122118,-2.71875343764019,-1.62181272348726));
#13347=CARTESIAN_POINT('Ctrl Pts',(4.864569532897,-2.45553051679639,-1.95376212132765));
#13348=CARTESIAN_POINT('Ctrl Pts',(4.93512932625151,-1.96613181358349,-2.46385086322354));
#13349=CARTESIAN_POINT('Ctrl Pts',(4.9756994436907,-1.62585920990471,-2.69999321328486));
#13350=CARTESIAN_POINT('Ctrl Pts',(5.04626242660797,-0.977563840795617,
-2.98201038085689));
#13351=CARTESIAN_POINT('Ctrl Pts',(5.08823528459042,-0.568604604223984,
-3.11705696110184));
#13352=CARTESIAN_POINT('Ctrl Pts',(5.18091313253766,0.359581070464712,-3.13013165576389));
#13353=CARTESIAN_POINT('Ctrl Pts',(5.22156923818307,0.76814459272642,-3.05621103088525));
#13354=CARTESIAN_POINT('Ctrl Pts',(5.30450195222119,1.54078105288758,-2.7516677549357));
#13355=CARTESIAN_POINT('Ctrl Pts',(5.34442070507877,1.87904024871205,-2.52442476815786));
#13356=CARTESIAN_POINT('Ctrl Pts',(5.43294291587883,2.52230748364104,-1.91404302998674));
#13357=CARTESIAN_POINT('Ctrl Pts',(5.47433319728519,2.73245626285581,-1.54560310783341));
#13358=CARTESIAN_POINT('Ctrl Pts',(5.5343323040062,2.97612381593512,-0.9960478248867));
#13359=CARTESIAN_POINT('Ctrl Pts',(5.57615309906016,3.1132119990785,-0.589454969171629));
#13360=CARTESIAN_POINT('Ctrl Pts',(5.66680868120744,3.13182588768285,0.31847213362576));
#13361=CARTESIAN_POINT('Ctrl Pts',(5.70759897116911,3.06923750138774,0.730496208269452));
#13362=CARTESIAN_POINT('Ctrl Pts',(5.79080330384514,2.7666700067854,1.50682910689435));
#13363=CARTESIAN_POINT('Ctrl Pts',(5.83078354921002,2.54824617086083,1.85148038354482));
#13364=CARTESIAN_POINT('Ctrl Pts',(5.92220716171829,1.92091911867347,2.51858797774256));
#13365=CARTESIAN_POINT('Ctrl Pts',(5.9637094679032,1.55043320018976,2.7281035822818));
#13366=CARTESIAN_POINT('Ctrl Pts',(6.01485344133236,1.08338856035466,2.93893917134752));
#13367=CARTESIAN_POINT('Ctrl Pts',(6.0368943099015,0.872618420486184,3.00870846633562));
#13368=CARTESIAN_POINT('Ctrl Pts',(6.08102337747936,0.440649532003025,3.10173920341104));
#13369=CARTESIAN_POINT('Ctrl Pts',(6.10304208760836,0.220102539161381,3.12463812164867));
#13370=CARTESIAN_POINT('Ctrl Pts',(6.12501389259301,-4.18742151370166E-6,
3.12449702806922));
#13371=CARTESIAN_POINT('',(6.468,0.,2.25));
#13372=CARTESIAN_POINT('Ctrl Pts',(6.386050567538,0.6826354359695,2.100935843176));
#13373=CARTESIAN_POINT('Ctrl Pts',(6.439133900872,0.3251200195628,2.217099643673));
#13374=CARTESIAN_POINT('Ctrl Pts',(6.545300567538,-0.4500302339061,2.2627584625));
#13375=CARTESIAN_POINT('Ctrl Pts',(6.704550567538,-1.498365337642,1.754345766741));
#13376=CARTESIAN_POINT('Ctrl Pts',(6.863800567538,-2.164505898152,0.7985285881669));
#13377=CARTESIAN_POINT('Ctrl Pts',(7.023050567538,-2.278706807749,-0.3609111019352));
#13378=CARTESIAN_POINT('Ctrl Pts',(7.182300567538,-1.811812146172,-1.428317898065));
#13379=CARTESIAN_POINT('Ctrl Pts',(7.341550567538,-0.8828928310149,-2.13149160242));
#13380=CARTESIAN_POINT('Ctrl Pts',(7.500800567538,0.271171719174,-2.291118092888));
#13381=CARTESIAN_POINT('Ctrl Pts',(7.660050567538,1.35608517812,-1.866491128517));
#13382=CARTESIAN_POINT('Ctrl Pts',(7.819300567538,2.09518612394,-0.9658940328033));
#13383=CARTESIAN_POINT('Ctrl Pts',(7.978550567538,2.299997866445,0.1810137579678));
#13384=CARTESIAN_POINT('Ctrl Pts',(8.137800567538,1.918291788201,1.281761594049));
#13385=CARTESIAN_POINT('Ctrl Pts',(8.297050567538,1.047405984058,2.055649987917));
#13386=CARTESIAN_POINT('Ctrl Pts',(8.456300567538,-0.0905767102614,2.305331218682));
#13387=CARTESIAN_POINT('Ctrl Pts',(8.615550567538,-1.205461620183,1.967134578661));
#13388=CARTESIAN_POINT('Ctrl Pts',(8.774800567538,-2.012944190303,1.127302911826));
#13389=CARTESIAN_POINT('Ctrl Pts',(8.934050567538,-2.30710991682,0.));
#13390=CARTESIAN_POINT('Ctrl Pts',(9.093300567538,-2.012944190303,-1.127302911826));
#13391=CARTESIAN_POINT('Ctrl Pts',(9.252550567538,-1.205461620183,-1.967134578661));
#13392=CARTESIAN_POINT('Ctrl Pts',(9.411800567538,-0.09057671026141,-2.305331218682));
#13393=CARTESIAN_POINT('Ctrl Pts',(9.571050567538,1.047405984058,-2.055649987917));
#13394=CARTESIAN_POINT('Ctrl Pts',(9.730300567538,1.918291788201,-1.281761594049));
#13395=CARTESIAN_POINT('Ctrl Pts',(9.889550567538,2.299997866445,-0.1810137579678));
#13396=CARTESIAN_POINT('Ctrl Pts',(10.04880056754,2.09518612394,0.9658940328033));
#13397=CARTESIAN_POINT('Ctrl Pts',(10.20805056754,1.35608517812,1.866491128517));
#13398=CARTESIAN_POINT('Ctrl Pts',(10.36730056754,0.271171719174,2.291118092888));
#13399=CARTESIAN_POINT('Ctrl Pts',(10.52655056754,-0.8828928310149,2.13149160242));
#13400=CARTESIAN_POINT('Ctrl Pts',(10.68580056754,-1.811812146172,1.428317898065));
#13401=CARTESIAN_POINT('Ctrl Pts',(10.84505056754,-2.278706807749,0.3609111019352));
#13402=CARTESIAN_POINT('Ctrl Pts',(11.00430056754,-2.164505898152,-0.7985285881669));
#13403=CARTESIAN_POINT('Ctrl Pts',(11.16355056754,-1.498365337642,-1.754345766741));
#13404=CARTESIAN_POINT('Ctrl Pts',(11.32280056754,-0.4500302339061,-2.2627584625));
#13405=CARTESIAN_POINT('Ctrl Pts',(11.4289672342,0.3251200195628,-2.217099643673));
#13406=CARTESIAN_POINT('Ctrl Pts',(11.48205056754,0.6826354359695,-2.100935843176));
#13407=CARTESIAN_POINT('Ctrl Pts',(6.261016855846,0.7812005935783,2.404288206087));
#13408=CARTESIAN_POINT('Ctrl Pts',(6.314100189179,0.3720638262881,2.537224800233));
#13409=CARTESIAN_POINT('Ctrl Pts',(6.420266855846,-0.5150097216332,2.589476257585));
#13410=CARTESIAN_POINT('Ctrl Pts',(6.579516855846,-1.714713051046,2.007654279437));
#13411=CARTESIAN_POINT('Ctrl Pts',(6.738766855846,-2.477037087943,0.9138274607431));
#13412=CARTESIAN_POINT('Ctrl Pts',(6.898016855846,-2.607727371018,-0.4130227530019));
#13413=CARTESIAN_POINT('Ctrl Pts',(7.057266855846,-2.073418181158,-1.634551520464));
#13414=CARTESIAN_POINT('Ctrl Pts',(7.216516855846,-1.010372985802,-2.439255885761));
#13415=CARTESIAN_POINT('Ctrl Pts',(7.375766855846,0.3103259760892,-2.6219307112));
#13416=CARTESIAN_POINT('Ctrl Pts',(7.535016855846,1.551889178717,-2.135992215868));
#13417=CARTESIAN_POINT('Ctrl Pts',(7.694266855846,2.397708289717,-1.105358661447));
#13418=CARTESIAN_POINT('Ctrl Pts',(7.853516855846,2.632092627808,0.2071501825414));
#13419=CARTESIAN_POINT('Ctrl Pts',(8.012766855846,2.195272329322,1.466834074728));
#13420=CARTESIAN_POINT('Ctrl Pts',(8.172016855846,1.198640054924,2.3524635642));
#13421=CARTESIAN_POINT('Ctrl Pts',(8.331266855846,-0.1036550054277,2.638196058298));
#13422=CARTESIAN_POINT('Ctrl Pts',(8.490516855846,-1.37951721168,2.251167489299));
#13423=CARTESIAN_POINT('Ctrl Pts',(8.649766855846,-2.303591512314,1.290073233029));
#13424=CARTESIAN_POINT('Ctrl Pts',(8.809016855846,-2.640231581167,1.108429745068E-14));
#13425=CARTESIAN_POINT('Ctrl Pts',(8.968266855846,-2.303591512314,-1.290073233029));
#13426=CARTESIAN_POINT('Ctrl Pts',(9.127516855846,-1.37951721168,-2.251167489299));
#13427=CARTESIAN_POINT('Ctrl Pts',(9.286766855846,-0.1036550054277,-2.638196058298));
#13428=CARTESIAN_POINT('Ctrl Pts',(9.446016855846,1.198640054924,-2.3524635642));
#13429=CARTESIAN_POINT('Ctrl Pts',(9.605266855846,2.195272329322,-1.466834074728));
#13430=CARTESIAN_POINT('Ctrl Pts',(9.764516855846,2.632092627808,-0.2071501825414));
#13431=CARTESIAN_POINT('Ctrl Pts',(9.923766855846,2.397708289717,1.105358661447));
#13432=CARTESIAN_POINT('Ctrl Pts',(10.08301685585,1.551889178717,2.135992215868));
#13433=CARTESIAN_POINT('Ctrl Pts',(10.24226685585,0.3103259760892,2.6219307112));
#13434=CARTESIAN_POINT('Ctrl Pts',(10.40151685585,-1.010372985802,2.439255885761));
#13435=CARTESIAN_POINT('Ctrl Pts',(10.56076685585,-2.073418181158,1.634551520464));
#13436=CARTESIAN_POINT('Ctrl Pts',(10.72001685585,-2.607727371018,0.4130227530019));
#13437=CARTESIAN_POINT('Ctrl Pts',(10.87926685585,-2.477037087943,-0.913827460743));
#13438=CARTESIAN_POINT('Ctrl Pts',(11.03851685585,-1.714713051046,-2.007654279437));
#13439=CARTESIAN_POINT('Ctrl Pts',(11.19776685585,-0.5150097216332,-2.589476257585));
#13440=CARTESIAN_POINT('Ctrl Pts',(11.30393352251,0.3720638262881,-2.537224800233));
#13441=CARTESIAN_POINT('Ctrl Pts',(11.35701685585,0.7812005935783,-2.404288206087));
#13442=CARTESIAN_POINT('Ctrl Pts',(6.135983144154,0.8797657511871,2.707640568999));
#13443=CARTESIAN_POINT('Ctrl Pts',(6.189066477487,0.4190076330134,2.857349956793));
#13444=CARTESIAN_POINT('Ctrl Pts',(6.295233144154,-0.5799892093603,2.91619405267));
#13445=CARTESIAN_POINT('Ctrl Pts',(6.454483144154,-1.931060764449,2.260962792133));
#13446=CARTESIAN_POINT('Ctrl Pts',(6.613733144154,-2.789568277733,1.029126333319));
#13447=CARTESIAN_POINT('Ctrl Pts',(6.772983144154,-2.936747934286,-0.4651344040686));
#13448=CARTESIAN_POINT('Ctrl Pts',(6.932233144154,-2.335024216144,-1.840785142863));
#13449=CARTESIAN_POINT('Ctrl Pts',(7.091483144154,-1.137853140589,-2.747020169102));
#13450=CARTESIAN_POINT('Ctrl Pts',(7.250733144154,0.3494802330045,-2.952743329512));
#13451=CARTESIAN_POINT('Ctrl Pts',(7.409983144154,1.747693179314,-2.405493303218));
#13452=CARTESIAN_POINT('Ctrl Pts',(7.569233144154,2.700230455495,-1.244823290091));
#13453=CARTESIAN_POINT('Ctrl Pts',(7.728483144154,2.964187389171,0.2332866071149));
#13454=CARTESIAN_POINT('Ctrl Pts',(7.887733144154,2.472252870444,1.651906555408));
#13455=CARTESIAN_POINT('Ctrl Pts',(8.046983144154,1.34987412579,2.649277140482));
#13456=CARTESIAN_POINT('Ctrl Pts',(8.206233144154,-0.116733300594,2.971060897913));
#13457=CARTESIAN_POINT('Ctrl Pts',(8.365483144154,-1.553572803177,2.535200399938));
#13458=CARTESIAN_POINT('Ctrl Pts',(8.524733144154,-2.594238834326,1.452843554231));
#13459=CARTESIAN_POINT('Ctrl Pts',(8.683983144154,-2.973353245513,1.647272319884E-14));
#13460=CARTESIAN_POINT('Ctrl Pts',(8.843233144154,-2.594238834326,-1.452843554231));
#13461=CARTESIAN_POINT('Ctrl Pts',(9.002483144154,-1.553572803177,-2.535200399938));
#13462=CARTESIAN_POINT('Ctrl Pts',(9.161733144154,-0.1167333005941,-2.971060897913));
#13463=CARTESIAN_POINT('Ctrl Pts',(9.320983144154,1.34987412579,-2.649277140482));
#13464=CARTESIAN_POINT('Ctrl Pts',(9.480233144154,2.472252870444,-1.651906555408));
#13465=CARTESIAN_POINT('Ctrl Pts',(9.639483144154,2.964187389171,-0.2332866071149));
#13466=CARTESIAN_POINT('Ctrl Pts',(9.798733144154,2.700230455495,1.244823290091));
#13467=CARTESIAN_POINT('Ctrl Pts',(9.957983144154,1.747693179314,2.405493303218));
#13468=CARTESIAN_POINT('Ctrl Pts',(10.11723314415,0.3494802330045,2.952743329512));
#13469=CARTESIAN_POINT('Ctrl Pts',(10.27648314415,-1.137853140589,2.747020169102));
#13470=CARTESIAN_POINT('Ctrl Pts',(10.43573314415,-2.335024216144,1.840785142863));
#13471=CARTESIAN_POINT('Ctrl Pts',(10.59498314415,-2.936747934286,0.4651344040687));
#13472=CARTESIAN_POINT('Ctrl Pts',(10.75423314415,-2.789568277733,-1.029126333319));
#13473=CARTESIAN_POINT('Ctrl Pts',(10.91348314415,-1.931060764449,-2.260962792133));
#13474=CARTESIAN_POINT('Ctrl Pts',(11.07273314415,-0.5799892093604,-2.91619405267));
#13475=CARTESIAN_POINT('Ctrl Pts',(11.17889981082,0.4190076330134,-2.857349956793));
#13476=CARTESIAN_POINT('Ctrl Pts',(11.23198314415,0.8797657511871,-2.707640568999));
#13477=CARTESIAN_POINT('Ctrl Pts',(6.010949432462,0.9783309087958,3.010992931911));
#13478=CARTESIAN_POINT('Ctrl Pts',(6.064032765795,0.4659514397387,3.177475113353));
#13479=CARTESIAN_POINT('Ctrl Pts',(6.170199432462,-0.6449686970874,3.242911847755));
#13480=CARTESIAN_POINT('Ctrl Pts',(6.329449432462,-2.147408477853,2.51427130483));
#13481=CARTESIAN_POINT('Ctrl Pts',(6.488699432462,-3.102099467523,1.144425205895));
#13482=CARTESIAN_POINT('Ctrl Pts',(6.647949432462,-3.265768497555,-0.5172460551353));
#13483=CARTESIAN_POINT('Ctrl Pts',(6.807199432462,-2.59663025113,-2.047018765263));
#13484=CARTESIAN_POINT('Ctrl Pts',(6.966449432462,-1.265333295377,-3.054784452443));
#13485=CARTESIAN_POINT('Ctrl Pts',(7.125699432462,0.3886344899198,-3.283555947824));
#13486=CARTESIAN_POINT('Ctrl Pts',(7.284949432462,1.943497179912,-2.674994390568));
#13487=CARTESIAN_POINT('Ctrl Pts',(7.444199432462,3.002752621272,-1.384287918735));
#13488=CARTESIAN_POINT('Ctrl Pts',(7.603449432462,3.296282150534,0.2594230316885));
#13489=CARTESIAN_POINT('Ctrl Pts',(7.762699432462,2.749233411565,1.836979036087));
#13490=CARTESIAN_POINT('Ctrl Pts',(7.921949432462,1.501108196656,2.946090716765));
#13491=CARTESIAN_POINT('Ctrl Pts',(8.081199432462,-0.1298115957604,3.303925737529));
#13492=CARTESIAN_POINT('Ctrl Pts',(8.240449432462,-1.727628394674,2.819233310576));
#13493=CARTESIAN_POINT('Ctrl Pts',(8.399699432462,-2.884886156338,1.615613875434));
#13494=CARTESIAN_POINT('Ctrl Pts',(8.558949432462,-3.30647490986,1.754152378908E-14));
#13495=CARTESIAN_POINT('Ctrl Pts',(8.718199432462,-2.884886156338,-1.615613875434));
#13496=CARTESIAN_POINT('Ctrl Pts',(8.877449432462,-1.727628394674,-2.819233310576));
#13497=CARTESIAN_POINT('Ctrl Pts',(9.036699432462,-0.1298115957604,-3.303925737529));
#13498=CARTESIAN_POINT('Ctrl Pts',(9.195949432462,1.501108196656,-2.946090716765));
#13499=CARTESIAN_POINT('Ctrl Pts',(9.355199432462,2.749233411565,-1.836979036087));
#13500=CARTESIAN_POINT('Ctrl Pts',(9.514449432462,3.296282150534,-0.2594230316885));
#13501=CARTESIAN_POINT('Ctrl Pts',(9.673699432462,3.002752621272,1.384287918735));
#13502=CARTESIAN_POINT('Ctrl Pts',(9.832949432462,1.943497179912,2.674994390568));
#13503=CARTESIAN_POINT('Ctrl Pts',(9.992199432462,0.3886344899198,3.283555947824));
#13504=CARTESIAN_POINT('Ctrl Pts',(10.15144943246,-1.265333295377,3.054784452443));
#13505=CARTESIAN_POINT('Ctrl Pts',(10.31069943246,-2.59663025113,2.047018765263));
#13506=CARTESIAN_POINT('Ctrl Pts',(10.46994943246,-3.265768497555,0.5172460551354));
#13507=CARTESIAN_POINT('Ctrl Pts',(10.62919943246,-3.102099467523,-1.144425205895));
#13508=CARTESIAN_POINT('Ctrl Pts',(10.78844943246,-2.147408477853,-2.51427130483));
#13509=CARTESIAN_POINT('Ctrl Pts',(10.94769943246,-0.6449686970875,-3.242911847755));
#13510=CARTESIAN_POINT('Ctrl Pts',(11.05386609913,0.4659514397387,-3.177475113353));
#13511=CARTESIAN_POINT('Ctrl Pts',(11.10694943246,0.9783309087959,-3.010992931911));
#13512=CARTESIAN_POINT('',(11.0250134741351,-1.1227774403895E-10,-3.12449703104719));
#13513=CARTESIAN_POINT('Ctrl Pts',(6.12498723189613,-7.07736163719358E-6,
3.12449703527009));
#13514=CARTESIAN_POINT('Ctrl Pts',(6.14695866368768,-0.220110064033207,
3.12463734035084));
#13515=CARTESIAN_POINT('Ctrl Pts',(6.16897699922435,-0.440653219467678,
3.1017384092623));
#13516=CARTESIAN_POINT('Ctrl Pts',(6.21310569009841,-0.87261842048626,3.0087084663356));
#13517=CARTESIAN_POINT('Ctrl Pts',(6.23514655866772,-1.08338856035471,2.9389391713475));
#13518=CARTESIAN_POINT('Ctrl Pts',(6.28629053209712,-1.55043320018978,2.72810358228179));
#13519=CARTESIAN_POINT('Ctrl Pts',(6.32779283828223,-1.92091911867348,2.51858797774255));
#13520=CARTESIAN_POINT('Ctrl Pts',(6.4192164507904,-2.54824617086084,1.85148038354481));
#13521=CARTESIAN_POINT('Ctrl Pts',(6.45919669615489,-2.76667000678541,1.50682910689433));
#13522=CARTESIAN_POINT('Ctrl Pts',(6.54240102883078,-3.06923750138774,0.730496208269489));
#13523=CARTESIAN_POINT('Ctrl Pts',(6.58319131879264,-3.13182588768285,0.318472133625827));
#13524=CARTESIAN_POINT('Ctrl Pts',(6.67384690094006,-3.11321199907849,-0.589454969171753));
#13525=CARTESIAN_POINT('Ctrl Pts',(6.715667695994,-2.97612381593503,-0.996047824886871));
#13526=CARTESIAN_POINT('Ctrl Pts',(6.77566680271496,-2.73245626285591,-1.54560310783311));
#13527=CARTESIAN_POINT('Ctrl Pts',(6.81705708412131,-2.52230748364124,-1.91404302998654));
#13528=CARTESIAN_POINT('Ctrl Pts',(6.90557929492136,-1.87904024871203,-2.52442476815788));
#13529=CARTESIAN_POINT('Ctrl Pts',(6.94549804777898,-1.54078105288757,-2.7516677549357));
#13530=CARTESIAN_POINT('Ctrl Pts',(7.0284307618169,-0.768144592726452,-3.05621103088524));
#13531=CARTESIAN_POINT('Ctrl Pts',(7.06908686746197,-0.359581070464751,
-3.13013165576389));
#13532=CARTESIAN_POINT('Ctrl Pts',(7.16176471540898,0.56860460422395,-3.11705696110185));
#13533=CARTESIAN_POINT('Ctrl Pts',(7.20373757339158,0.97756384079559,-2.9820103808569));
#13534=CARTESIAN_POINT('Ctrl Pts',(7.27430055630902,1.62585920990471,-2.69999321328487));
#13535=CARTESIAN_POINT('Ctrl Pts',(7.31487067374851,1.96613181358351,-2.46385086322353));
#13536=CARTESIAN_POINT('Ctrl Pts',(7.38543046710326,2.45553051679631,-1.95376212132773));
#13537=CARTESIAN_POINT('Ctrl Pts',(7.42677217877916,2.71875343764016,-1.62181272348735));
#13538=CARTESIAN_POINT('Ctrl Pts',(7.51751008605417,3.05336233804939,-0.776946962299028));
#13539=CARTESIAN_POINT('Ctrl Pts',(7.55791907247006,3.1286208842104,-0.371271841828451));
#13540=CARTESIAN_POINT('Ctrl Pts',(7.65122878779405,3.1195612174274,0.563189413652742));
#13541=CARTESIAN_POINT('Ctrl Pts',(7.69352621934936,2.98141015394768,0.975053271184142));
#13542=CARTESIAN_POINT('Ctrl Pts',(7.76288521992931,2.70782042248997,1.61380337445919));
#13543=CARTESIAN_POINT('Ctrl Pts',(7.80352769034976,2.47211612449971,1.955325207837));
#13544=CARTESIAN_POINT('Ctrl Pts',(7.87355979919688,1.96811675189463,2.44349049201393));
#13545=CARTESIAN_POINT('Ctrl Pts',(7.91507806923605,1.63734153359,2.71166246485518));
#13546=CARTESIAN_POINT('Ctrl Pts',(8.00669238599482,0.78471093229284,3.05077446246927));
#13547=CARTESIAN_POINT('Ctrl Pts',(8.04681070224775,0.382385740435304,3.12715191531059));
#13548=CARTESIAN_POINT('Ctrl Pts',(8.13204749336205,-0.471183768083647,
3.12237996970145));
#13549=CARTESIAN_POINT('Ctrl Pts',(8.17300860642011,-0.877409231626746,
3.02091407068734));
#13550=CARTESIAN_POINT('Ctrl Pts',(8.25984142912633,-1.67903873524074,2.68319768942737));
#13551=CARTESIAN_POINT('Ctrl Pts',(8.30138319477005,-2.00874122018004,2.41423377541336));
#13552=CARTESIAN_POINT('Ctrl Pts',(8.3616942874132,-2.43162777346988,1.98258700351925));
#13553=CARTESIAN_POINT('Ctrl Pts',(8.40323523064723,-2.70311754303439,1.65387788875613));
#13554=CARTESIAN_POINT('Ctrl Pts',(8.49538249933782,-3.04697916736015,0.79728039457302));
#13555=CARTESIAN_POINT('Ctrl Pts',(8.53518829630558,-3.125,0.398671791438241));
#13556=CARTESIAN_POINT('Ctrl Pts',(8.61481170369442,-3.125,-0.398671791438241));
#13557=CARTESIAN_POINT('Ctrl Pts',(8.65461750066257,-3.04697916736015,-0.797280394573019));
#13558=CARTESIAN_POINT('Ctrl Pts',(8.74676476935333,-2.70311754303436,-1.65387788875621));
#13559=CARTESIAN_POINT('Ctrl Pts',(8.78830571258729,-2.4316277734698,-1.98258700351933));
#13560=CARTESIAN_POINT('Ctrl Pts',(8.84861680523022,-2.00874122018003,-2.41423377541336));
#13561=CARTESIAN_POINT('Ctrl Pts',(8.89015857087361,-1.67903873524074,-2.68319768942736));
#13562=CARTESIAN_POINT('Ctrl Pts',(8.97699139357984,-0.877409231626881,
-3.02091407068728));
#13563=CARTESIAN_POINT('Ctrl Pts',(9.0179525066381,-0.471183768083787,-3.12237996970145));
#13564=CARTESIAN_POINT('Ctrl Pts',(9.10318929775232,0.382385740435283,-3.12715191531059));
#13565=CARTESIAN_POINT('Ctrl Pts',(9.14330761400503,0.784710932292816,-3.05077446246928));
#13566=CARTESIAN_POINT('Ctrl Pts',(9.23492193076374,1.63734153358998,-2.71166246485519));
#13567=CARTESIAN_POINT('Ctrl Pts',(9.27644020080298,1.96811675189461,-2.44349049201395));
#13568=CARTESIAN_POINT('Ctrl Pts',(9.34647230965026,2.4721161244997,-1.95532520783702));
#13569=CARTESIAN_POINT('Ctrl Pts',(9.38711478007088,2.70782042248997,-1.61380337445919));
#13570=CARTESIAN_POINT('Ctrl Pts',(9.45647378065097,2.98141015394769,-0.97505327118413));
#13571=CARTESIAN_POINT('Ctrl Pts',(9.4987712122064,3.1195612174274,-0.563189413652723));
#13572=CARTESIAN_POINT('Ctrl Pts',(9.59208092753043,3.1286208842104,0.371271841828488));
#13573=CARTESIAN_POINT('Ctrl Pts',(9.63248991394628,3.05336233804938,0.776946962299067));
#13574=CARTESIAN_POINT('Ctrl Pts',(9.72322782122119,2.71875343764021,1.62181272348721));
#13575=CARTESIAN_POINT('Ctrl Pts',(9.76456953289697,2.45553051679643,1.95376212132761));
#13576=CARTESIAN_POINT('Ctrl Pts',(9.83512932625145,1.96613181358349,2.46385086322354));
#13577=CARTESIAN_POINT('Ctrl Pts',(9.87569944369059,1.62585920990472,2.69999321328486));
#13578=CARTESIAN_POINT('Ctrl Pts',(9.94626242660763,0.977563840795634,2.98201038085688));
#13579=CARTESIAN_POINT('Ctrl Pts',(9.98823528459023,0.568604604224015,3.11705696110183));
#13580=CARTESIAN_POINT('Ctrl Pts',(10.0809131325367,-0.359581070464643,
3.1301316557639));
#13581=CARTESIAN_POINT('Ctrl Pts',(10.1215692381812,-0.768144592726318,
3.05621103088527));
#13582=CARTESIAN_POINT('Ctrl Pts',(10.2045019522189,-1.54078105288753,2.75166775493574));
#13583=CARTESIAN_POINT('Ctrl Pts',(10.2444207050765,-1.87904024871197,2.5244247681579));
#13584=CARTESIAN_POINT('Ctrl Pts',(10.3329429158766,-2.52230748364106,1.91404302998675));
#13585=CARTESIAN_POINT('Ctrl Pts',(10.3743331972831,-2.73245626285578,1.54560310783337));
#13586=CARTESIAN_POINT('Ctrl Pts',(10.4343323040041,-2.97612381593498,0.996047824887012));
#13587=CARTESIAN_POINT('Ctrl Pts',(10.476153099058,-3.11321199907846,0.589454969171896));
#13588=CARTESIAN_POINT('Ctrl Pts',(10.5668086812053,-3.13182588768287,-0.31847213362573));
#13589=CARTESIAN_POINT('Ctrl Pts',(10.607598971167,-3.06923750138775,-0.730496208269382));
#13590=CARTESIAN_POINT('Ctrl Pts',(10.690803303843,-2.76667000678551,-1.50682910689415));
#13591=CARTESIAN_POINT('Ctrl Pts',(10.7307835492079,-2.54824617086096,-1.85148038354464));
#13592=CARTESIAN_POINT('Ctrl Pts',(10.8222071617162,-1.9209191186736,-2.51858797774247));
#13593=CARTESIAN_POINT('Ctrl Pts',(10.8637094679009,-1.55043320018988,-2.72810358228172));
#13594=CARTESIAN_POINT('Ctrl Pts',(10.9148534207039,-1.08338874871494,-2.93893908631701));
#13595=CARTESIAN_POINT('Ctrl Pts',(10.9368942686374,-0.872618815068493,
-3.00870833572371));
#13596=CARTESIAN_POINT('Ctrl Pts',(10.9810231968561,-0.440651309409201,
-3.10173886632448));
#13597=CARTESIAN_POINT('Ctrl Pts',(11.0030417882076,-0.220105537948483,
-3.12463783133899));
#13598=CARTESIAN_POINT('Ctrl Pts',(11.0250134745746,-1.56339628742952E-10,
-3.12449703075077));
#13599=CARTESIAN_POINT('Ctrl Pts',(11.3678714938544,6.18854804392756E-16,
-2.24999999959601));
#13600=CARTESIAN_POINT('Ctrl Pts',(11.3107025569102,3.98751462744629E-15,
-2.39581565162524));
#13601=CARTESIAN_POINT('Ctrl Pts',(11.2535336199657,4.2949048620429E-12,
-2.54163130365436));
#13602=CARTESIAN_POINT('Ctrl Pts',(11.13924761349,4.2949048620429E-12,-2.83313031417626));
#13603=CARTESIAN_POINT('Ctrl Pts',(11.0821305439588,2.00190131796994E-14,
-2.97881367266907));
#13604=CARTESIAN_POINT('Ctrl Pts',(11.0250134744288,2.11995977951848E-15,
-3.12449703116234));
#13605=CARTESIAN_POINT('Origin',(9.8,0.,-1.75));
#13606=CARTESIAN_POINT('',(10.78,-1.07231969947071E-7,-3.12449703081926));
#13607=CARTESIAN_POINT('Ctrl Pts',(11.0250134741351,-2.08166817117217E-16,
-3.12449703075067));
#13608=CARTESIAN_POINT('Ctrl Pts',(10.9841756494234,-2.08166817117217E-16,
-3.12449703075067));
#13609=CARTESIAN_POINT('Ctrl Pts',(10.9433378247117,-2.08166817117217E-16,
-3.12449703075067));
#13610=CARTESIAN_POINT('Ctrl Pts',(10.8616666666667,-2.08166817117217E-16,
-3.12449703075067));
#13611=CARTESIAN_POINT('Ctrl Pts',(10.8208333333333,-2.08166817117217E-16,
-3.12449703075067));
#13612=CARTESIAN_POINT('Ctrl Pts',(10.78,-2.08166817117217E-16,-3.12449703075067));
#13613=CARTESIAN_POINT('',(10.5350134750064,1.02273221749522E-10,-3.1244970310227));
#13614=CARTESIAN_POINT('Ctrl Pts',(10.78,-2.08166817117217E-16,-3.12449703075067));
#13615=CARTESIAN_POINT('Ctrl Pts',(10.7391666666667,-2.08166817117217E-16,
-3.12449703075067));
#13616=CARTESIAN_POINT('Ctrl Pts',(10.6983333333333,-2.08166817117217E-16,
-3.12449703075067));
#13617=CARTESIAN_POINT('Ctrl Pts',(10.6166711583355,-2.08166817117217E-16,
-3.12449703075067));
#13618=CARTESIAN_POINT('Ctrl Pts',(10.5758423166709,-2.08166817117217E-16,
-3.12449703075067));
#13619=CARTESIAN_POINT('Ctrl Pts',(10.5350134750064,-2.08166817117217E-16,
-3.12449703075067));
#13620=CARTESIAN_POINT('Ctrl Pts',(10.5350134747368,-3.00103482296057E-15,
-3.12449703112841));
#13621=CARTESIAN_POINT('Ctrl Pts',(10.4778952085294,-2.57860806401112E-14,
-2.97881062037814));
#13622=CARTESIAN_POINT('Ctrl Pts',(10.4207769423208,-5.52122510811137E-12,
-2.83312420962837));
#13623=CARTESIAN_POINT('Ctrl Pts',(10.3064909358382,-5.52122510811137E-12,
-2.54162519908909));
#13624=CARTESIAN_POINT('Ctrl Pts',(10.2493231955644,-4.57359866157433E-15,
-2.39581259929954));
#13625=CARTESIAN_POINT('Ctrl Pts',(10.1921554552908,6.1604094142004E-16,
-2.24999999950992));
#13626=CARTESIAN_POINT('Ctrl Pts',(5.553050567538,0.9783309087959,3.010992931911));
#13627=CARTESIAN_POINT('Ctrl Pts',(5.606133900872,0.4659514397387,3.177475113353));
#13628=CARTESIAN_POINT('Ctrl Pts',(5.712300567538,-0.6449686970874,3.242911847755));
#13629=CARTESIAN_POINT('Ctrl Pts',(5.871550567538,-2.147408477853,2.51427130483));
#13630=CARTESIAN_POINT('Ctrl Pts',(6.030800567538,-3.102099467523,1.144425205895));
#13631=CARTESIAN_POINT('Ctrl Pts',(6.190050567538,-3.265768497555,-0.5172460551353));
#13632=CARTESIAN_POINT('Ctrl Pts',(6.349300567538,-2.59663025113,-2.047018765263));
#13633=CARTESIAN_POINT('Ctrl Pts',(6.508550567538,-1.265333295377,-3.054784452443));
#13634=CARTESIAN_POINT('Ctrl Pts',(6.667800567538,0.3886344899198,-3.283555947824));
#13635=CARTESIAN_POINT('Ctrl Pts',(6.827050567538,1.943497179912,-2.674994390568));
#13636=CARTESIAN_POINT('Ctrl Pts',(6.986300567538,3.002752621272,-1.384287918735));
#13637=CARTESIAN_POINT('Ctrl Pts',(7.145550567538,3.296282150534,0.2594230316885));
#13638=CARTESIAN_POINT('Ctrl Pts',(7.304800567538,2.749233411565,1.836979036087));
#13639=CARTESIAN_POINT('Ctrl Pts',(7.464050567538,1.501108196656,2.946090716765));
#13640=CARTESIAN_POINT('Ctrl Pts',(7.623300567538,-0.1298115957604,3.303925737529));
#13641=CARTESIAN_POINT('Ctrl Pts',(7.782550567538,-1.727628394674,2.819233310576));
#13642=CARTESIAN_POINT('Ctrl Pts',(7.941800567538,-2.884886156338,1.615613875434));
#13643=CARTESIAN_POINT('Ctrl Pts',(8.101050567538,-3.30647490986,1.287858708565E-14));
#13644=CARTESIAN_POINT('Ctrl Pts',(8.260300567538,-2.884886156338,-1.615613875434));
#13645=CARTESIAN_POINT('Ctrl Pts',(8.419550567538,-1.727628394674,-2.819233310576));
#13646=CARTESIAN_POINT('Ctrl Pts',(8.578800567538,-0.1298115957604,-3.303925737529));
#13647=CARTESIAN_POINT('Ctrl Pts',(8.738050567538,1.501108196656,-2.946090716765));
#13648=CARTESIAN_POINT('Ctrl Pts',(8.897300567538,2.749233411565,-1.836979036087));
#13649=CARTESIAN_POINT('Ctrl Pts',(9.056550567538,3.296282150534,-0.2594230316885));
#13650=CARTESIAN_POINT('Ctrl Pts',(9.215800567538,3.002752621272,1.384287918735));
#13651=CARTESIAN_POINT('Ctrl Pts',(9.375050567538,1.943497179912,2.674994390568));
#13652=CARTESIAN_POINT('Ctrl Pts',(9.534300567538,0.3886344899198,3.283555947824));
#13653=CARTESIAN_POINT('Ctrl Pts',(9.693550567538,-1.265333295377,3.054784452443));
#13654=CARTESIAN_POINT('Ctrl Pts',(9.852800567538,-2.59663025113,2.047018765263));
#13655=CARTESIAN_POINT('Ctrl Pts',(10.01205056754,-3.265768497555,0.5172460551353));
#13656=CARTESIAN_POINT('Ctrl Pts',(10.17130056754,-3.102099467523,-1.144425205895));
#13657=CARTESIAN_POINT('Ctrl Pts',(10.33055056754,-2.147408477853,-2.51427130483));
#13658=CARTESIAN_POINT('Ctrl Pts',(10.48980056754,-0.6449686970875,-3.242911847755));
#13659=CARTESIAN_POINT('Ctrl Pts',(10.5959672342,0.4659514397387,-3.177475113353));
#13660=CARTESIAN_POINT('Ctrl Pts',(10.64905056754,0.9783309087958,-3.010992931911));
#13661=CARTESIAN_POINT('Ctrl Pts',(5.428016855846,0.8797657511871,2.707640568999));
#13662=CARTESIAN_POINT('Ctrl Pts',(5.481100189179,0.4190076330134,2.857349956793));
#13663=CARTESIAN_POINT('Ctrl Pts',(5.587266855846,-0.5799892093603,2.91619405267));
#13664=CARTESIAN_POINT('Ctrl Pts',(5.746516855846,-1.931060764449,2.260962792133));
#13665=CARTESIAN_POINT('Ctrl Pts',(5.905766855846,-2.789568277733,1.029126333319));
#13666=CARTESIAN_POINT('Ctrl Pts',(6.065016855846,-2.936747934286,-0.4651344040686));
#13667=CARTESIAN_POINT('Ctrl Pts',(6.224266855846,-2.335024216144,-1.840785142863));
#13668=CARTESIAN_POINT('Ctrl Pts',(6.383516855846,-1.137853140589,-2.747020169102));
#13669=CARTESIAN_POINT('Ctrl Pts',(6.542766855846,0.3494802330045,-2.952743329512));
#13670=CARTESIAN_POINT('Ctrl Pts',(6.702016855846,1.747693179314,-2.405493303218));
#13671=CARTESIAN_POINT('Ctrl Pts',(6.861266855846,2.700230455495,-1.244823290091));
#13672=CARTESIAN_POINT('Ctrl Pts',(7.020516855846,2.964187389171,0.2332866071149));
#13673=CARTESIAN_POINT('Ctrl Pts',(7.179766855846,2.472252870444,1.651906555408));
#13674=CARTESIAN_POINT('Ctrl Pts',(7.339016855846,1.34987412579,2.649277140482));
#13675=CARTESIAN_POINT('Ctrl Pts',(7.498266855846,-0.116733300594,2.971060897913));
#13676=CARTESIAN_POINT('Ctrl Pts',(7.657516855846,-1.553572803177,2.535200399938));
#13677=CARTESIAN_POINT('Ctrl Pts',(7.816766855846,-2.594238834326,1.452843554231));
#13678=CARTESIAN_POINT('Ctrl Pts',(7.976016855846,-2.973353245513,1.228623977058E-14));
#13679=CARTESIAN_POINT('Ctrl Pts',(8.135266855846,-2.594238834326,-1.452843554231));
#13680=CARTESIAN_POINT('Ctrl Pts',(8.294516855846,-1.553572803177,-2.535200399938));
#13681=CARTESIAN_POINT('Ctrl Pts',(8.453766855846,-0.1167333005941,-2.971060897913));
#13682=CARTESIAN_POINT('Ctrl Pts',(8.613016855846,1.34987412579,-2.649277140482));
#13683=CARTESIAN_POINT('Ctrl Pts',(8.772266855846,2.472252870444,-1.651906555408));
#13684=CARTESIAN_POINT('Ctrl Pts',(8.931516855846,2.964187389171,-0.2332866071149));
#13685=CARTESIAN_POINT('Ctrl Pts',(9.090766855846,2.700230455495,1.244823290091));
#13686=CARTESIAN_POINT('Ctrl Pts',(9.250016855846,1.747693179314,2.405493303218));
#13687=CARTESIAN_POINT('Ctrl Pts',(9.409266855846,0.3494802330045,2.952743329512));
#13688=CARTESIAN_POINT('Ctrl Pts',(9.568516855846,-1.137853140589,2.747020169102));
#13689=CARTESIAN_POINT('Ctrl Pts',(9.727766855846,-2.335024216144,1.840785142863));
#13690=CARTESIAN_POINT('Ctrl Pts',(9.887016855846,-2.936747934286,0.4651344040686));
#13691=CARTESIAN_POINT('Ctrl Pts',(10.04626685585,-2.789568277733,-1.029126333319));
#13692=CARTESIAN_POINT('Ctrl Pts',(10.20551685585,-1.931060764449,-2.260962792133));
#13693=CARTESIAN_POINT('Ctrl Pts',(10.36476685585,-0.5799892093604,-2.91619405267));
#13694=CARTESIAN_POINT('Ctrl Pts',(10.47093352251,0.4190076330134,-2.857349956793));
#13695=CARTESIAN_POINT('Ctrl Pts',(10.52401685585,0.8797657511871,-2.707640568999));
#13696=CARTESIAN_POINT('Ctrl Pts',(5.302983144154,0.7812005935783,2.404288206087));
#13697=CARTESIAN_POINT('Ctrl Pts',(5.356066477487,0.3720638262881,2.537224800233));
#13698=CARTESIAN_POINT('Ctrl Pts',(5.462233144154,-0.5150097216332,2.589476257585));
#13699=CARTESIAN_POINT('Ctrl Pts',(5.621483144154,-1.714713051046,2.007654279437));
#13700=CARTESIAN_POINT('Ctrl Pts',(5.780733144154,-2.477037087943,0.9138274607431));
#13701=CARTESIAN_POINT('Ctrl Pts',(5.939983144154,-2.607727371018,-0.4130227530019));
#13702=CARTESIAN_POINT('Ctrl Pts',(6.099233144154,-2.073418181158,-1.634551520464));
#13703=CARTESIAN_POINT('Ctrl Pts',(6.258483144154,-1.010372985802,-2.439255885761));
#13704=CARTESIAN_POINT('Ctrl Pts',(6.417733144154,0.3103259760892,-2.6219307112));
#13705=CARTESIAN_POINT('Ctrl Pts',(6.576983144154,1.551889178717,-2.135992215868));
#13706=CARTESIAN_POINT('Ctrl Pts',(6.736233144154,2.397708289717,-1.105358661447));
#13707=CARTESIAN_POINT('Ctrl Pts',(6.895483144154,2.632092627808,0.2071501825414));
#13708=CARTESIAN_POINT('Ctrl Pts',(7.054733144154,2.195272329322,1.466834074728));
#13709=CARTESIAN_POINT('Ctrl Pts',(7.213983144154,1.198640054924,2.3524635642));
#13710=CARTESIAN_POINT('Ctrl Pts',(7.373233144154,-0.1036550054277,2.638196058298));
#13711=CARTESIAN_POINT('Ctrl Pts',(7.532483144154,-1.37951721168,2.251167489299));
#13712=CARTESIAN_POINT('Ctrl Pts',(7.691733144154,-2.303591512314,1.290073233029));
#13713=CARTESIAN_POINT('Ctrl Pts',(7.850983144154,-2.640231581167,1.108429745068E-14));
#13714=CARTESIAN_POINT('Ctrl Pts',(8.010233144154,-2.303591512314,-1.290073233029));
#13715=CARTESIAN_POINT('Ctrl Pts',(8.169483144154,-1.37951721168,-2.251167489299));
#13716=CARTESIAN_POINT('Ctrl Pts',(8.328733144154,-0.1036550054277,-2.638196058298));
#13717=CARTESIAN_POINT('Ctrl Pts',(8.487983144154,1.198640054924,-2.3524635642));
#13718=CARTESIAN_POINT('Ctrl Pts',(8.647233144154,2.195272329322,-1.466834074728));
#13719=CARTESIAN_POINT('Ctrl Pts',(8.806483144154,2.632092627808,-0.2071501825414));
#13720=CARTESIAN_POINT('Ctrl Pts',(8.965733144154,2.397708289717,1.105358661447));
#13721=CARTESIAN_POINT('Ctrl Pts',(9.124983144154,1.551889178717,2.135992215868));
#13722=CARTESIAN_POINT('Ctrl Pts',(9.284233144154,0.3103259760892,2.6219307112));
#13723=CARTESIAN_POINT('Ctrl Pts',(9.443483144154,-1.010372985802,2.439255885761));
#13724=CARTESIAN_POINT('Ctrl Pts',(9.602733144154,-2.073418181158,1.634551520464));
#13725=CARTESIAN_POINT('Ctrl Pts',(9.761983144154,-2.607727371018,0.4130227530019));
#13726=CARTESIAN_POINT('Ctrl Pts',(9.921233144154,-2.477037087943,-0.913827460743));
#13727=CARTESIAN_POINT('Ctrl Pts',(10.08048314415,-1.714713051046,-2.007654279437));
#13728=CARTESIAN_POINT('Ctrl Pts',(10.23973314415,-0.5150097216332,-2.589476257585));
#13729=CARTESIAN_POINT('Ctrl Pts',(10.34589981082,0.3720638262881,-2.537224800233));
#13730=CARTESIAN_POINT('Ctrl Pts',(10.39898314415,0.7812005935783,-2.404288206087));
#13731=CARTESIAN_POINT('Ctrl Pts',(5.177949432462,0.6826354359695,2.100935843176));
#13732=CARTESIAN_POINT('Ctrl Pts',(5.231032765795,0.3251200195628,2.217099643673));
#13733=CARTESIAN_POINT('Ctrl Pts',(5.337199432462,-0.4500302339061,2.2627584625));
#13734=CARTESIAN_POINT('Ctrl Pts',(5.496449432462,-1.498365337642,1.754345766741));
#13735=CARTESIAN_POINT('Ctrl Pts',(5.655699432462,-2.164505898152,0.7985285881669));
#13736=CARTESIAN_POINT('Ctrl Pts',(5.814949432462,-2.278706807749,-0.3609111019352));
#13737=CARTESIAN_POINT('Ctrl Pts',(5.974199432462,-1.811812146172,-1.428317898065));
#13738=CARTESIAN_POINT('Ctrl Pts',(6.133449432462,-0.8828928310149,-2.13149160242));
#13739=CARTESIAN_POINT('Ctrl Pts',(6.292699432462,0.271171719174,-2.291118092888));
#13740=CARTESIAN_POINT('Ctrl Pts',(6.451949432462,1.35608517812,-1.866491128517));
#13741=CARTESIAN_POINT('Ctrl Pts',(6.611199432462,2.09518612394,-0.9658940328033));
#13742=CARTESIAN_POINT('Ctrl Pts',(6.770449432462,2.299997866445,0.1810137579678));
#13743=CARTESIAN_POINT('Ctrl Pts',(6.929699432462,1.918291788201,1.281761594049));
#13744=CARTESIAN_POINT('Ctrl Pts',(7.088949432462,1.047405984058,2.055649987917));
#13745=CARTESIAN_POINT('Ctrl Pts',(7.248199432462,-0.0905767102614,2.305331218682));
#13746=CARTESIAN_POINT('Ctrl Pts',(7.407449432462,-1.205461620183,1.967134578661));
#13747=CARTESIAN_POINT('Ctrl Pts',(7.566699432462,-2.012944190303,1.127302911826));
#13748=CARTESIAN_POINT('Ctrl Pts',(7.725949432462,-2.30710991682,0.));
#13749=CARTESIAN_POINT('Ctrl Pts',(7.885199432462,-2.012944190303,-1.127302911826));
#13750=CARTESIAN_POINT('Ctrl Pts',(8.044449432462,-1.205461620183,-1.967134578661));
#13751=CARTESIAN_POINT('Ctrl Pts',(8.203699432462,-0.09057671026141,-2.305331218682));
#13752=CARTESIAN_POINT('Ctrl Pts',(8.362949432462,1.047405984058,-2.055649987917));
#13753=CARTESIAN_POINT('Ctrl Pts',(8.522199432462,1.918291788201,-1.281761594049));
#13754=CARTESIAN_POINT('Ctrl Pts',(8.681449432462,2.299997866445,-0.1810137579678));
#13755=CARTESIAN_POINT('Ctrl Pts',(8.840699432462,2.09518612394,0.9658940328033));
#13756=CARTESIAN_POINT('Ctrl Pts',(8.999949432462,1.35608517812,1.866491128517));
#13757=CARTESIAN_POINT('Ctrl Pts',(9.159199432462,0.271171719174,2.291118092888));
#13758=CARTESIAN_POINT('Ctrl Pts',(9.318449432462,-0.8828928310149,2.13149160242));
#13759=CARTESIAN_POINT('Ctrl Pts',(9.477699432462,-1.811812146172,1.428317898065));
#13760=CARTESIAN_POINT('Ctrl Pts',(9.636949432462,-2.278706807749,0.3609111019352));
#13761=CARTESIAN_POINT('Ctrl Pts',(9.796199432462,-2.164505898152,-0.7985285881669));
#13762=CARTESIAN_POINT('Ctrl Pts',(9.955449432462,-1.498365337642,-1.754345766741));
#13763=CARTESIAN_POINT('Ctrl Pts',(10.11469943246,-0.4500302339061,-2.2627584625));
#13764=CARTESIAN_POINT('Ctrl Pts',(10.22086609913,0.3251200195628,-2.217099643673));
#13765=CARTESIAN_POINT('Ctrl Pts',(10.27394943246,0.6826354359695,-2.100935843176));
#13766=CARTESIAN_POINT('',(5.63499255472031,-7.41993575758981E-7,3.12499989450239));
#13767=CARTESIAN_POINT('Ctrl Pts',(5.634986107407,4.18742151866297E-6,3.12449702806922));
#13768=CARTESIAN_POINT('Ctrl Pts',(5.65695791239165,-0.220102539161386,
3.12463812164867));
#13769=CARTESIAN_POINT('Ctrl Pts',(5.67897662252065,-0.44064953200304,3.10173920341104));
#13770=CARTESIAN_POINT('Ctrl Pts',(5.72310569009851,-0.872618420486203,
3.00870846633561));
#13771=CARTESIAN_POINT('Ctrl Pts',(5.74514655866766,-1.08338856035468,2.93893917134752));
#13772=CARTESIAN_POINT('Ctrl Pts',(5.79629053209681,-1.55043320018977,2.72810358228179));
#13773=CARTESIAN_POINT('Ctrl Pts',(5.8377928382817,-1.92091911867348,2.51858797774256));
#13774=CARTESIAN_POINT('Ctrl Pts',(5.92921645078997,-2.54824617086085,1.8514803835448));
#13775=CARTESIAN_POINT('Ctrl Pts',(5.96919669615485,-2.76667000678542,1.50682910689432));
#13776=CARTESIAN_POINT('Ctrl Pts',(6.05240102883088,-3.06923750138772,0.73049620826951));
#13777=CARTESIAN_POINT('Ctrl Pts',(6.09319131879255,-3.13182588768285,0.318472133625857));
#13778=CARTESIAN_POINT('Ctrl Pts',(6.18384690093985,-3.11321199907849,-0.589454969171778));
#13779=CARTESIAN_POINT('Ctrl Pts',(6.22566769599382,-2.97612381593501,-0.996047824886898));
#13780=CARTESIAN_POINT('Ctrl Pts',(6.28566680271478,-2.7324562628559,-1.54560310783314));
#13781=CARTESIAN_POINT('Ctrl Pts',(6.32705708412113,-2.52230748364122,-1.91404302998656));
#13782=CARTESIAN_POINT('Ctrl Pts',(6.41557929492122,-1.87904024871203,-2.52442476815788));
#13783=CARTESIAN_POINT('Ctrl Pts',(6.4554980477788,-1.54078105288756,-2.75166775493571));
#13784=CARTESIAN_POINT('Ctrl Pts',(6.53843076181692,-0.768144592726403,
-3.05621103088525));
#13785=CARTESIAN_POINT('Ctrl Pts',(6.57908686746234,-0.359581070464692,
-3.13013165576389));
#13786=CARTESIAN_POINT('Ctrl Pts',(6.67176471540957,0.568604604224001,-3.11705696110184));
#13787=CARTESIAN_POINT('Ctrl Pts',(6.71373757339203,0.97756384079563,-2.98201038085689));
#13788=CARTESIAN_POINT('Ctrl Pts',(6.78430055630929,1.62585920990473,-2.69999321328485));
#13789=CARTESIAN_POINT('Ctrl Pts',(6.82487067374848,1.96613181358351,-2.46385086322353));
#13790=CARTESIAN_POINT('Ctrl Pts',(6.89543046710297,2.45553051679625,-1.95376212132779));
#13791=CARTESIAN_POINT('Ctrl Pts',(6.9367721787788,2.71875343764013,-1.62181272348741));
#13792=CARTESIAN_POINT('Ctrl Pts',(7.02751008605373,3.05336233804938,-0.776946962299042));
#13793=CARTESIAN_POINT('Ctrl Pts',(7.06791907246958,3.1286208842104,-0.371271841828463));
#13794=CARTESIAN_POINT('Ctrl Pts',(7.16122878779359,3.1195612174274,0.563189413652646));
#13795=CARTESIAN_POINT('Ctrl Pts',(7.20352621934902,2.98141015394773,0.975053271184048));
#13796=CARTESIAN_POINT('Ctrl Pts',(7.27288521992913,2.70782042248996,1.61380337445921));
#13797=CARTESIAN_POINT('Ctrl Pts',(7.31352769034975,2.47211612449969,1.95532520783703));
#13798=CARTESIAN_POINT('Ctrl Pts',(7.38355979919702,1.9681167518946,2.44349049201396));
#13799=CARTESIAN_POINT('Ctrl Pts',(7.42507806923627,1.63734153358997,2.7116624648552));
#13800=CARTESIAN_POINT('Ctrl Pts',(7.51669238599497,0.784710932292811,3.05077446246928));
#13801=CARTESIAN_POINT('Ctrl Pts',(7.55681070224769,0.382385740435282,3.12715191531059));
#13802=CARTESIAN_POINT('Ctrl Pts',(7.6420474933619,-0.471183768083625,3.12237996970145));
#13803=CARTESIAN_POINT('Ctrl Pts',(7.68300860642016,-0.877409231626726,
3.02091407068735));
#13804=CARTESIAN_POINT('Ctrl Pts',(7.7698414291264,-1.67903873524072,2.68319768942737));
#13805=CARTESIAN_POINT('Ctrl Pts',(7.81138319476979,-2.00874122018002,2.41423377541338));
#13806=CARTESIAN_POINT('Ctrl Pts',(7.87169428741273,-2.43162777346986,1.98258700351926));
#13807=CARTESIAN_POINT('Ctrl Pts',(7.91323523064669,-2.70311754303439,1.65387788875613));
#13808=CARTESIAN_POINT('Ctrl Pts',(8.00538249933744,-3.04697916736015,0.797280394573023));
#13809=CARTESIAN_POINT('Ctrl Pts',(8.04518829630558,-3.125,0.398671791438245));
#13810=CARTESIAN_POINT('Ctrl Pts',(8.12481170369442,-3.125,-0.398671791438237));
#13811=CARTESIAN_POINT('Ctrl Pts',(8.16461750066219,-3.04697916736015,-0.797280394573014));
#13812=CARTESIAN_POINT('Ctrl Pts',(8.25676476935278,-2.70311754303438,-1.65387788875615));
#13813=CARTESIAN_POINT('Ctrl Pts',(8.29830571258681,-2.43162777346985,-1.98258700351927));
#13814=CARTESIAN_POINT('Ctrl Pts',(8.35861680522996,-2.00874122018002,-2.41423377541338));
#13815=CARTESIAN_POINT('Ctrl Pts',(8.40015857087367,-1.67903873524071,-2.68319768942738));
#13816=CARTESIAN_POINT('Ctrl Pts',(8.48699139357988,-0.877409231626862,
-3.02091407068729));
#13817=CARTESIAN_POINT('Ctrl Pts',(8.52795250663794,-0.471183768083765,
-3.12237996970145));
#13818=CARTESIAN_POINT('Ctrl Pts',(8.61318929775226,0.382385740435305,-3.12715191531059));
#13819=CARTESIAN_POINT('Ctrl Pts',(8.65330761400518,0.78471093229284,-3.05077446246927));
#13820=CARTESIAN_POINT('Ctrl Pts',(8.74492193076395,1.63734153359001,-2.71166246485517));
#13821=CARTESIAN_POINT('Ctrl Pts',(8.78644020080312,1.96811675189465,-2.44349049201392));
#13822=CARTESIAN_POINT('Ctrl Pts',(8.85647230965024,2.47211612449972,-1.955325207837));
#13823=CARTESIAN_POINT('Ctrl Pts',(8.89711478007069,2.70782042248998,-1.61380337445918));
#13824=CARTESIAN_POINT('Ctrl Pts',(8.96647378065064,2.98141015394768,-0.975053271184154));
#13825=CARTESIAN_POINT('Ctrl Pts',(9.00877121220594,3.1195612174274,-0.563189413652753));
#13826=CARTESIAN_POINT('Ctrl Pts',(9.10208092752994,3.1286208842104,0.371271841828464));
#13827=CARTESIAN_POINT('Ctrl Pts',(9.14248991394583,3.05336233804938,0.776946962299041));
#13828=CARTESIAN_POINT('Ctrl Pts',(9.23322782122083,2.71875343764019,1.62181272348726));
#13829=CARTESIAN_POINT('Ctrl Pts',(9.27456953289673,2.45553051679638,1.95376212132765));
#13830=CARTESIAN_POINT('Ctrl Pts',(9.3451293262515,1.96613181358349,2.46385086322354));
#13831=CARTESIAN_POINT('Ctrl Pts',(9.38569944369098,1.6258592099047,2.69999321328487));
#13832=CARTESIAN_POINT('Ctrl Pts',(9.45626242660842,0.977563840795583,2.9820103808569));
#13833=CARTESIAN_POINT('Ctrl Pts',(9.49823528459103,0.568604604223939,3.11705696110185));
#13834=CARTESIAN_POINT('Ctrl Pts',(9.59091313253803,-0.35958107046477,3.13013165576388));
#13835=CARTESIAN_POINT('Ctrl Pts',(9.63156923818311,-0.768144592726469,
3.05621103088523));
#13836=CARTESIAN_POINT('Ctrl Pts',(9.71450195222103,-1.54078105288761,2.75166775493568));
#13837=CARTESIAN_POINT('Ctrl Pts',(9.75442070507848,-1.87904024871206,2.52442476815785));
#13838=CARTESIAN_POINT('Ctrl Pts',(9.84294291587878,-2.52230748364123,1.91404302998655));
#13839=CARTESIAN_POINT('Ctrl Pts',(9.88433319728545,-2.73245626285591,1.54560310783313));
#13840=CARTESIAN_POINT('Ctrl Pts',(9.94433230400693,-2.97612381593506,0.996047824886782));
#13841=CARTESIAN_POINT('Ctrl Pts',(9.98615309906173,-3.11321199907852,0.589454969171631));
#13842=CARTESIAN_POINT('Ctrl Pts',(10.0768086812096,-3.13182588768283,-0.318472133625934));
#13843=CARTESIAN_POINT('Ctrl Pts',(10.1175989711713,-3.06923750138772,-0.73049620826962));
#13844=CARTESIAN_POINT('Ctrl Pts',(10.2008033038473,-2.7666700067853,-1.50682910689455));
#13845=CARTESIAN_POINT('Ctrl Pts',(10.2407835492118,-2.54824617086069,-1.85148038354501));
#13846=CARTESIAN_POINT('Ctrl Pts',(10.33220716172,-1.92091911867334,-2.51858797774264));
#13847=CARTESIAN_POINT('Ctrl Pts',(10.3737094679055,-1.55043320018966,-2.72810358228187));
#13848=CARTESIAN_POINT('Ctrl Pts',(10.4248534244673,-1.08338871438423,-2.93893910181472));
#13849=CARTESIAN_POINT('Ctrl Pts',(10.446894276161,-0.872618743151924,-3.00870835952902));
#13850=CARTESIAN_POINT('Ctrl Pts',(10.4910232042645,-0.44065123519992,-3.10173887397661));
#13851=CARTESIAN_POINT('Ctrl Pts',(10.5130417918927,-0.220105501026149,
-3.12463783133622));
#13852=CARTESIAN_POINT('Ctrl Pts',(10.5350134746029,1.42376700706937E-10,
-3.12449703075058));
#13853=CARTESIAN_POINT('',(5.635,0.,3.125));
#13854=CARTESIAN_POINT('Ctrl Pts',(0.6530505675382,-0.9783309087958,-3.010992931911));
#13855=CARTESIAN_POINT('Ctrl Pts',(0.7061339008715,-0.4659514397387,-3.177475113353));
#13856=CARTESIAN_POINT('Ctrl Pts',(0.8123005675382,0.6449686970875,-3.242911847755));
#13857=CARTESIAN_POINT('Ctrl Pts',(0.9715505675382,2.147408477853,-2.51427130483));
#13858=CARTESIAN_POINT('Ctrl Pts',(1.130800567538,3.102099467523,-1.144425205895));
#13859=CARTESIAN_POINT('Ctrl Pts',(1.290050567538,3.265768497555,0.5172460551354));
#13860=CARTESIAN_POINT('Ctrl Pts',(1.449300567538,2.59663025113,2.047018765263));
#13861=CARTESIAN_POINT('Ctrl Pts',(1.608550567538,1.265333295377,3.054784452443));
#13862=CARTESIAN_POINT('Ctrl Pts',(1.767800567538,-0.3886344899198,3.283555947824));
#13863=CARTESIAN_POINT('Ctrl Pts',(1.927050567538,-1.943497179912,2.674994390568));
#13864=CARTESIAN_POINT('Ctrl Pts',(2.086300567538,-3.002752621272,1.384287918735));
#13865=CARTESIAN_POINT('Ctrl Pts',(2.245550567538,-3.296282150534,-0.2594230316885));
#13866=CARTESIAN_POINT('Ctrl Pts',(2.404800567538,-2.749233411565,-1.836979036087));
#13867=CARTESIAN_POINT('Ctrl Pts',(2.564050567538,-1.501108196656,-2.946090716765));
#13868=CARTESIAN_POINT('Ctrl Pts',(2.723300567538,0.1298115957604,-3.303925737529));
#13869=CARTESIAN_POINT('Ctrl Pts',(2.882550567538,1.727628394674,-2.819233310576));
#13870=CARTESIAN_POINT('Ctrl Pts',(3.041800567538,2.884886156338,-1.615613875434));
#13871=CARTESIAN_POINT('Ctrl Pts',(3.201050567538,3.30647490986,0.));
#13872=CARTESIAN_POINT('Ctrl Pts',(3.360300567538,2.884886156338,1.615613875434));
#13873=CARTESIAN_POINT('Ctrl Pts',(3.519550567538,1.727628394674,2.819233310576));
#13874=CARTESIAN_POINT('Ctrl Pts',(3.678800567538,0.1298115957604,3.303925737529));
#13875=CARTESIAN_POINT('Ctrl Pts',(3.838050567538,-1.501108196656,2.946090716765));
#13876=CARTESIAN_POINT('Ctrl Pts',(3.997300567538,-2.749233411565,1.836979036087));
#13877=CARTESIAN_POINT('Ctrl Pts',(4.156550567538,-3.296282150534,0.2594230316885));
#13878=CARTESIAN_POINT('Ctrl Pts',(4.315800567538,-3.002752621272,-1.384287918735));
#13879=CARTESIAN_POINT('Ctrl Pts',(4.475050567538,-1.943497179912,-2.674994390568));
#13880=CARTESIAN_POINT('Ctrl Pts',(4.634300567538,-0.3886344899198,-3.283555947824));
#13881=CARTESIAN_POINT('Ctrl Pts',(4.793550567538,1.265333295377,-3.054784452443));
#13882=CARTESIAN_POINT('Ctrl Pts',(4.952800567538,2.59663025113,-2.047018765263));
#13883=CARTESIAN_POINT('Ctrl Pts',(5.112050567538,3.265768497555,-0.5172460551353));
#13884=CARTESIAN_POINT('Ctrl Pts',(5.271300567538,3.102099467523,1.144425205895));
#13885=CARTESIAN_POINT('Ctrl Pts',(5.430550567538,2.147408477853,2.51427130483));
#13886=CARTESIAN_POINT('Ctrl Pts',(5.589800567538,0.6449686970875,3.242911847755));
#13887=CARTESIAN_POINT('Ctrl Pts',(5.695967234205,-0.4659514397387,3.177475113353));
#13888=CARTESIAN_POINT('Ctrl Pts',(5.749050567538,-0.9783309087958,3.010992931911));
#13889=CARTESIAN_POINT('Ctrl Pts',(0.5280168558461,-0.8797657511871,-2.707640568999));
#13890=CARTESIAN_POINT('Ctrl Pts',(0.5811001891794,-0.4190076330134,-2.857349956793));
#13891=CARTESIAN_POINT('Ctrl Pts',(0.6872668558461,0.5799892093603,-2.91619405267));
#13892=CARTESIAN_POINT('Ctrl Pts',(0.8465168558461,1.931060764449,-2.260962792133));
#13893=CARTESIAN_POINT('Ctrl Pts',(1.005766855846,2.789568277733,-1.029126333319));
#13894=CARTESIAN_POINT('Ctrl Pts',(1.165016855846,2.936747934286,0.4651344040687));
#13895=CARTESIAN_POINT('Ctrl Pts',(1.324266855846,2.335024216144,1.840785142863));
#13896=CARTESIAN_POINT('Ctrl Pts',(1.483516855846,1.137853140589,2.747020169102));
#13897=CARTESIAN_POINT('Ctrl Pts',(1.642766855846,-0.3494802330045,2.952743329512));
#13898=CARTESIAN_POINT('Ctrl Pts',(1.802016855846,-1.747693179314,2.405493303218));
#13899=CARTESIAN_POINT('Ctrl Pts',(1.961266855846,-2.700230455495,1.244823290091));
#13900=CARTESIAN_POINT('Ctrl Pts',(2.120516855846,-2.964187389171,-0.2332866071149));
#13901=CARTESIAN_POINT('Ctrl Pts',(2.279766855846,-2.472252870444,-1.651906555408));
#13902=CARTESIAN_POINT('Ctrl Pts',(2.439016855846,-1.34987412579,-2.649277140482));
#13903=CARTESIAN_POINT('Ctrl Pts',(2.598266855846,0.1167333005941,-2.971060897913));
#13904=CARTESIAN_POINT('Ctrl Pts',(2.757516855846,1.553572803177,-2.535200399938));
#13905=CARTESIAN_POINT('Ctrl Pts',(2.916766855846,2.594238834326,-1.452843554231));
#13906=CARTESIAN_POINT('Ctrl Pts',(3.076016855846,2.973353245513,0.));
#13907=CARTESIAN_POINT('Ctrl Pts',(3.235266855846,2.594238834326,1.452843554231));
#13908=CARTESIAN_POINT('Ctrl Pts',(3.394516855846,1.553572803177,2.535200399938));
#13909=CARTESIAN_POINT('Ctrl Pts',(3.553766855846,0.1167333005941,2.971060897913));
#13910=CARTESIAN_POINT('Ctrl Pts',(3.713016855846,-1.34987412579,2.649277140482));
#13911=CARTESIAN_POINT('Ctrl Pts',(3.872266855846,-2.472252870444,1.651906555408));
#13912=CARTESIAN_POINT('Ctrl Pts',(4.031516855846,-2.964187389171,0.2332866071149));
#13913=CARTESIAN_POINT('Ctrl Pts',(4.190766855846,-2.700230455495,-1.244823290091));
#13914=CARTESIAN_POINT('Ctrl Pts',(4.350016855846,-1.747693179314,-2.405493303218));
#13915=CARTESIAN_POINT('Ctrl Pts',(4.509266855846,-0.3494802330045,-2.952743329512));
#13916=CARTESIAN_POINT('Ctrl Pts',(4.668516855846,1.137853140589,-2.747020169102));
#13917=CARTESIAN_POINT('Ctrl Pts',(4.827766855846,2.335024216144,-1.840785142863));
#13918=CARTESIAN_POINT('Ctrl Pts',(4.987016855846,2.936747934286,-0.4651344040686));
#13919=CARTESIAN_POINT('Ctrl Pts',(5.146266855846,2.789568277733,1.029126333319));
#13920=CARTESIAN_POINT('Ctrl Pts',(5.305516855846,1.931060764449,2.260962792133));
#13921=CARTESIAN_POINT('Ctrl Pts',(5.464766855846,0.5799892093604,2.91619405267));
#13922=CARTESIAN_POINT('Ctrl Pts',(5.570933522513,-0.4190076330134,2.857349956793));
#13923=CARTESIAN_POINT('Ctrl Pts',(5.624016855846,-0.8797657511871,2.707640568999));
#13924=CARTESIAN_POINT('Ctrl Pts',(0.4029831441539,-0.7812005935783,-2.404288206087));
#13925=CARTESIAN_POINT('Ctrl Pts',(0.4560664774873,-0.3720638262881,-2.537224800233));
#13926=CARTESIAN_POINT('Ctrl Pts',(0.5622331441539,0.5150097216332,-2.589476257585));
#13927=CARTESIAN_POINT('Ctrl Pts',(0.7214831441539,1.714713051046,-2.007654279437));
#13928=CARTESIAN_POINT('Ctrl Pts',(0.8807331441539,2.477037087943,-0.9138274607431));
#13929=CARTESIAN_POINT('Ctrl Pts',(1.039983144154,2.607727371018,0.413022753002));
#13930=CARTESIAN_POINT('Ctrl Pts',(1.199233144154,2.073418181158,1.634551520464));
#13931=CARTESIAN_POINT('Ctrl Pts',(1.358483144154,1.010372985802,2.439255885761));
#13932=CARTESIAN_POINT('Ctrl Pts',(1.517733144154,-0.3103259760893,2.6219307112));
#13933=CARTESIAN_POINT('Ctrl Pts',(1.676983144154,-1.551889178717,2.135992215868));
#13934=CARTESIAN_POINT('Ctrl Pts',(1.836233144154,-2.397708289717,1.105358661447));
#13935=CARTESIAN_POINT('Ctrl Pts',(1.995483144154,-2.632092627808,-0.2071501825414));
#13936=CARTESIAN_POINT('Ctrl Pts',(2.154733144154,-2.195272329322,-1.466834074728));
#13937=CARTESIAN_POINT('Ctrl Pts',(2.313983144154,-1.198640054924,-2.3524635642));
#13938=CARTESIAN_POINT('Ctrl Pts',(2.473233144154,0.1036550054277,-2.638196058298));
#13939=CARTESIAN_POINT('Ctrl Pts',(2.632483144154,1.37951721168,-2.251167489299));
#13940=CARTESIAN_POINT('Ctrl Pts',(2.791733144154,2.303591512314,-1.290073233029));
#13941=CARTESIAN_POINT('Ctrl Pts',(2.950983144154,2.640231581167,0.));
#13942=CARTESIAN_POINT('Ctrl Pts',(3.110233144154,2.303591512314,1.290073233029));
#13943=CARTESIAN_POINT('Ctrl Pts',(3.269483144154,1.37951721168,2.251167489299));
#13944=CARTESIAN_POINT('Ctrl Pts',(3.428733144154,0.1036550054277,2.638196058298));
#13945=CARTESIAN_POINT('Ctrl Pts',(3.587983144154,-1.198640054924,2.3524635642));
#13946=CARTESIAN_POINT('Ctrl Pts',(3.747233144154,-2.195272329322,1.466834074728));
#13947=CARTESIAN_POINT('Ctrl Pts',(3.906483144154,-2.632092627808,0.2071501825414));
#13948=CARTESIAN_POINT('Ctrl Pts',(4.065733144154,-2.397708289717,-1.105358661447));
#13949=CARTESIAN_POINT('Ctrl Pts',(4.224983144154,-1.551889178717,-2.135992215868));
#13950=CARTESIAN_POINT('Ctrl Pts',(4.384233144154,-0.3103259760893,-2.6219307112));
#13951=CARTESIAN_POINT('Ctrl Pts',(4.543483144154,1.010372985802,-2.439255885761));
#13952=CARTESIAN_POINT('Ctrl Pts',(4.702733144154,2.073418181158,-1.634551520464));
#13953=CARTESIAN_POINT('Ctrl Pts',(4.861983144154,2.607727371018,-0.4130227530019));
#13954=CARTESIAN_POINT('Ctrl Pts',(5.021233144154,2.477037087943,0.913827460743));
#13955=CARTESIAN_POINT('Ctrl Pts',(5.180483144154,1.714713051046,2.007654279437));
#13956=CARTESIAN_POINT('Ctrl Pts',(5.339733144154,0.5150097216332,2.589476257585));
#13957=CARTESIAN_POINT('Ctrl Pts',(5.445899810821,-0.3720638262881,2.537224800233));
#13958=CARTESIAN_POINT('Ctrl Pts',(5.498983144154,-0.7812005935783,2.404288206087));
#13959=CARTESIAN_POINT('Ctrl Pts',(0.2779494324618,-0.6826354359695,-2.100935843176));
#13960=CARTESIAN_POINT('Ctrl Pts',(0.3310327657952,-0.3251200195628,-2.217099643673));
#13961=CARTESIAN_POINT('Ctrl Pts',(0.4371994324618,0.4500302339061,-2.2627584625));
#13962=CARTESIAN_POINT('Ctrl Pts',(0.5964494324618,1.498365337642,-1.754345766741));
#13963=CARTESIAN_POINT('Ctrl Pts',(0.7556994324618,2.164505898152,-0.7985285881669));
#13964=CARTESIAN_POINT('Ctrl Pts',(0.9149494324618,2.278706807749,0.3609111019353));
#13965=CARTESIAN_POINT('Ctrl Pts',(1.074199432462,1.811812146172,1.428317898065));
#13966=CARTESIAN_POINT('Ctrl Pts',(1.233449432462,0.8828928310149,2.13149160242));
#13967=CARTESIAN_POINT('Ctrl Pts',(1.392699432462,-0.271171719174,2.291118092888));
#13968=CARTESIAN_POINT('Ctrl Pts',(1.551949432462,-1.35608517812,1.866491128517));
#13969=CARTESIAN_POINT('Ctrl Pts',(1.711199432462,-2.09518612394,0.9658940328033));
#13970=CARTESIAN_POINT('Ctrl Pts',(1.870449432462,-2.299997866445,-0.1810137579678));
#13971=CARTESIAN_POINT('Ctrl Pts',(2.029699432462,-1.918291788201,-1.281761594049));
#13972=CARTESIAN_POINT('Ctrl Pts',(2.188949432462,-1.047405984058,-2.055649987917));
#13973=CARTESIAN_POINT('Ctrl Pts',(2.348199432462,0.09057671026141,-2.305331218682));
#13974=CARTESIAN_POINT('Ctrl Pts',(2.507449432462,1.205461620183,-1.967134578661));
#13975=CARTESIAN_POINT('Ctrl Pts',(2.666699432462,2.012944190303,-1.127302911826));
#13976=CARTESIAN_POINT('Ctrl Pts',(2.825949432462,2.30710991682,0.));
#13977=CARTESIAN_POINT('Ctrl Pts',(2.985199432462,2.012944190303,1.127302911826));
#13978=CARTESIAN_POINT('Ctrl Pts',(3.144449432462,1.205461620183,1.967134578661));
#13979=CARTESIAN_POINT('Ctrl Pts',(3.303699432462,0.09057671026142,2.305331218682));
#13980=CARTESIAN_POINT('Ctrl Pts',(3.462949432462,-1.047405984058,2.055649987917));
#13981=CARTESIAN_POINT('Ctrl Pts',(3.622199432462,-1.918291788201,1.281761594049));
#13982=CARTESIAN_POINT('Ctrl Pts',(3.781449432462,-2.299997866445,0.1810137579678));
#13983=CARTESIAN_POINT('Ctrl Pts',(3.940699432462,-2.09518612394,-0.9658940328033));
#13984=CARTESIAN_POINT('Ctrl Pts',(4.099949432462,-1.35608517812,-1.866491128517));
#13985=CARTESIAN_POINT('Ctrl Pts',(4.259199432462,-0.271171719174,-2.291118092888));
#13986=CARTESIAN_POINT('Ctrl Pts',(4.418449432462,0.8828928310149,-2.13149160242));
#13987=CARTESIAN_POINT('Ctrl Pts',(4.577699432462,1.811812146172,-1.428317898065));
#13988=CARTESIAN_POINT('Ctrl Pts',(4.736949432462,2.278706807749,-0.3609111019352));
#13989=CARTESIAN_POINT('Ctrl Pts',(4.896199432462,2.164505898152,0.7985285881669));
#13990=CARTESIAN_POINT('Ctrl Pts',(5.055449432462,1.498365337642,1.754345766741));
#13991=CARTESIAN_POINT('Ctrl Pts',(5.214699432462,0.4500302339061,2.2627584625));
#13992=CARTESIAN_POINT('Ctrl Pts',(5.320866099128,-0.3251200195628,2.217099643673));
#13993=CARTESIAN_POINT('Ctrl Pts',(5.373949432462,-0.6826354359695,2.100935843176));
#13994=CARTESIAN_POINT('Ctrl Pts',(0.734986525425182,1.56341571633245E-10,
-3.12449703075077));
#13995=CARTESIAN_POINT('Ctrl Pts',(0.756958211791874,0.220105537948462,
-3.12463783133899));
#13996=CARTESIAN_POINT('Ctrl Pts',(0.77897680314279,0.440651309409153,-3.10173886632448));
#13997=CARTESIAN_POINT('Ctrl Pts',(0.823105731360934,0.872618815068403,
-3.00870833572373));
#13998=CARTESIAN_POINT('Ctrl Pts',(0.845146579294268,1.08338874871482,-2.93893908631705));
#13999=CARTESIAN_POINT('Ctrl Pts',(0.896290532096981,1.55043320018977,-2.72810358228179));
#14000=CARTESIAN_POINT('Ctrl Pts',(0.937792838281873,1.92091911867349,-2.51858797774255));
#14001=CARTESIAN_POINT('Ctrl Pts',(1.02921645079008,2.54824617086085,-1.85148038354479));
#14002=CARTESIAN_POINT('Ctrl Pts',(1.06919669615493,2.76667000678543,-1.50682910689431));
#14003=CARTESIAN_POINT('Ctrl Pts',(1.1524010288309,3.06923750138774,-0.730496208269469));
#14004=CARTESIAN_POINT('Ctrl Pts',(1.19319131879256,3.13182588768285,-0.318472133625813));
#14005=CARTESIAN_POINT('Ctrl Pts',(1.28384690093984,3.11321199907849,0.589454969171711));
#14006=CARTESIAN_POINT('Ctrl Pts',(1.32566769599381,2.97612381593505,0.996047824886831));
#14007=CARTESIAN_POINT('Ctrl Pts',(1.38566680271478,2.73245626285591,1.54560310783312));
#14008=CARTESIAN_POINT('Ctrl Pts',(1.42705708412114,2.52230748364124,1.91404302998655));
#14009=CARTESIAN_POINT('Ctrl Pts',(1.51557929492124,1.879040248712,2.5244247681579));
#14010=CARTESIAN_POINT('Ctrl Pts',(1.55549804777882,1.54078105288753,2.75166775493572));
#14011=CARTESIAN_POINT('Ctrl Pts',(1.63843076181693,0.768144592726395,3.05621103088525));
#14012=CARTESIAN_POINT('Ctrl Pts',(1.67908686746235,0.359581070464684,3.13013165576389));
#14013=CARTESIAN_POINT('Ctrl Pts',(1.77176471540958,-0.56860460422401,3.11705696110184));
#14014=CARTESIAN_POINT('Ctrl Pts',(1.81373757339203,-0.977563840795641,
2.98201038085689));
#14015=CARTESIAN_POINT('Ctrl Pts',(1.8843005563093,-1.62585920990474,2.69999321328485));
#14016=CARTESIAN_POINT('Ctrl Pts',(1.92487067374849,-1.96613181358352,2.46385086322352));
#14017=CARTESIAN_POINT('Ctrl Pts',(1.99543046710298,-2.45553051679632,1.95376212132772));
#14018=CARTESIAN_POINT('Ctrl Pts',(2.03677217877881,-2.71875343764016,1.62181272348734));
#14019=CARTESIAN_POINT('Ctrl Pts',(2.12751008605373,-3.05336233804938,0.776946962299037));
#14020=CARTESIAN_POINT('Ctrl Pts',(2.16791907246958,-3.1286208842104,0.371271841828459));
#14021=CARTESIAN_POINT('Ctrl Pts',(2.2612287877936,-3.1195612174274,-0.563189413652693));
#14022=CARTESIAN_POINT('Ctrl Pts',(2.30352621934903,-2.98141015394771,-0.975053271184097));
#14023=CARTESIAN_POINT('Ctrl Pts',(2.37288521992913,-2.70782042248996,-1.61380337445921));
#14024=CARTESIAN_POINT('Ctrl Pts',(2.41352769034975,-2.47211612449969,-1.95532520783703));
#14025=CARTESIAN_POINT('Ctrl Pts',(2.48355979919702,-1.9681167518946,-2.44349049201396));
#14026=CARTESIAN_POINT('Ctrl Pts',(2.52507806923627,-1.63734153358997,-2.7116624648552));
#14027=CARTESIAN_POINT('Ctrl Pts',(2.61669238599497,-0.784710932292806,
-3.05077446246928));
#14028=CARTESIAN_POINT('Ctrl Pts',(2.65681070224768,-0.382385740435277,
-3.12715191531059));
#14029=CARTESIAN_POINT('Ctrl Pts',(2.74204749336189,0.471183768083628,-3.12237996970145));
#14030=CARTESIAN_POINT('Ctrl Pts',(2.78300860642015,0.877409231626729,-3.02091407068735));
#14031=CARTESIAN_POINT('Ctrl Pts',(2.8698414291264,1.67903873524071,-2.68319768942737));
#14032=CARTESIAN_POINT('Ctrl Pts',(2.91138319476978,2.00874122018001,-2.41423377541338));
#14033=CARTESIAN_POINT('Ctrl Pts',(2.97169428741273,2.43162777346987,-1.98258700351926));
#14034=CARTESIAN_POINT('Ctrl Pts',(3.01323523064669,2.70311754303439,-1.65387788875612));
#14035=CARTESIAN_POINT('Ctrl Pts',(3.10538249933744,3.04697916736015,-0.797280394573023));
#14036=CARTESIAN_POINT('Ctrl Pts',(3.14518829630558,3.125,-0.398671791438245));
#14037=CARTESIAN_POINT('Ctrl Pts',(3.22481170369442,3.125,0.398671791438237));
#14038=CARTESIAN_POINT('Ctrl Pts',(3.26461750066218,3.04697916736015,0.797280394573014));
#14039=CARTESIAN_POINT('Ctrl Pts',(3.35676476935278,2.70311754303438,1.65387788875616));
#14040=CARTESIAN_POINT('Ctrl Pts',(3.39830571258681,2.43162777346985,1.98258700351928));
#14041=CARTESIAN_POINT('Ctrl Pts',(3.45861680522996,2.00874122018001,2.41423377541339));
#14042=CARTESIAN_POINT('Ctrl Pts',(3.50015857087367,1.6790387352407,2.68319768942739));
#14043=CARTESIAN_POINT('Ctrl Pts',(3.58699139357987,0.877409231626872,3.02091407068728));
#14044=CARTESIAN_POINT('Ctrl Pts',(3.62795250663793,0.471183768083777,3.12237996970145));
#14045=CARTESIAN_POINT('Ctrl Pts',(3.71318929775225,-0.3823857404353,3.12715191531059));
#14046=CARTESIAN_POINT('Ctrl Pts',(3.75330761400518,-0.784710932292834,
3.05077446246928));
#14047=CARTESIAN_POINT('Ctrl Pts',(3.84492193076394,-1.63734153359002,2.71166246485517));
#14048=CARTESIAN_POINT('Ctrl Pts',(3.88644020080312,-1.96811675189465,2.44349049201392));
#14049=CARTESIAN_POINT('Ctrl Pts',(3.95647230965024,-2.47211612449971,1.955325207837));
#14050=CARTESIAN_POINT('Ctrl Pts',(3.99711478007069,-2.70782042248997,1.61380337445918));
#14051=CARTESIAN_POINT('Ctrl Pts',(4.06647378065064,-2.98141015394767,0.975053271184186));
#14052=CARTESIAN_POINT('Ctrl Pts',(4.10877121220594,-3.1195612174274,0.563189413652785));
#14053=CARTESIAN_POINT('Ctrl Pts',(4.20208092752994,-3.1286208842104,-0.371271841828458));
#14054=CARTESIAN_POINT('Ctrl Pts',(4.24248991394583,-3.05336233804938,-0.776946962299035));
#14055=CARTESIAN_POINT('Ctrl Pts',(4.33322782122083,-2.71875343764019,-1.62181272348727));
#14056=CARTESIAN_POINT('Ctrl Pts',(4.37456953289673,-2.45553051679637,-1.95376212132766));
#14057=CARTESIAN_POINT('Ctrl Pts',(4.44512932625149,-1.9661318135835,-2.46385086322354));
#14058=CARTESIAN_POINT('Ctrl Pts',(4.48569944369097,-1.62585920990471,-2.69999321328487));
#14059=CARTESIAN_POINT('Ctrl Pts',(4.55626242660842,-0.97756384079559,-2.9820103808569));
#14060=CARTESIAN_POINT('Ctrl Pts',(4.59823528459102,-0.568604604223948,
-3.11705696110185));
#14061=CARTESIAN_POINT('Ctrl Pts',(4.69091313253802,0.35958107046476,-3.13013165576389));
#14062=CARTESIAN_POINT('Ctrl Pts',(4.73156923818309,0.76814459272646,-3.05621103088524));
#14063=CARTESIAN_POINT('Ctrl Pts',(4.81450195222101,1.5407810528876,-2.75166775493569));
#14064=CARTESIAN_POINT('Ctrl Pts',(4.85442070507863,1.87904024871205,-2.52442476815786));
#14065=CARTESIAN_POINT('Ctrl Pts',(4.94294291587866,2.52230748364104,-1.91404302998674));
#14066=CARTESIAN_POINT('Ctrl Pts',(4.98433319728502,2.7324562628558,-1.54560310783341));
#14067=CARTESIAN_POINT('Ctrl Pts',(5.04433230400602,2.97612381593511,-0.996047824886731));
#14068=CARTESIAN_POINT('Ctrl Pts',(5.08615309905995,3.1132119990785,-0.589454969171663));
#14069=CARTESIAN_POINT('Ctrl Pts',(5.17680868120734,3.13182588768285,0.318472133625777));
#14070=CARTESIAN_POINT('Ctrl Pts',(5.21759897116921,3.06923750138774,0.730496208269473));
#14071=CARTESIAN_POINT('Ctrl Pts',(5.30080330384511,2.7666700067854,1.50682910689435));
#14072=CARTESIAN_POINT('Ctrl Pts',(5.3407835492096,2.54824617086083,1.85148038354482));
#14073=CARTESIAN_POINT('Ctrl Pts',(5.43220716171777,1.92091911867348,2.51858797774255));
#14074=CARTESIAN_POINT('Ctrl Pts',(5.47370946790287,1.55043320018978,2.72810358228179));
#14075=CARTESIAN_POINT('Ctrl Pts',(5.52485344133227,1.08338856035471,2.9389391713475));
#14076=CARTESIAN_POINT('Ctrl Pts',(5.54689430990158,0.87261842048627,3.00870846633559));
#14077=CARTESIAN_POINT('Ctrl Pts',(5.59102300077564,0.440653219467686,3.1017384092623));
#14078=CARTESIAN_POINT('Ctrl Pts',(5.61304133631232,0.220110064033209,3.12463734035084));
#14079=CARTESIAN_POINT('Ctrl Pts',(5.63501276810388,7.07736163903239E-6,
3.12449703527009));
#14080=CARTESIAN_POINT('Ctrl Pts',(0.9259788629516,-0.9656781074217,-2.972051613422));
#14081=CARTESIAN_POINT('Ctrl Pts',(0.979062196285,-0.4599252670358,-3.136380672689));
#14082=CARTESIAN_POINT('Ctrl Pts',(1.085228862952,0.6366272854614,-3.200971110614));
#14083=CARTESIAN_POINT('Ctrl Pts',(1.244478862952,2.119635939241,-2.481754111378));
#14084=CARTESIAN_POINT('Ctrl Pts',(1.403728862952,3.061979863765,-1.129624298873));
#14085=CARTESIAN_POINT('Ctrl Pts',(1.562978862952,3.223532154246,0.5105564866689));
#14086=CARTESIAN_POINT('Ctrl Pts',(1.722228862952,2.563047905408,2.020544571702));
#14087=CARTESIAN_POINT('Ctrl Pts',(1.881478862952,1.248968678135,3.015276776083));
#14088=CARTESIAN_POINT('Ctrl Pts',(2.040728862952,-0.383608261101,3.241089558554));
#14089=CARTESIAN_POINT('Ctrl Pts',(2.199978862952,-1.918361836065,2.640398557608));
#14090=CARTESIAN_POINT('Ctrl Pts',(2.359228862952,-2.963917875123,1.366384855545));
#14091=CARTESIAN_POINT('Ctrl Pts',(2.518478862952,-3.253651172662,-0.256067900963));
#14092=CARTESIAN_POINT('Ctrl Pts',(2.677728862952,-2.713677441724,-1.813221296591));
#14093=CARTESIAN_POINT('Ctrl Pts',(2.836978862952,-1.481694291113,-2.907988781792));
#14094=CARTESIAN_POINT('Ctrl Pts',(2.996228862952,0.1281327360592,-3.261195904774));
#14095=CARTESIAN_POINT('Ctrl Pts',(3.155478862952,1.705284892359,-2.782772028626));
#14096=CARTESIAN_POINT('Ctrl Pts',(3.314728862952,2.84757578293,-1.59471906236));
#14097=CARTESIAN_POINT('Ctrl Pts',(3.473978862952,3.263712108535,0.));
#14098=CARTESIAN_POINT('Ctrl Pts',(3.633228862952,2.84757578293,1.59471906236));
#14099=CARTESIAN_POINT('Ctrl Pts',(3.792478862952,1.705284892359,2.782772028626));
#14100=CARTESIAN_POINT('Ctrl Pts',(3.951728862952,0.1281327360592,3.261195904774));
#14101=CARTESIAN_POINT('Ctrl Pts',(4.110978862952,-1.481694291113,2.907988781792));
#14102=CARTESIAN_POINT('Ctrl Pts',(4.270228862952,-2.713677441724,1.813221296591));
#14103=CARTESIAN_POINT('Ctrl Pts',(4.429478862952,-3.253651172662,0.256067900963));
#14104=CARTESIAN_POINT('Ctrl Pts',(4.588728862952,-2.963917875123,-1.366384855545));
#14105=CARTESIAN_POINT('Ctrl Pts',(4.747978862952,-1.918361836065,-2.640398557608));
#14106=CARTESIAN_POINT('Ctrl Pts',(4.907228862952,-0.383608261101,-3.241089558554));
#14107=CARTESIAN_POINT('Ctrl Pts',(5.066478862952,1.248968678135,-3.015276776083));
#14108=CARTESIAN_POINT('Ctrl Pts',(5.225728862952,2.563047905408,-2.020544571702));
#14109=CARTESIAN_POINT('Ctrl Pts',(5.384978862952,3.223532154246,-0.510556486669));
#14110=CARTESIAN_POINT('Ctrl Pts',(5.544228862952,3.061979863765,1.129624298873));
#14111=CARTESIAN_POINT('Ctrl Pts',(5.703478862952,2.119635939241,2.481754111378));
#14112=CARTESIAN_POINT('Ctrl Pts',(5.862728862952,0.6366272854614,3.200971110614));
#14113=CARTESIAN_POINT('Ctrl Pts',(5.968895529618,-0.4599252670358,3.136380672689));
#14114=CARTESIAN_POINT('Ctrl Pts',(6.021978862952,-0.9656781074217,2.972051613422));
#14115=CARTESIAN_POINT('Ctrl Pts',(0.8149929543172,-0.9656781074217,-2.972051613422));
#14116=CARTESIAN_POINT('Ctrl Pts',(0.8680762876505,-0.4599252670358,-3.136380672689));
#14117=CARTESIAN_POINT('Ctrl Pts',(0.9742429543172,0.6366272854614,-3.200971110614));
#14118=CARTESIAN_POINT('Ctrl Pts',(1.133492954317,2.119635939241,-2.481754111378));
#14119=CARTESIAN_POINT('Ctrl Pts',(1.292742954317,3.061979863765,-1.129624298873));
#14120=CARTESIAN_POINT('Ctrl Pts',(1.451992954317,3.223532154246,0.5105564866689));
#14121=CARTESIAN_POINT('Ctrl Pts',(1.611242954317,2.563047905408,2.020544571702));
#14122=CARTESIAN_POINT('Ctrl Pts',(1.770492954317,1.248968678135,3.015276776083));
#14123=CARTESIAN_POINT('Ctrl Pts',(1.929742954317,-0.383608261101,3.241089558554));
#14124=CARTESIAN_POINT('Ctrl Pts',(2.088992954317,-1.918361836065,2.640398557608));
#14125=CARTESIAN_POINT('Ctrl Pts',(2.248242954317,-2.963917875123,1.366384855545));
#14126=CARTESIAN_POINT('Ctrl Pts',(2.407492954317,-3.253651172662,-0.256067900963));
#14127=CARTESIAN_POINT('Ctrl Pts',(2.566742954317,-2.713677441724,-1.813221296591));
#14128=CARTESIAN_POINT('Ctrl Pts',(2.725992954317,-1.481694291113,-2.907988781792));
#14129=CARTESIAN_POINT('Ctrl Pts',(2.885242954317,0.1281327360592,-3.261195904774));
#14130=CARTESIAN_POINT('Ctrl Pts',(3.044492954317,1.705284892359,-2.782772028626));
#14131=CARTESIAN_POINT('Ctrl Pts',(3.203742954317,2.84757578293,-1.59471906236));
#14132=CARTESIAN_POINT('Ctrl Pts',(3.362992954317,3.263712108535,0.));
#14133=CARTESIAN_POINT('Ctrl Pts',(3.522242954317,2.84757578293,1.59471906236));
#14134=CARTESIAN_POINT('Ctrl Pts',(3.681492954317,1.705284892359,2.782772028626));
#14135=CARTESIAN_POINT('Ctrl Pts',(3.840742954317,0.1281327360592,3.261195904774));
#14136=CARTESIAN_POINT('Ctrl Pts',(3.999992954317,-1.481694291113,2.907988781792));
#14137=CARTESIAN_POINT('Ctrl Pts',(4.159242954317,-2.713677441724,1.813221296591));
#14138=CARTESIAN_POINT('Ctrl Pts',(4.318492954317,-3.253651172662,0.256067900963));
#14139=CARTESIAN_POINT('Ctrl Pts',(4.477742954317,-2.963917875123,-1.366384855545));
#14140=CARTESIAN_POINT('Ctrl Pts',(4.636992954317,-1.918361836065,-2.640398557608));
#14141=CARTESIAN_POINT('Ctrl Pts',(4.796242954317,-0.383608261101,-3.241089558554));
#14142=CARTESIAN_POINT('Ctrl Pts',(4.955492954317,1.248968678135,-3.015276776083));
#14143=CARTESIAN_POINT('Ctrl Pts',(5.114742954317,2.563047905408,-2.020544571702));
#14144=CARTESIAN_POINT('Ctrl Pts',(5.273992954317,3.223532154246,-0.510556486669));
#14145=CARTESIAN_POINT('Ctrl Pts',(5.433242954317,3.061979863765,1.129624298873));
#14146=CARTESIAN_POINT('Ctrl Pts',(5.592492954317,2.119635939241,2.481754111378));
#14147=CARTESIAN_POINT('Ctrl Pts',(5.751742954317,0.6366272854614,3.200971110614));
#14148=CARTESIAN_POINT('Ctrl Pts',(5.857909620984,-0.4599252670358,3.136380672689));
#14149=CARTESIAN_POINT('Ctrl Pts',(5.910992954317,-0.9656781074217,2.972051613422));
#14150=CARTESIAN_POINT('Ctrl Pts',(0.7040070456828,-0.9656781074217,-2.972051613422));
#14151=CARTESIAN_POINT('Ctrl Pts',(0.7570903790161,-0.4599252670358,-3.136380672689));
#14152=CARTESIAN_POINT('Ctrl Pts',(0.8632570456828,0.6366272854614,-3.200971110614));
#14153=CARTESIAN_POINT('Ctrl Pts',(1.022507045683,2.119635939241,-2.481754111378));
#14154=CARTESIAN_POINT('Ctrl Pts',(1.181757045683,3.061979863765,-1.129624298873));
#14155=CARTESIAN_POINT('Ctrl Pts',(1.341007045683,3.223532154246,0.5105564866689));
#14156=CARTESIAN_POINT('Ctrl Pts',(1.500257045683,2.563047905408,2.020544571702));
#14157=CARTESIAN_POINT('Ctrl Pts',(1.659507045683,1.248968678135,3.015276776083));
#14158=CARTESIAN_POINT('Ctrl Pts',(1.818757045683,-0.383608261101,3.241089558554));
#14159=CARTESIAN_POINT('Ctrl Pts',(1.978007045683,-1.918361836065,2.640398557608));
#14160=CARTESIAN_POINT('Ctrl Pts',(2.137257045683,-2.963917875123,1.366384855545));
#14161=CARTESIAN_POINT('Ctrl Pts',(2.296507045683,-3.253651172662,-0.256067900963));
#14162=CARTESIAN_POINT('Ctrl Pts',(2.455757045683,-2.713677441724,-1.813221296591));
#14163=CARTESIAN_POINT('Ctrl Pts',(2.615007045683,-1.481694291113,-2.907988781792));
#14164=CARTESIAN_POINT('Ctrl Pts',(2.774257045683,0.1281327360592,-3.261195904774));
#14165=CARTESIAN_POINT('Ctrl Pts',(2.933507045683,1.705284892359,-2.782772028626));
#14166=CARTESIAN_POINT('Ctrl Pts',(3.092757045683,2.84757578293,-1.59471906236));
#14167=CARTESIAN_POINT('Ctrl Pts',(3.252007045683,3.263712108535,0.));
#14168=CARTESIAN_POINT('Ctrl Pts',(3.411257045683,2.84757578293,1.59471906236));
#14169=CARTESIAN_POINT('Ctrl Pts',(3.570507045683,1.705284892359,2.782772028626));
#14170=CARTESIAN_POINT('Ctrl Pts',(3.729757045683,0.1281327360592,3.261195904774));
#14171=CARTESIAN_POINT('Ctrl Pts',(3.889007045683,-1.481694291113,2.907988781792));
#14172=CARTESIAN_POINT('Ctrl Pts',(4.048257045683,-2.713677441724,1.813221296591));
#14173=CARTESIAN_POINT('Ctrl Pts',(4.207507045683,-3.253651172662,0.256067900963));
#14174=CARTESIAN_POINT('Ctrl Pts',(4.366757045683,-2.963917875123,-1.366384855545));
#14175=CARTESIAN_POINT('Ctrl Pts',(4.526007045683,-1.918361836065,-2.640398557608));
#14176=CARTESIAN_POINT('Ctrl Pts',(4.685257045683,-0.383608261101,-3.241089558554));
#14177=CARTESIAN_POINT('Ctrl Pts',(4.844507045683,1.248968678135,-3.015276776083));
#14178=CARTESIAN_POINT('Ctrl Pts',(5.003757045683,2.563047905408,-2.020544571702));
#14179=CARTESIAN_POINT('Ctrl Pts',(5.163007045683,3.223532154246,-0.510556486669));
#14180=CARTESIAN_POINT('Ctrl Pts',(5.322257045683,3.061979863765,1.129624298873));
#14181=CARTESIAN_POINT('Ctrl Pts',(5.481507045683,2.119635939241,2.481754111378));
#14182=CARTESIAN_POINT('Ctrl Pts',(5.640757045683,0.6366272854614,3.200971110614));
#14183=CARTESIAN_POINT('Ctrl Pts',(5.746923712349,-0.4599252670358,3.136380672689));
#14184=CARTESIAN_POINT('Ctrl Pts',(5.800007045683,-0.9656781074217,2.972051613422));
#14185=CARTESIAN_POINT('Ctrl Pts',(0.5930211370484,-0.9656781074217,-2.972051613422));
#14186=CARTESIAN_POINT('Ctrl Pts',(0.6461044703817,-0.4599252670358,-3.136380672689));
#14187=CARTESIAN_POINT('Ctrl Pts',(0.7522711370484,0.6366272854614,-3.200971110614));
#14188=CARTESIAN_POINT('Ctrl Pts',(0.9115211370484,2.119635939241,-2.481754111378));
#14189=CARTESIAN_POINT('Ctrl Pts',(1.070771137048,3.061979863765,-1.129624298873));
#14190=CARTESIAN_POINT('Ctrl Pts',(1.230021137048,3.223532154246,0.5105564866689));
#14191=CARTESIAN_POINT('Ctrl Pts',(1.389271137048,2.563047905408,2.020544571702));
#14192=CARTESIAN_POINT('Ctrl Pts',(1.548521137048,1.248968678135,3.015276776083));
#14193=CARTESIAN_POINT('Ctrl Pts',(1.707771137048,-0.383608261101,3.241089558554));
#14194=CARTESIAN_POINT('Ctrl Pts',(1.867021137048,-1.918361836065,2.640398557608));
#14195=CARTESIAN_POINT('Ctrl Pts',(2.026271137048,-2.963917875123,1.366384855545));
#14196=CARTESIAN_POINT('Ctrl Pts',(2.185521137048,-3.253651172662,-0.256067900963));
#14197=CARTESIAN_POINT('Ctrl Pts',(2.344771137048,-2.713677441724,-1.813221296591));
#14198=CARTESIAN_POINT('Ctrl Pts',(2.504021137048,-1.481694291113,-2.907988781792));
#14199=CARTESIAN_POINT('Ctrl Pts',(2.663271137048,0.1281327360592,-3.261195904774));
#14200=CARTESIAN_POINT('Ctrl Pts',(2.822521137048,1.705284892359,-2.782772028626));
#14201=CARTESIAN_POINT('Ctrl Pts',(2.981771137048,2.84757578293,-1.59471906236));
#14202=CARTESIAN_POINT('Ctrl Pts',(3.141021137048,3.263712108535,0.));
#14203=CARTESIAN_POINT('Ctrl Pts',(3.300271137048,2.84757578293,1.59471906236));
#14204=CARTESIAN_POINT('Ctrl Pts',(3.459521137048,1.705284892359,2.782772028626));
#14205=CARTESIAN_POINT('Ctrl Pts',(3.618771137048,0.1281327360592,3.261195904774));
#14206=CARTESIAN_POINT('Ctrl Pts',(3.778021137048,-1.481694291113,2.907988781792));
#14207=CARTESIAN_POINT('Ctrl Pts',(3.937271137048,-2.713677441724,1.813221296591));
#14208=CARTESIAN_POINT('Ctrl Pts',(4.096521137048,-3.253651172662,0.256067900963));
#14209=CARTESIAN_POINT('Ctrl Pts',(4.255771137048,-2.963917875123,-1.366384855545));
#14210=CARTESIAN_POINT('Ctrl Pts',(4.415021137048,-1.918361836065,-2.640398557608));
#14211=CARTESIAN_POINT('Ctrl Pts',(4.574271137048,-0.383608261101,-3.241089558554));
#14212=CARTESIAN_POINT('Ctrl Pts',(4.733521137048,1.248968678135,-3.015276776083));
#14213=CARTESIAN_POINT('Ctrl Pts',(4.892771137048,2.563047905408,-2.020544571702));
#14214=CARTESIAN_POINT('Ctrl Pts',(5.052021137048,3.223532154246,-0.510556486669));
#14215=CARTESIAN_POINT('Ctrl Pts',(5.211271137048,3.061979863765,1.129624298873));
#14216=CARTESIAN_POINT('Ctrl Pts',(5.370521137048,2.119635939241,2.481754111378));
#14217=CARTESIAN_POINT('Ctrl Pts',(5.529771137048,0.6366272854614,3.200971110614));
#14218=CARTESIAN_POINT('Ctrl Pts',(5.635937803715,-0.4599252670358,3.136380672689));
#14219=CARTESIAN_POINT('Ctrl Pts',(5.689021137048,-0.9656781074217,2.972051613422));
#14220=CARTESIAN_POINT('',(5.88,-1.32348898008484E-22,3.125));
#14221=CARTESIAN_POINT('',(5.88,0.,3.125));
#14222=CARTESIAN_POINT('Ctrl Pts',(0.98,3.2169591004938E-7,-3.12449703095644));
#14223=CARTESIAN_POINT('Ctrl Pts',(0.9957051282051,0.157306535044492,-3.12459764304402));
#14224=CARTESIAN_POINT('Ctrl Pts',(1.01141025641005,0.314639539052909,-3.112929841749));
#14225=CARTESIAN_POINT('Ctrl Pts',(1.02711538461519,0.470193579471061,-3.08937038670253));
#14226=CARTESIAN_POINT('Ctrl Pts',(1.03182698771781,0.516860431844727,-3.08230245321972));
#14227=CARTESIAN_POINT('Ctrl Pts',(1.03653859082045,0.563365438343652,-3.07416446995282));
#14228=CARTESIAN_POINT('Ctrl Pts',(1.04125019392309,0.609657256300367,-3.06495400126008));
#14229=CARTESIAN_POINT('Ctrl Pts',(1.05224371902567,0.717669381189642,-3.04346332885533));
#14230=CARTESIAN_POINT('Ctrl Pts',(1.0632372441283,0.824520523417935,-3.01613287001461));
#14231=CARTESIAN_POINT('Ctrl Pts',(1.07423076923084,0.929617596829347,-2.98324879794399));
#14232=CARTESIAN_POINT('Ctrl Pts',(1.089935897436,1.07975715593506,-2.93627127590627));
#14233=CARTESIAN_POINT('Ctrl Pts',(1.10564102564099,1.22632914373851,-2.87796151164342));
#14234=CARTESIAN_POINT('Ctrl Pts',(1.12134615384615,1.36775803719343,-2.8091039241222));
#14235=CARTESIAN_POINT('Ctrl Pts',(1.13705128205133,1.5091869306485,-2.74024633660091));
#14236=CARTESIAN_POINT('Ctrl Pts',(1.15275641025667,1.64548597437029,-2.66083432711573));
#14237=CARTESIAN_POINT('Ctrl Pts',(1.16846153846185,1.77506014945936,-2.57161807835128));
#14238=CARTESIAN_POINT('Ctrl Pts',(1.17914097076807,1.86317013579121,-2.51095134091064));
#14239=CARTESIAN_POINT('Ctrl Pts',(1.18982040307421,1.94817288076982,-2.44574669164713));
#14240=CARTESIAN_POINT('Ctrl Pts',(1.20049983538033,2.02952515103173,-2.37626864249983));
#14241=CARTESIAN_POINT('Ctrl Pts',(1.20552553127922,2.06780918704612,-2.34357256496935));
#14242=CARTESIAN_POINT('Ctrl Pts',(1.2105512271781,2.10528488988288,-2.30993026036317));
#14243=CARTESIAN_POINT('Ctrl Pts',(1.21557692307699,2.14191592065948,-2.27539299236903));
#14244=CARTESIAN_POINT('Ctrl Pts',(1.23128205128199,2.25638664196909,-2.16746520831449));
#14245=CARTESIAN_POINT('Ctrl Pts',(1.24698717948701,2.36259770943883,-2.05080969082419));
#14246=CARTESIAN_POINT('Ctrl Pts',(1.26269230769218,2.45953351178139,-1.92692186650592));
#14247=CARTESIAN_POINT('Ctrl Pts',(1.27839743589734,2.55646931412384,-1.80303404218777));
#14248=CARTESIAN_POINT('Ctrl Pts',(1.29410256410266,2.64414127751746,-1.6719042538725));
#14249=CARTESIAN_POINT('Ctrl Pts',(1.30980769230782,2.72154967470347,-1.53495847225765));
#14250=CARTESIAN_POINT('Ctrl Pts',(1.32551282051299,2.79895807188956,-1.39801269064265));
#14251=CARTESIAN_POINT('Ctrl Pts',(1.34121794871801,2.86610550760182,-1.25523572060086));
#14252=CARTESIAN_POINT('Ctrl Pts',(1.35692307692301,2.92192333127629,-1.10813935100359));
#14253=CARTESIAN_POINT('Ctrl Pts',(1.35786539277047,2.9252724296811,-1.09931349244548));
#14254=CARTESIAN_POINT('Ctrl Pts',(1.35880770861792,2.92858070337731,-1.09047219858789));
#14255=CARTESIAN_POINT('Ctrl Pts',(1.35975002446537,2.93184792475783,-1.08161580336685));
#14256=CARTESIAN_POINT('Ctrl Pts',(1.37451283682291,2.98303392179007,-0.942866889013087));
#14257=CARTESIAN_POINT('Ctrl Pts',(1.38927564918046,3.02414182613375,-0.800411122418192));
#14258=CARTESIAN_POINT('Ctrl Pts',(1.40403846153816,3.05502438429729,-0.655798952752522));
#14259=CARTESIAN_POINT('Ctrl Pts',(1.41974358974334,3.08787818772652,-0.50195613408092));
#14260=CARTESIAN_POINT('Ctrl Pts',(1.4354487179487,3.10916841598543,-0.345660030799849));
#14261=CARTESIAN_POINT('Ctrl Pts',(1.45115384615389,3.1187342224115,-0.188648419769014));
#14262=CARTESIAN_POINT('Ctrl Pts',(1.46685897435902,3.12830002883752,-0.0316368087388328));
#14263=CARTESIAN_POINT('Ctrl Pts',(1.48256410256397,3.12614026969898,0.12610510103707));
#14264=CARTESIAN_POINT('Ctrl Pts',(1.49826923076908,3.11205714799653,0.282798238157188));
#14265=CARTESIAN_POINT('Ctrl Pts',(1.50517951072145,3.10586055333675,0.351743453374321));
#14266=CARTESIAN_POINT('Ctrl Pts',(1.51208979067384,3.09735519217736,0.420484489677447));
#14267=CARTESIAN_POINT('Ctrl Pts',(1.51900007062624,3.0865260643595,0.488857703250767));
#14268=CARTESIAN_POINT('Ctrl Pts',(1.52779491887912,3.07274362189333,0.575877627491321));
#14269=CARTESIAN_POINT('Ctrl Pts',(1.536589767132,3.05519690668903,0.66230164565767));
#14270=CARTESIAN_POINT('Ctrl Pts',(1.54538461538482,3.0340200977109,0.74781859016398));
#14271=CARTESIAN_POINT('Ctrl Pts',(1.56108974359,2.99620426616755,0.900527828411023));
#14272=CARTESIAN_POINT('Ctrl Pts',(1.576794871795,2.94681582966476,1.05034855944726));
#14273=CARTESIAN_POINT('Ctrl Pts',(1.5925,2.88658577275698,1.1956628320182));
#14274=CARTESIAN_POINT('Ctrl Pts',(1.608205128205,2.82635571584919,1.34097710458913));
#14275=CARTESIAN_POINT('Ctrl Pts',(1.62391025641,2.75527937991822,1.48179891776845));
#14276=CARTESIAN_POINT('Ctrl Pts',(1.63961538461517,2.67404531641151,1.61651716219695));
#14277=CARTESIAN_POINT('Ctrl Pts',(1.65249354986765,2.60743359059155,1.72698578057497));
#14278=CARTESIAN_POINT('Ctrl Pts',(1.66537171512024,2.53398384454478,1.83335602635669));
#14279=CARTESIAN_POINT('Ctrl Pts',(1.67824988037278,2.45411540900217,1.93466859159332));
#14280=CARTESIAN_POINT('Ctrl Pts',(1.68107684332548,2.43658301180572,1.9569083177461));
#14281=CARTESIAN_POINT('Ctrl Pts',(1.68390380627817,2.41874138908149,1.97890437133876));
#14282=CARTESIAN_POINT('Ctrl Pts',(1.68673076923086,2.4005992967642,2.00064999697506));
#14283=CARTESIAN_POINT('Ctrl Pts',(1.70243589743605,2.29981131668746,2.12145732421479));
#14284=CARTESIAN_POINT('Ctrl Pts',(1.71814102564111,2.18976698077217,2.23451450223418));
#14285=CARTESIAN_POINT('Ctrl Pts',(1.73384615384633,2.07193616153301,2.33873186210924));
#14286=CARTESIAN_POINT('Ctrl Pts',(1.74955128205139,1.95410534229508,2.44294922198321));
#14287=CARTESIAN_POINT('Ctrl Pts',(1.76525641025661,1.82847988986133,2.53833958057375));
#14288=CARTESIAN_POINT('Ctrl Pts',(1.78096153846167,1.69644712969505,2.62385329049029));
#14289=CARTESIAN_POINT('Ctrl Pts',(1.79666666666689,1.56441436952739,2.70936700040773));
#14290=CARTESIAN_POINT('Ctrl Pts',(1.81237179487195,1.42595984987577,2.78500861783667));
#14291=CARTESIAN_POINT('Ctrl Pts',(1.82807692307697,1.28252819003516,2.84966078036119));
#14292=CARTESIAN_POINT('Ctrl Pts',(1.83121799320022,1.25384145182002,2.86259139598291));
#14293=CARTESIAN_POINT('Ctrl Pts',(1.83435906332346,1.22495656311743,2.8750820037678));
#14294=CARTESIAN_POINT('Ctrl Pts',(1.83750013344671,1.19588572614117,2.887123539098));
#14295=CARTESIAN_POINT('Ctrl Pts',(1.85006419152849,1.07960443666829,2.93528882778825));
#14296=CARTESIAN_POINT('Ctrl Pts',(1.86262824961027,0.960347655502351,2.97626761538678));
#14297=CARTESIAN_POINT('Ctrl Pts',(1.87519230769217,0.83908019289306,3.00992620370386));
#14298=CARTESIAN_POINT('Ctrl Pts',(1.89089743589733,0.687495327956873,3.05199958805779));
#14299=CARTESIAN_POINT('Ctrl Pts',(1.90660256410267,0.532757793114142,3.08264413157538));
#14300=CARTESIAN_POINT('Ctrl Pts',(1.92230769230783,0.376606556598297,3.10163498008567));
#14301=CARTESIAN_POINT('Ctrl Pts',(1.938012820513,0.220455320082452,3.12062582859596));
#14302=CARTESIAN_POINT('Ctrl Pts',(1.953717948718,0.0628756645481053,3.12796387302098));
#14303=CARTESIAN_POINT('Ctrl Pts',(1.96942307692303,-0.0943789619765685,
3.12338542308761));
#14304=CARTESIAN_POINT('Ctrl Pts',(1.97853202085236,-0.185586340671023,
3.12072993099726));
#14305=CARTESIAN_POINT('Ctrl Pts',(1.9876409647817,-0.276685802602259,3.11406434039434));
#14306=CARTESIAN_POINT('Ctrl Pts',(1.99674990871107,-0.367304367055667,
3.1033389279845));
#14307=CARTESIAN_POINT('Ctrl Pts',(2.0033460929868,-0.432925228768213,3.09557218825737));
#14308=CARTESIAN_POINT('Ctrl Pts',(2.00994227726255,-0.49829389512535,3.0856767051092));
#14309=CARTESIAN_POINT('Ctrl Pts',(2.01653846153833,-0.563276981103758,
3.07370359533635));
#14310=CARTESIAN_POINT('Ctrl Pts',(2.03224358974339,-0.717997900620613,
3.04519632262624));
#14311=CARTESIAN_POINT('Ctrl Pts',(2.04794871794861,-0.870526272338106,
3.00491480017494));
#14312=CARTESIAN_POINT('Ctrl Pts',(2.06365384615367,-1.01920094228015,2.95353305961267));
#14313=CARTESIAN_POINT('Ctrl Pts',(2.07935897435889,-1.16787561222373,2.90215131904986));
#14314=CARTESIAN_POINT('Ctrl Pts',(2.09506410256395,-1.31271118268685,2.83966664030563));
#14315=CARTESIAN_POINT('Ctrl Pts',(2.11076923076914,-1.45207966320917,2.76670577109897));
#14316=CARTESIAN_POINT('Ctrl Pts',(2.12584614949763,-1.58587336592168,2.69666335686228));
#14317=CARTESIAN_POINT('Ctrl Pts',(2.14092306822624,-1.71463784791186,2.61695511461419));
#14318=CARTESIAN_POINT('Ctrl Pts',(2.15599998695471,-1.836828913414,2.52817810742183));
#14319=CARTESIAN_POINT('Ctrl Pts',(2.15662819643142,-1.84192024452083,2.52447903878345));
#14320=CARTESIAN_POINT('Ctrl Pts',(2.15725640590813,-1.8470001649315,2.52076422913783));
#14321=CARTESIAN_POINT('Ctrl Pts',(2.15788461538483,-1.85206859791098,2.51703377008661));
#14322=CARTESIAN_POINT('Ctrl Pts',(2.17358974359,-1.97877854529902,2.42377293936711));
#14323=CARTESIAN_POINT('Ctrl Pts',(2.189294871795,-2.09828043057227,2.32075011669408));
#14324=CARTESIAN_POINT('Ctrl Pts',(2.205,-2.20940661429584,2.20940720229315));
#14325=CARTESIAN_POINT('Ctrl Pts',(2.220705128205,-2.32053279801942,2.09806428789222));
#14326=CARTESIAN_POINT('Ctrl Pts',(2.23641025641,-2.42329735285879,1.97839483543744));
#14327=CARTESIAN_POINT('Ctrl Pts',(2.25211538461517,-2.51660034679189,1.85174928324409));
#14328=CARTESIAN_POINT('Ctrl Pts',(2.26782051282033,-2.60990334072498,1.72510373105075));
#14329=CARTESIAN_POINT('Ctrl Pts',(2.28352564102567,-2.69375117108915,1.59146857523107));
#14330=CARTESIAN_POINT('Ctrl Pts',(2.29923076923086,-2.76698261297629,1.45222443021403));
#14331=CARTESIAN_POINT('Ctrl Pts',(2.30457056320872,-2.79188153817257,1.40488097415942));
#14332=CARTESIAN_POINT('Ctrl Pts',(2.30991035718657,-2.81555228674541,1.35689047491984));
#14333=CARTESIAN_POINT('Ctrl Pts',(2.31525015116441,-2.83794741820317,1.30831167980417));
#14334=CARTESIAN_POINT('Ctrl Pts',(2.3256154853917,-2.88141969889172,1.21401301400872));
#14335=CARTESIAN_POINT('Ctrl Pts',(2.33598081961898,-2.9200846630212,1.11749740512214));
#14336=CARTESIAN_POINT('Ctrl Pts',(2.34634615384633,-2.95384328122045,1.01930854475146));
#14337=CARTESIAN_POINT('Ctrl Pts',(2.36205128205139,-3.00499295138217,0.87053682098386));
#14338=CARTESIAN_POINT('Ctrl Pts',(2.37775641025661,-3.04488646955173,0.717917299307509));
#14339=CARTESIAN_POINT('Ctrl Pts',(2.39346153846167,-3.07323267657501,0.563190821606756));
#14340=CARTESIAN_POINT('Ctrl Pts',(2.40916666666689,-3.10157888359858,0.408464343904395));
#14341=CARTESIAN_POINT('Ctrl Pts',(2.42487179487195,-3.11838067165169,0.25161647302184));
#14342=CARTESIAN_POINT('Ctrl Pts',(2.44057692307697,-3.12331108802163,0.094376207787104));
#14343=CARTESIAN_POINT('Ctrl Pts',(2.45188456103662,-3.12686097074617,-0.0188362390481932));
#14344=CARTESIAN_POINT('Ctrl Pts',(2.46319219899625,-3.12425420322951,-0.132257831845052));
#14345=CARTESIAN_POINT('Ctrl Pts',(2.47449983695594,-3.11536666791583,-0.245184674149663));
#14346=CARTESIAN_POINT('Ctrl Pts',(2.47889732720134,-3.11191034485466,-0.289101422213973));
#14347=CARTESIAN_POINT('Ctrl Pts',(2.48329481744675,-3.10750429091715,-0.332943335439869));
#14348=CARTESIAN_POINT('Ctrl Pts',(2.48769230769217,-3.10216193300488,-0.37667061407462));
#14349=CARTESIAN_POINT('Ctrl Pts',(2.50339743589733,-3.08308231912341,-0.532837536272352));
#14350=CARTESIAN_POINT('Ctrl Pts',(2.51910256410267,-3.05206338319806,-0.687523279012142));
#14351=CARTESIAN_POINT('Ctrl Pts',(2.53480769230783,-3.0097189125242,-0.839021679403842));
#14352=CARTESIAN_POINT('Ctrl Pts',(2.550512820513,-2.96737444185033,-0.990520079795541));
#14353=CARTESIAN_POINT('Ctrl Pts',(2.566217948718,-2.91370372918221,-1.13884614555346));
#14354=CARTESIAN_POINT('Ctrl Pts',(2.58192307692303,-2.84927329204631,-1.28235426733883));
#14355=CARTESIAN_POINT('Ctrl Pts',(2.59762820512805,-2.78484285491041,-1.42586238912421));
#14356=CARTESIAN_POINT('Ctrl Pts',(2.61333333333311,-2.70964227733817,-1.56456383704047));
#14357=CARTESIAN_POINT('Ctrl Pts',(2.62903846153833,-2.62426134529928,-1.69671142476984));
#14358=CARTESIAN_POINT('Ctrl Pts',(2.6306089923509,-2.61572315428164,-1.70992633493315));
#14359=CARTESIAN_POINT('Ctrl Pts',(2.63217952316347,-2.60708334093589,-1.72307544280506));
#14360=CARTESIAN_POINT('Ctrl Pts',(2.63375005397604,-2.59834253844517,-1.7361569781865));
#14361=CARTESIAN_POINT('Ctrl Pts',(2.64788465136855,-2.5196763173783,-1.85388929799372));
#14362=CARTESIAN_POINT('Ctrl Pts',(2.66201924876118,-2.4328286128156,-1.96614691665661));
#14363=CARTESIAN_POINT('Ctrl Pts',(2.67615384615367,-2.33882800562177,-2.07202028766332));
#14364=CARTESIAN_POINT('Ctrl Pts',(2.69185897435889,-2.23438275356725,-2.18965751630222));
#14365=CARTESIAN_POINT('Ctrl Pts',(2.70756410256395,-2.12110179310409,-2.29942752308062));
#14366=CARTESIAN_POINT('Ctrl Pts',(2.72326923076914,-2.00029920318409,-2.40017868230316));
#14367=CARTESIAN_POINT('Ctrl Pts',(2.73897435897433,-1.87949661326408,-2.5009298415257));
#14368=CARTESIAN_POINT('Ctrl Pts',(2.75467948717967,-1.75116000914845,-2.59267025933498));
#14369=CARTESIAN_POINT('Ctrl Pts',(2.77038461538483,-1.61660883785066,-2.674197927153));
#14370=CARTESIAN_POINT('Ctrl Pts',(2.77792308497015,-1.55202420668778,-2.71333124947796));
#14371=CARTESIAN_POINT('Ctrl Pts',(2.78546155455542,-1.48600787178097,-2.75011066378684));
#14372=CARTESIAN_POINT('Ctrl Pts',(2.79300002414067,-1.41872031168613,-2.78439538808883));
#14373=CARTESIAN_POINT('Ctrl Pts',(2.80116668276046,-1.34582560455246,-2.82153709650612));
#14374=CARTESIAN_POINT('Ctrl Pts',(2.80933334138023,-1.27143900290213,-2.85575093945237));
#14375=CARTESIAN_POINT('Ctrl Pts',(2.8175,-1.19582529175154,-2.88697719853058));
#14376=CARTESIAN_POINT('Ctrl Pts',(2.833205128205,-1.05041416549221,-2.94702775592731));
#14377=CARTESIAN_POINT('Ctrl Pts',(2.84891025641,-0.900465813463126,-2.99603287482205));
#14378=CARTESIAN_POINT('Ctrl Pts',(2.86461538461517,-0.747723396432291,
-3.03363235324925));
#14379=CARTESIAN_POINT('Ctrl Pts',(2.88032051282033,-0.594980979401457,
-3.07123183167645));
#14380=CARTESIAN_POINT('Ctrl Pts',(2.89602564102567,-0.439430544027183,
-3.09743052627249));
#14381=CARTESIAN_POINT('Ctrl Pts',(2.91173076923086,-0.282778041871423,
-3.11184033086417));
#14382=CARTESIAN_POINT('Ctrl Pts',(2.92523715029811,-0.148057181168531,
-3.12423273603125));
#14383=CARTESIAN_POINT('Ctrl Pts',(2.93874353136525,-0.0125106239082456,
-3.12790266438722));
#14384=CARTESIAN_POINT('Ctrl Pts',(2.95224991243248,0.122686924247132,-3.12259073825233));
#14385=CARTESIAN_POINT('Ctrl Pts',(2.95444865957043,0.144696167180856,-3.1217259927422));
#14386=CARTESIAN_POINT('Ctrl Pts',(2.95664740670838,0.166696155154839,-3.12062326574181));
#14387=CARTESIAN_POINT('Ctrl Pts',(2.95884615384633,0.1886819155548,-3.11928401449904));
#14388=CARTESIAN_POINT('Ctrl Pts',(2.97455128205139,0.345720976484957,-3.10971806118707));
#14389=CARTESIAN_POINT('Ctrl Pts',(2.99025641025661,0.502004351790296,-3.08808590041721));
#14390=CARTESIAN_POINT('Ctrl Pts',(3.00596153846167,0.655779338422631,-3.05493687313145));
#14391=CARTESIAN_POINT('Ctrl Pts',(3.02166666666689,0.809554325056565,-3.02178784584535));
#14392=CARTESIAN_POINT('Ctrl Pts',(3.03737179487195,0.960836126315138,-2.9771233215876));
#14393=CARTESIAN_POINT('Ctrl Pts',(3.05307692307697,1.10796040920211,-2.9214504428197));
#14394=CARTESIAN_POINT('Ctrl Pts',(3.068782051282,1.25508469208908,-2.86577756405179));
#14395=CARTESIAN_POINT('Ctrl Pts',(3.084487179487,1.39806382918831,-2.79908769904581));
#14396=CARTESIAN_POINT('Ctrl Pts',(3.10019230769217,1.53515081641421,-2.72188982514671));
#14397=CARTESIAN_POINT('Ctrl Pts',(3.10396158983553,1.56805214178305,-2.70336208288368));
#14398=CARTESIAN_POINT('Ctrl Pts',(3.1077308719789,1.60061292833792,-2.68422968792613));
#14399=CARTESIAN_POINT('Ctrl Pts',(3.11150015412227,1.63280801473754,-2.66450051360633));
#14400=CARTESIAN_POINT('Ctrl Pts',(3.12343600018412,1.73475729329959,-2.60202591535358));
#14401=CARTESIAN_POINT('Ctrl Pts',(3.13537184624603,1.8330386668105,-2.53356607404464));
#14402=CARTESIAN_POINT('Ctrl Pts',(3.14730769230783,1.92707055798493,-2.45972435726965));
#14403=CARTESIAN_POINT('Ctrl Pts',(3.163012820513,2.05079726312352,-2.36256378542284));
#14404=CARTESIAN_POINT('Ctrl Pts',(3.178717948718,2.16717972241397,-2.25608242363812));
#14405=CARTESIAN_POINT('Ctrl Pts',(3.19442307692303,2.27501273852753,-2.14155794469054));
#14406=CARTESIAN_POINT('Ctrl Pts',(3.21012820512806,2.3828457546411,-2.02703346574295));
#14407=CARTESIAN_POINT('Ctrl Pts',(3.22583333333311,2.48213900530219,-1.90445476333191));
#14408=CARTESIAN_POINT('Ctrl Pts',(3.24153846153833,2.57165193077396,-1.77508287620843));
#14409=CARTESIAN_POINT('Ctrl Pts',(3.25127559877096,2.62714970373215,-1.69487265426663));
#14410=CARTESIAN_POINT('Ctrl Pts',(3.26101273600365,2.67888797642152,-1.61204808608716));
#14411=CARTESIAN_POINT('Ctrl Pts',(3.27074987323633,2.72655002210233,-1.52694137967767));
#14412=CARTESIAN_POINT('Ctrl Pts',(3.27671786420879,2.75576257724611,-1.47477860910038));
#14413=CARTESIAN_POINT('Ctrl Pts',(3.28268585518124,2.78344401079767,-1.42175865550711));
#14414=CARTESIAN_POINT('Ctrl Pts',(3.28865384615367,2.80956688241491,-1.36798352909411));
#14415=CARTESIAN_POINT('Ctrl Pts',(3.30435897435889,2.87831079468499,-1.22647104047447));
#14416=CARTESIAN_POINT('Ctrl Pts',(3.32006410256394,2.9362584893282,-1.07973927060473));
#14417=CARTESIAN_POINT('Ctrl Pts',(3.33576923076914,2.982977349702,-0.929533639746724));
#14418=CARTESIAN_POINT('Ctrl Pts',(3.35147435897433,3.0296962100758,-0.779328008888721));
#14419=CARTESIAN_POINT('Ctrl Pts',(3.36717948717967,3.06519301000169,-0.625635251226046));
#14420=CARTESIAN_POINT('Ctrl Pts',(3.38288461538483,3.08901983228559,-0.470139769698067));
#14421=CARTESIAN_POINT('Ctrl Pts',(3.39858974359,3.11284665456948,-0.314644288170088));
#14422=CARTESIAN_POINT('Ctrl Pts',(3.414294871795,3.125,-0.157330906751383));
#14423=CARTESIAN_POINT('Ctrl Pts',(3.43,3.125,0.));
#14424=CARTESIAN_POINT('Ctrl Pts',(3.445705128205,3.125,0.157330906751383));
#14425=CARTESIAN_POINT('Ctrl Pts',(3.46141025641,3.11284665456948,0.314644288170091));
#14426=CARTESIAN_POINT('Ctrl Pts',(3.47711538461517,3.08901983228559,0.47013976969807));
#14427=CARTESIAN_POINT('Ctrl Pts',(3.49282051282033,3.06519301000169,0.625635251226049));
#14428=CARTESIAN_POINT('Ctrl Pts',(3.50852564102567,3.0296962100758,0.779328008888722));
#14429=CARTESIAN_POINT('Ctrl Pts',(3.52423076923086,2.982977349702,0.929533639746725));
#14430=CARTESIAN_POINT('Ctrl Pts',(3.53993589743606,2.9362584893282,1.07973927060473));
#14431=CARTESIAN_POINT('Ctrl Pts',(3.55564102564111,2.87831079468499,1.22647104047447));
#14432=CARTESIAN_POINT('Ctrl Pts',(3.57134615384633,2.80956688241491,1.36798352909411));
#14433=CARTESIAN_POINT('Ctrl Pts',(3.57731414481876,2.78344401079767,1.42175865550711));
#14434=CARTESIAN_POINT('Ctrl Pts',(3.58328213579121,2.75576257724611,1.47477860910038));
#14435=CARTESIAN_POINT('Ctrl Pts',(3.58925012676367,2.72655002210233,1.52694137967767));
#14436=CARTESIAN_POINT('Ctrl Pts',(3.59898726399635,2.67888797642152,1.61204808608716));
#14437=CARTESIAN_POINT('Ctrl Pts',(3.60872440122904,2.62714970373215,1.69487265426663));
#14438=CARTESIAN_POINT('Ctrl Pts',(3.61846153846167,2.57165193077395,1.77508287620844));
#14439=CARTESIAN_POINT('Ctrl Pts',(3.63416666666689,2.48213900530219,1.90445476333191));
#14440=CARTESIAN_POINT('Ctrl Pts',(3.64987179487195,2.3828457546411,2.02703346574295));
#14441=CARTESIAN_POINT('Ctrl Pts',(3.66557692307697,2.27501273852753,2.14155794469054));
#14442=CARTESIAN_POINT('Ctrl Pts',(3.681282051282,2.16717972241396,2.25608242363812));
#14443=CARTESIAN_POINT('Ctrl Pts',(3.696987179487,2.05079726312352,2.36256378542284));
#14444=CARTESIAN_POINT('Ctrl Pts',(3.71269230769217,1.92707055798493,2.45972435726965));
#14445=CARTESIAN_POINT('Ctrl Pts',(3.72462815375397,1.8330386668105,2.53356607404464));
#14446=CARTESIAN_POINT('Ctrl Pts',(3.73656399981588,1.73475729329959,2.60202591535358));
#14447=CARTESIAN_POINT('Ctrl Pts',(3.74849984587773,1.63280801473754,2.66450051360633));
#14448=CARTESIAN_POINT('Ctrl Pts',(3.7522691280211,1.60061292833792,2.68422968792613));
#14449=CARTESIAN_POINT('Ctrl Pts',(3.75603841016447,1.56805214178305,2.70336208288368));
#14450=CARTESIAN_POINT('Ctrl Pts',(3.75980769230783,1.53515081641421,2.72188982514671));
#14451=CARTESIAN_POINT('Ctrl Pts',(3.775512820513,1.39806382918831,2.79908769904581));
#14452=CARTESIAN_POINT('Ctrl Pts',(3.791217948718,1.25508469208908,2.86577756405179));
#14453=CARTESIAN_POINT('Ctrl Pts',(3.80692307692303,1.10796040920211,2.92145044281969));
#14454=CARTESIAN_POINT('Ctrl Pts',(3.82262820512805,0.960836126315141,2.9771233215876));
#14455=CARTESIAN_POINT('Ctrl Pts',(3.83833333333311,0.809554325056562,3.02178784584535));
#14456=CARTESIAN_POINT('Ctrl Pts',(3.85403846153833,0.655779338422628,3.05493687313145));
#14457=CARTESIAN_POINT('Ctrl Pts',(3.86974358974339,0.502004351790293,3.08808590041721));
#14458=CARTESIAN_POINT('Ctrl Pts',(3.88544871794861,0.345720976484962,3.10971806118707));
#14459=CARTESIAN_POINT('Ctrl Pts',(3.90115384615367,0.188681915554805,3.11928401449904));
#14460=CARTESIAN_POINT('Ctrl Pts',(3.90335259329162,0.166696155154845,3.12062326574181));
#14461=CARTESIAN_POINT('Ctrl Pts',(3.90555134042957,0.144696167180862,3.1217259927422));
#14462=CARTESIAN_POINT('Ctrl Pts',(3.90775008756752,0.122686924247137,3.12259073825233));
#14463=CARTESIAN_POINT('Ctrl Pts',(3.92125646863475,-0.0125106239082456,
3.12790266438722));
#14464=CARTESIAN_POINT('Ctrl Pts',(3.9347628497019,-0.148057181168534,3.12423273603126));
#14465=CARTESIAN_POINT('Ctrl Pts',(3.94826923076914,-0.282778041871425,
3.11184033086417));
#14466=CARTESIAN_POINT('Ctrl Pts',(3.96397435897433,-0.439430544027182,
3.09743052627249));
#14467=CARTESIAN_POINT('Ctrl Pts',(3.97967948717967,-0.594980979401456,
3.07123183167645));
#14468=CARTESIAN_POINT('Ctrl Pts',(3.99538461538483,-0.747723396432294,
3.03363235324925));
#14469=CARTESIAN_POINT('Ctrl Pts',(4.01108974359,-0.900465813463131,2.99603287482204));
#14470=CARTESIAN_POINT('Ctrl Pts',(4.026794871795,-1.05041416549222,2.94702775592731));
#14471=CARTESIAN_POINT('Ctrl Pts',(4.0425,-1.19582529175154,2.88697719853058));
#14472=CARTESIAN_POINT('Ctrl Pts',(4.05066665861977,-1.27143900290213,2.85575093945237));
#14473=CARTESIAN_POINT('Ctrl Pts',(4.05883331723954,-1.34582560455246,2.82153709650612));
#14474=CARTESIAN_POINT('Ctrl Pts',(4.06699997585933,-1.41872031168613,2.78439538808883));
#14475=CARTESIAN_POINT('Ctrl Pts',(4.07453844544458,-1.48600787178097,2.75011066378684));
#14476=CARTESIAN_POINT('Ctrl Pts',(4.08207691502986,-1.55202420668778,2.71333124947796));
#14477=CARTESIAN_POINT('Ctrl Pts',(4.08961538461517,-1.61660883785066,2.674197927153));
#14478=CARTESIAN_POINT('Ctrl Pts',(4.10532051282033,-1.75116000914844,2.59267025933498));
#14479=CARTESIAN_POINT('Ctrl Pts',(4.12102564102567,-1.87949661326408,2.5009298415257));
#14480=CARTESIAN_POINT('Ctrl Pts',(4.13673076923086,-2.00029920318409,2.40017868230316));
#14481=CARTESIAN_POINT('Ctrl Pts',(4.15243589743605,-2.12110179310409,2.29942752308062));
#14482=CARTESIAN_POINT('Ctrl Pts',(4.16814102564111,-2.23438275356726,2.18965751630222));
#14483=CARTESIAN_POINT('Ctrl Pts',(4.18384615384633,-2.33882800562177,2.07202028766331));
#14484=CARTESIAN_POINT('Ctrl Pts',(4.19798075123882,-2.4328286128156,1.9661469166566));
#14485=CARTESIAN_POINT('Ctrl Pts',(4.21211534863145,-2.5196763173783,1.85388929799372));
#14486=CARTESIAN_POINT('Ctrl Pts',(4.22624994602396,-2.59834253844517,1.7361569781865));
#14487=CARTESIAN_POINT('Ctrl Pts',(4.22782047683653,-2.60708334093589,1.72307544280507));
#14488=CARTESIAN_POINT('Ctrl Pts',(4.2293910076491,-2.61572315428164,1.70992633493316));
#14489=CARTESIAN_POINT('Ctrl Pts',(4.23096153846167,-2.62426134529928,1.69671142476984));
#14490=CARTESIAN_POINT('Ctrl Pts',(4.24666666666689,-2.70964227733817,1.56456383704048));
#14491=CARTESIAN_POINT('Ctrl Pts',(4.26237179487195,-2.78484285491041,1.42586238912421));
#14492=CARTESIAN_POINT('Ctrl Pts',(4.27807692307697,-2.84927329204631,1.28235426733883));
#14493=CARTESIAN_POINT('Ctrl Pts',(4.293782051282,-2.91370372918221,1.13884614555346));
#14494=CARTESIAN_POINT('Ctrl Pts',(4.309487179487,-2.96737444185033,0.990520079795544));
#14495=CARTESIAN_POINT('Ctrl Pts',(4.32519230769217,-3.0097189125242,0.839021679403841));
#14496=CARTESIAN_POINT('Ctrl Pts',(4.34089743589733,-3.05206338319806,0.687523279012144));
#14497=CARTESIAN_POINT('Ctrl Pts',(4.35660256410267,-3.08308231912341,0.532837536272352));
#14498=CARTESIAN_POINT('Ctrl Pts',(4.37230769230783,-3.10216193300488,0.376670614074617));
#14499=CARTESIAN_POINT('Ctrl Pts',(4.37670518255325,-3.10750429091715,0.332943335439869));
#14500=CARTESIAN_POINT('Ctrl Pts',(4.38110267279866,-3.11191034485466,0.289101422213986));
#14501=CARTESIAN_POINT('Ctrl Pts',(4.38550016304406,-3.11536666791583,0.245184674149674));
#14502=CARTESIAN_POINT('Ctrl Pts',(4.39680780100375,-3.12425420322951,0.132257831845052));
#14503=CARTESIAN_POINT('Ctrl Pts',(4.40811543896338,-3.12686097074617,0.0188362390481956));
#14504=CARTESIAN_POINT('Ctrl Pts',(4.41942307692303,-3.12331108802163,-0.0943762077871013));
#14505=CARTESIAN_POINT('Ctrl Pts',(4.43512820512805,-3.11838067165169,-0.251616473021838));
#14506=CARTESIAN_POINT('Ctrl Pts',(4.45083333333311,-3.10157888359858,-0.408464343904398));
#14507=CARTESIAN_POINT('Ctrl Pts',(4.46653846153833,-3.07323267657501,-0.563190821606759));
#14508=CARTESIAN_POINT('Ctrl Pts',(4.48224358974339,-3.04488646955173,-0.717917299307511));
#14509=CARTESIAN_POINT('Ctrl Pts',(4.49794871794861,-3.00499295138217,-0.87053682098386));
#14510=CARTESIAN_POINT('Ctrl Pts',(4.51365384615367,-2.95384328122045,-1.01930854475146));
#14511=CARTESIAN_POINT('Ctrl Pts',(4.52401918038102,-2.9200846630212,-1.11749740512214));
#14512=CARTESIAN_POINT('Ctrl Pts',(4.5343845146083,-2.88141969889172,-1.21401301400872));
#14513=CARTESIAN_POINT('Ctrl Pts',(4.54474984883559,-2.83794741820317,-1.30831167980417));
#14514=CARTESIAN_POINT('Ctrl Pts',(4.55008964281343,-2.8155522867454,-1.35689047491985));
#14515=CARTESIAN_POINT('Ctrl Pts',(4.55542943679128,-2.79188153817257,-1.40488097415943));
#14516=CARTESIAN_POINT('Ctrl Pts',(4.56076923076914,-2.76698261297628,-1.45222443021404));
#14517=CARTESIAN_POINT('Ctrl Pts',(4.57647435897433,-2.69375117108915,-1.59146857523107));
#14518=CARTESIAN_POINT('Ctrl Pts',(4.59217948717967,-2.60990334072498,-1.72510373105075));
#14519=CARTESIAN_POINT('Ctrl Pts',(4.60788461538483,-2.51660034679189,-1.8517492832441));
#14520=CARTESIAN_POINT('Ctrl Pts',(4.62358974359,-2.42329735285879,-1.97839483543744));
#14521=CARTESIAN_POINT('Ctrl Pts',(4.639294871795,-2.32053279801942,-2.09806428789222));
#14522=CARTESIAN_POINT('Ctrl Pts',(4.655,-2.20940661429584,-2.20940720229315));
#14523=CARTESIAN_POINT('Ctrl Pts',(4.670705128205,-2.09828043057227,-2.32075011669408));
#14524=CARTESIAN_POINT('Ctrl Pts',(4.68641025641,-1.97877854529902,-2.42377293936711));
#14525=CARTESIAN_POINT('Ctrl Pts',(4.70211538461517,-1.85206859791098,-2.51703377008662));
#14526=CARTESIAN_POINT('Ctrl Pts',(4.70274359409187,-1.84700016493149,-2.52076422913783));
#14527=CARTESIAN_POINT('Ctrl Pts',(4.70337180356858,-1.84192024452082,-2.52447903878346));
#14528=CARTESIAN_POINT('Ctrl Pts',(4.70400001304529,-1.83682891341399,-2.52817810742184));
#14529=CARTESIAN_POINT('Ctrl Pts',(4.71907693177376,-1.71463784791186,-2.61695511461419));
#14530=CARTESIAN_POINT('Ctrl Pts',(4.73415385050237,-1.58587336592168,-2.69666335686228));
#14531=CARTESIAN_POINT('Ctrl Pts',(4.74923076923086,-1.45207966320917,-2.76670577109897));
#14532=CARTESIAN_POINT('Ctrl Pts',(4.76493589743605,-1.31271118268685,-2.83966664030563));
#14533=CARTESIAN_POINT('Ctrl Pts',(4.78064102564111,-1.16787561222373,-2.90215131904986));
#14534=CARTESIAN_POINT('Ctrl Pts',(4.79634615384633,-1.01920094228016,-2.95353305961267));
#14535=CARTESIAN_POINT('Ctrl Pts',(4.81205128205139,-0.870526272338138,
-3.00491480017493));
#14536=CARTESIAN_POINT('Ctrl Pts',(4.82775641025661,-0.717997900620678,
-3.04519632262622));
#14537=CARTESIAN_POINT('Ctrl Pts',(4.84346153846167,-0.563276981103821,
-3.07370359533634));
#14538=CARTESIAN_POINT('Ctrl Pts',(4.85005772273745,-0.498293895125397,
-3.08567670510919));
#14539=CARTESIAN_POINT('Ctrl Pts',(4.8566539070132,-0.432925228768243,-3.09557218825737));
#14540=CARTESIAN_POINT('Ctrl Pts',(4.86325009128893,-0.367304367055667,
-3.1033389279845));
#14541=CARTESIAN_POINT('Ctrl Pts',(4.87235903521831,-0.276685802602259,
-3.11406434039434));
#14542=CARTESIAN_POINT('Ctrl Pts',(4.88146797914764,-0.185586340671027,
-3.12072993099726));
#14543=CARTESIAN_POINT('Ctrl Pts',(4.89057692307697,-0.0943789619765783,
-3.12338542308761));
#14544=CARTESIAN_POINT('Ctrl Pts',(4.906282051282,0.0628756645481118,-3.12796387302098));
#14545=CARTESIAN_POINT('Ctrl Pts',(4.921987179487,0.220455320082457,-3.12062582859596));
#14546=CARTESIAN_POINT('Ctrl Pts',(4.93769230769217,0.376606556598298,-3.10163498008567));
#14547=CARTESIAN_POINT('Ctrl Pts',(4.95339743589733,0.53275779311414,-3.08264413157538));
#14548=CARTESIAN_POINT('Ctrl Pts',(4.96910256410267,0.687495327956871,-3.0519995880578));
#14549=CARTESIAN_POINT('Ctrl Pts',(4.98480769230783,0.839080192893056,-3.00992620370386));
#14550=CARTESIAN_POINT('Ctrl Pts',(4.99737175038973,0.960347655502346,-2.97626761538679));
#14551=CARTESIAN_POINT('Ctrl Pts',(5.00993580847151,1.07960443666828,-2.93528882778825));
#14552=CARTESIAN_POINT('Ctrl Pts',(5.02249986655329,1.19588572614116,-2.887123539098));
#14553=CARTESIAN_POINT('Ctrl Pts',(5.02564093667654,1.22495656311742,-2.8750820037678));
#14554=CARTESIAN_POINT('Ctrl Pts',(5.02878200679978,1.25384145182002,-2.86259139598291));
#14555=CARTESIAN_POINT('Ctrl Pts',(5.03192307692303,1.28252819003516,-2.84966078036119));
#14556=CARTESIAN_POINT('Ctrl Pts',(5.04762820512805,1.42595984987577,-2.78500861783667));
#14557=CARTESIAN_POINT('Ctrl Pts',(5.06333333333311,1.56441436952739,-2.70936700040773));
#14558=CARTESIAN_POINT('Ctrl Pts',(5.07903846153833,1.69644712969505,-2.62385329049029));
#14559=CARTESIAN_POINT('Ctrl Pts',(5.09474358974339,1.82847988986133,-2.53833958057375));
#14560=CARTESIAN_POINT('Ctrl Pts',(5.11044871794861,1.95410534229508,-2.44294922198321));
#14561=CARTESIAN_POINT('Ctrl Pts',(5.12615384615367,2.07193616153302,-2.33873186210924));
#14562=CARTESIAN_POINT('Ctrl Pts',(5.14185897435889,2.18976698077217,-2.23451450223419));
#14563=CARTESIAN_POINT('Ctrl Pts',(5.15756410256395,2.29981131668746,-2.12145732421479));
#14564=CARTESIAN_POINT('Ctrl Pts',(5.17326923076914,2.40059929676421,-2.00064999697507));
#14565=CARTESIAN_POINT('Ctrl Pts',(5.17609619372183,2.4187413890815,-1.97890437133877));
#14566=CARTESIAN_POINT('Ctrl Pts',(5.17892315667452,2.43658301180573,-1.95690831774611));
#14567=CARTESIAN_POINT('Ctrl Pts',(5.18175011962722,2.45411540900217,-1.93466859159333));
#14568=CARTESIAN_POINT('Ctrl Pts',(5.19462828487976,2.53398384454479,-1.83335602635671));
#14569=CARTESIAN_POINT('Ctrl Pts',(5.20750645013235,2.60743359059156,-1.72698578057499));
#14570=CARTESIAN_POINT('Ctrl Pts',(5.22038461538483,2.67404531641152,-1.61651716219696));
#14571=CARTESIAN_POINT('Ctrl Pts',(5.23608974359,2.75527937991824,-1.48179891776846));
#14572=CARTESIAN_POINT('Ctrl Pts',(5.251794871795,2.82635571584921,-1.34097710458914));
#14573=CARTESIAN_POINT('Ctrl Pts',(5.2675,2.886585772757,-1.1956628320182));
#14574=CARTESIAN_POINT('Ctrl Pts',(5.283205128205,2.94681582966478,-1.05034855944727));
#14575=CARTESIAN_POINT('Ctrl Pts',(5.29891025641,2.99620426616756,-0.900527828411028));
#14576=CARTESIAN_POINT('Ctrl Pts',(5.31461538461517,3.03402009771089,-0.747818590164115));
#14577=CARTESIAN_POINT('Ctrl Pts',(5.323410232868,3.05519690668903,-0.662301645657758));
#14578=CARTESIAN_POINT('Ctrl Pts',(5.33220508112087,3.07274362189333,-0.575877627491407));
#14579=CARTESIAN_POINT('Ctrl Pts',(5.34099992937375,3.0865260643595,-0.488857703250828));
#14580=CARTESIAN_POINT('Ctrl Pts',(5.34791020932613,3.09735519217733,-0.420484489677707));
#14581=CARTESIAN_POINT('Ctrl Pts',(5.35482048927851,3.1058605533367,-0.351743453374755));
#14582=CARTESIAN_POINT('Ctrl Pts',(5.36173076923086,3.11205714799649,-0.282798238157759));
#14583=CARTESIAN_POINT('Ctrl Pts',(5.37743589743605,3.12614026969903,-0.126105101036853));
#14584=CARTESIAN_POINT('Ctrl Pts',(5.39314102564111,3.12830002883755,0.0316368087400967));
#14585=CARTESIAN_POINT('Ctrl Pts',(5.40884615384633,3.11873422241136,0.188648419771248));
#14586=CARTESIAN_POINT('Ctrl Pts',(5.42455128205139,3.10916841598526,0.345660030800768));
#14587=CARTESIAN_POINT('Ctrl Pts',(5.44025641025661,3.08787818772652,0.501956134080478));
#14588=CARTESIAN_POINT('Ctrl Pts',(5.45596153846167,3.05502438429764,0.655798952750868));
#14589=CARTESIAN_POINT('Ctrl Pts',(5.47072435081943,3.02414182613405,0.80041112241712));
#14590=CARTESIAN_POINT('Ctrl Pts',(5.48548716317704,2.98303392179022,0.942866889012676));
#14591=CARTESIAN_POINT('Ctrl Pts',(5.50024997553463,2.93184792475783,1.08161580336684));
#14592=CARTESIAN_POINT('Ctrl Pts',(5.50119229138207,2.92858070337733,1.09047219858784));
#14593=CARTESIAN_POINT('Ctrl Pts',(5.50213460722953,2.92527242968113,1.09931349244539));
#14594=CARTESIAN_POINT('Ctrl Pts',(5.50307692307697,2.92192333127633,1.10813935100346));
#14595=CARTESIAN_POINT('Ctrl Pts',(5.518782051282,2.8661055076018,1.25523572060092));
#14596=CARTESIAN_POINT('Ctrl Pts',(5.534487179487,2.79895807188958,1.3980126906426));
#14597=CARTESIAN_POINT('Ctrl Pts',(5.55019230769217,2.72154967470353,1.53495847225753));
#14598=CARTESIAN_POINT('Ctrl Pts',(5.56589743589733,2.64414127751749,1.67190425387245));
#14599=CARTESIAN_POINT('Ctrl Pts',(5.58160256410267,2.55646931412381,1.80303404218782));
#14600=CARTESIAN_POINT('Ctrl Pts',(5.59730769230783,2.45953351178131,1.92692186650602));
#14601=CARTESIAN_POINT('Ctrl Pts',(5.613012820513,2.3625977094388,2.05080969082422));
#14602=CARTESIAN_POINT('Ctrl Pts',(5.628717948718,2.25638664196914,2.16746520831446));
#14603=CARTESIAN_POINT('Ctrl Pts',(5.64442307692303,2.14191592065938,2.27539299236912));
#14604=CARTESIAN_POINT('Ctrl Pts',(5.64944877282191,2.10528488988284,2.30993026036321));
#14605=CARTESIAN_POINT('Ctrl Pts',(5.65447446872079,2.0678091870461,2.34357256496936));
#14606=CARTESIAN_POINT('Ctrl Pts',(5.65950016461967,2.02952515103173,2.37626864249984));
#14607=CARTESIAN_POINT('Ctrl Pts',(5.67017959692584,1.94817288076942,2.44574669164748));
#14608=CARTESIAN_POINT('Ctrl Pts',(5.68085902923205,1.86317013579029,2.51095134091135));
#14609=CARTESIAN_POINT('Ctrl Pts',(5.69153846153833,1.7750601494579,2.57161807835228));
#14610=CARTESIAN_POINT('Ctrl Pts',(5.70724358974339,1.64548597436975,2.66083432711599));
#14611=CARTESIAN_POINT('Ctrl Pts',(5.72294871794861,1.509186930649,2.74024633660057));
#14612=CARTESIAN_POINT('Ctrl Pts',(5.73865384615367,1.36775803719504,2.80910392412142));
#14613=CARTESIAN_POINT('Ctrl Pts',(5.75435897435889,1.22632914373961,2.87796151164299));
#14614=CARTESIAN_POINT('Ctrl Pts',(5.77006410256395,1.07975715593558,2.9362712759061));
#14615=CARTESIAN_POINT('Ctrl Pts',(5.78576923076914,0.929617596829541,2.98324879794393));
#14616=CARTESIAN_POINT('Ctrl Pts',(5.7967627558717,0.82452052341797,3.01613287001461));
#14617=CARTESIAN_POINT('Ctrl Pts',(5.80775628097433,0.717669381189646,3.04346332885533));
#14618=CARTESIAN_POINT('Ctrl Pts',(5.81874980607692,0.609657256300376,3.06495400126008));
#14619=CARTESIAN_POINT('Ctrl Pts',(5.82346140917957,0.563365438343646,3.07416446995282));
#14620=CARTESIAN_POINT('Ctrl Pts',(5.82817301228221,0.516860431844721,3.08230245321972));
#14621=CARTESIAN_POINT('Ctrl Pts',(5.83288461538483,0.470193579471047,3.08937038670253));
#14622=CARTESIAN_POINT('Ctrl Pts',(5.84858974359,0.31463953905291,3.112929841749));
#14623=CARTESIAN_POINT('Ctrl Pts',(5.864294871795,0.157306535044493,3.12459764304402));
#14624=CARTESIAN_POINT('Ctrl Pts',(5.88,3.21695909424879E-7,3.12449703095644));
#14625=CARTESIAN_POINT('Ctrl Pts',(1.170978862952,-0.9656781074217,-2.972051613422));
#14626=CARTESIAN_POINT('Ctrl Pts',(1.224062196285,-0.4599252670358,-3.136380672689));
#14627=CARTESIAN_POINT('Ctrl Pts',(1.330228862952,0.6366272854614,-3.200971110614));
#14628=CARTESIAN_POINT('Ctrl Pts',(1.489478862952,2.119635939241,-2.481754111378));
#14629=CARTESIAN_POINT('Ctrl Pts',(1.648728862952,3.061979863765,-1.129624298873));
#14630=CARTESIAN_POINT('Ctrl Pts',(1.807978862952,3.223532154246,0.5105564866689));
#14631=CARTESIAN_POINT('Ctrl Pts',(1.967228862952,2.563047905408,2.020544571702));
#14632=CARTESIAN_POINT('Ctrl Pts',(2.126478862952,1.248968678135,3.015276776083));
#14633=CARTESIAN_POINT('Ctrl Pts',(2.285728862952,-0.383608261101,3.241089558554));
#14634=CARTESIAN_POINT('Ctrl Pts',(2.444978862952,-1.918361836065,2.640398557608));
#14635=CARTESIAN_POINT('Ctrl Pts',(2.604228862952,-2.963917875123,1.366384855545));
#14636=CARTESIAN_POINT('Ctrl Pts',(2.763478862952,-3.253651172662,-0.256067900963));
#14637=CARTESIAN_POINT('Ctrl Pts',(2.922728862952,-2.713677441724,-1.813221296591));
#14638=CARTESIAN_POINT('Ctrl Pts',(3.081978862952,-1.481694291113,-2.907988781792));
#14639=CARTESIAN_POINT('Ctrl Pts',(3.241228862952,0.1281327360592,-3.261195904774));
#14640=CARTESIAN_POINT('Ctrl Pts',(3.400478862952,1.705284892359,-2.782772028626));
#14641=CARTESIAN_POINT('Ctrl Pts',(3.559728862952,2.84757578293,-1.59471906236));
#14642=CARTESIAN_POINT('Ctrl Pts',(3.718978862952,3.263712108535,0.));
#14643=CARTESIAN_POINT('Ctrl Pts',(3.878228862952,2.84757578293,1.59471906236));
#14644=CARTESIAN_POINT('Ctrl Pts',(4.037478862952,1.705284892359,2.782772028626));
#14645=CARTESIAN_POINT('Ctrl Pts',(4.196728862952,0.1281327360592,3.261195904774));
#14646=CARTESIAN_POINT('Ctrl Pts',(4.355978862952,-1.481694291113,2.907988781792));
#14647=CARTESIAN_POINT('Ctrl Pts',(4.515228862952,-2.713677441724,1.813221296591));
#14648=CARTESIAN_POINT('Ctrl Pts',(4.674478862952,-3.253651172662,0.256067900963));
#14649=CARTESIAN_POINT('Ctrl Pts',(4.833728862952,-2.963917875123,-1.366384855545));
#14650=CARTESIAN_POINT('Ctrl Pts',(4.992978862952,-1.918361836065,-2.640398557608));
#14651=CARTESIAN_POINT('Ctrl Pts',(5.152228862952,-0.383608261101,-3.241089558554));
#14652=CARTESIAN_POINT('Ctrl Pts',(5.311478862952,1.248968678135,-3.015276776083));
#14653=CARTESIAN_POINT('Ctrl Pts',(5.470728862952,2.563047905408,-2.020544571702));
#14654=CARTESIAN_POINT('Ctrl Pts',(5.629978862952,3.223532154246,-0.510556486669));
#14655=CARTESIAN_POINT('Ctrl Pts',(5.789228862952,3.061979863765,1.129624298873));
#14656=CARTESIAN_POINT('Ctrl Pts',(5.948478862952,2.119635939241,2.481754111378));
#14657=CARTESIAN_POINT('Ctrl Pts',(6.107728862952,0.6366272854614,3.200971110614));
#14658=CARTESIAN_POINT('Ctrl Pts',(6.213895529618,-0.4599252670358,3.136380672689));
#14659=CARTESIAN_POINT('Ctrl Pts',(6.266978862952,-0.9656781074217,2.972051613422));
#14660=CARTESIAN_POINT('Ctrl Pts',(1.059992954317,-0.9656781074217,-2.972051613422));
#14661=CARTESIAN_POINT('Ctrl Pts',(1.113076287651,-0.4599252670358,-3.136380672689));
#14662=CARTESIAN_POINT('Ctrl Pts',(1.219242954317,0.6366272854614,-3.200971110614));
#14663=CARTESIAN_POINT('Ctrl Pts',(1.378492954317,2.119635939241,-2.481754111378));
#14664=CARTESIAN_POINT('Ctrl Pts',(1.537742954317,3.061979863765,-1.129624298873));
#14665=CARTESIAN_POINT('Ctrl Pts',(1.696992954317,3.223532154246,0.5105564866689));
#14666=CARTESIAN_POINT('Ctrl Pts',(1.856242954317,2.563047905408,2.020544571702));
#14667=CARTESIAN_POINT('Ctrl Pts',(2.015492954317,1.248968678135,3.015276776083));
#14668=CARTESIAN_POINT('Ctrl Pts',(2.174742954317,-0.383608261101,3.241089558554));
#14669=CARTESIAN_POINT('Ctrl Pts',(2.333992954317,-1.918361836065,2.640398557608));
#14670=CARTESIAN_POINT('Ctrl Pts',(2.493242954317,-2.963917875123,1.366384855545));
#14671=CARTESIAN_POINT('Ctrl Pts',(2.652492954317,-3.253651172662,-0.256067900963));
#14672=CARTESIAN_POINT('Ctrl Pts',(2.811742954317,-2.713677441724,-1.813221296591));
#14673=CARTESIAN_POINT('Ctrl Pts',(2.970992954317,-1.481694291113,-2.907988781792));
#14674=CARTESIAN_POINT('Ctrl Pts',(3.130242954317,0.1281327360592,-3.261195904774));
#14675=CARTESIAN_POINT('Ctrl Pts',(3.289492954317,1.705284892359,-2.782772028626));
#14676=CARTESIAN_POINT('Ctrl Pts',(3.448742954317,2.84757578293,-1.59471906236));
#14677=CARTESIAN_POINT('Ctrl Pts',(3.607992954317,3.263712108535,0.));
#14678=CARTESIAN_POINT('Ctrl Pts',(3.767242954317,2.84757578293,1.59471906236));
#14679=CARTESIAN_POINT('Ctrl Pts',(3.926492954317,1.705284892359,2.782772028626));
#14680=CARTESIAN_POINT('Ctrl Pts',(4.085742954317,0.1281327360592,3.261195904774));
#14681=CARTESIAN_POINT('Ctrl Pts',(4.244992954317,-1.481694291113,2.907988781792));
#14682=CARTESIAN_POINT('Ctrl Pts',(4.404242954317,-2.713677441724,1.813221296591));
#14683=CARTESIAN_POINT('Ctrl Pts',(4.563492954317,-3.253651172662,0.256067900963));
#14684=CARTESIAN_POINT('Ctrl Pts',(4.722742954317,-2.963917875123,-1.366384855545));
#14685=CARTESIAN_POINT('Ctrl Pts',(4.881992954317,-1.918361836065,-2.640398557608));
#14686=CARTESIAN_POINT('Ctrl Pts',(5.041242954317,-0.383608261101,-3.241089558554));
#14687=CARTESIAN_POINT('Ctrl Pts',(5.200492954317,1.248968678135,-3.015276776083));
#14688=CARTESIAN_POINT('Ctrl Pts',(5.359742954317,2.563047905408,-2.020544571702));
#14689=CARTESIAN_POINT('Ctrl Pts',(5.518992954317,3.223532154246,-0.510556486669));
#14690=CARTESIAN_POINT('Ctrl Pts',(5.678242954317,3.061979863765,1.129624298873));
#14691=CARTESIAN_POINT('Ctrl Pts',(5.837492954317,2.119635939241,2.481754111378));
#14692=CARTESIAN_POINT('Ctrl Pts',(5.996742954317,0.6366272854614,3.200971110614));
#14693=CARTESIAN_POINT('Ctrl Pts',(6.102909620984,-0.4599252670358,3.136380672689));
#14694=CARTESIAN_POINT('Ctrl Pts',(6.155992954317,-0.9656781074217,2.972051613422));
#14695=CARTESIAN_POINT('Ctrl Pts',(0.9490070456828,-0.9656781074217,-2.972051613422));
#14696=CARTESIAN_POINT('Ctrl Pts',(1.002090379016,-0.4599252670358,-3.136380672689));
#14697=CARTESIAN_POINT('Ctrl Pts',(1.108257045683,0.6366272854614,-3.200971110614));
#14698=CARTESIAN_POINT('Ctrl Pts',(1.267507045683,2.119635939241,-2.481754111378));
#14699=CARTESIAN_POINT('Ctrl Pts',(1.426757045683,3.061979863765,-1.129624298873));
#14700=CARTESIAN_POINT('Ctrl Pts',(1.586007045683,3.223532154246,0.5105564866689));
#14701=CARTESIAN_POINT('Ctrl Pts',(1.745257045683,2.563047905408,2.020544571702));
#14702=CARTESIAN_POINT('Ctrl Pts',(1.904507045683,1.248968678135,3.015276776083));
#14703=CARTESIAN_POINT('Ctrl Pts',(2.063757045683,-0.383608261101,3.241089558554));
#14704=CARTESIAN_POINT('Ctrl Pts',(2.223007045683,-1.918361836065,2.640398557608));
#14705=CARTESIAN_POINT('Ctrl Pts',(2.382257045683,-2.963917875123,1.366384855545));
#14706=CARTESIAN_POINT('Ctrl Pts',(2.541507045683,-3.253651172662,-0.256067900963));
#14707=CARTESIAN_POINT('Ctrl Pts',(2.700757045683,-2.713677441724,-1.813221296591));
#14708=CARTESIAN_POINT('Ctrl Pts',(2.860007045683,-1.481694291113,-2.907988781792));
#14709=CARTESIAN_POINT('Ctrl Pts',(3.019257045683,0.1281327360592,-3.261195904774));
#14710=CARTESIAN_POINT('Ctrl Pts',(3.178507045683,1.705284892359,-2.782772028626));
#14711=CARTESIAN_POINT('Ctrl Pts',(3.337757045683,2.84757578293,-1.59471906236));
#14712=CARTESIAN_POINT('Ctrl Pts',(3.497007045683,3.263712108535,0.));
#14713=CARTESIAN_POINT('Ctrl Pts',(3.656257045683,2.84757578293,1.59471906236));
#14714=CARTESIAN_POINT('Ctrl Pts',(3.815507045683,1.705284892359,2.782772028626));
#14715=CARTESIAN_POINT('Ctrl Pts',(3.974757045683,0.1281327360592,3.261195904774));
#14716=CARTESIAN_POINT('Ctrl Pts',(4.134007045683,-1.481694291113,2.907988781792));
#14717=CARTESIAN_POINT('Ctrl Pts',(4.293257045683,-2.713677441724,1.813221296591));
#14718=CARTESIAN_POINT('Ctrl Pts',(4.452507045683,-3.253651172662,0.256067900963));
#14719=CARTESIAN_POINT('Ctrl Pts',(4.611757045683,-2.963917875123,-1.366384855545));
#14720=CARTESIAN_POINT('Ctrl Pts',(4.771007045683,-1.918361836065,-2.640398557608));
#14721=CARTESIAN_POINT('Ctrl Pts',(4.930257045683,-0.383608261101,-3.241089558554));
#14722=CARTESIAN_POINT('Ctrl Pts',(5.089507045683,1.248968678135,-3.015276776083));
#14723=CARTESIAN_POINT('Ctrl Pts',(5.248757045683,2.563047905408,-2.020544571702));
#14724=CARTESIAN_POINT('Ctrl Pts',(5.408007045683,3.223532154246,-0.510556486669));
#14725=CARTESIAN_POINT('Ctrl Pts',(5.567257045683,3.061979863765,1.129624298873));
#14726=CARTESIAN_POINT('Ctrl Pts',(5.726507045683,2.119635939241,2.481754111378));
#14727=CARTESIAN_POINT('Ctrl Pts',(5.885757045683,0.6366272854614,3.200971110614));
#14728=CARTESIAN_POINT('Ctrl Pts',(5.991923712349,-0.4599252670358,3.136380672689));
#14729=CARTESIAN_POINT('Ctrl Pts',(6.045007045683,-0.9656781074217,2.972051613422));
#14730=CARTESIAN_POINT('Ctrl Pts',(0.8380211370484,-0.9656781074217,-2.972051613422));
#14731=CARTESIAN_POINT('Ctrl Pts',(0.8911044703817,-0.4599252670358,-3.136380672689));
#14732=CARTESIAN_POINT('Ctrl Pts',(0.9972711370484,0.6366272854614,-3.200971110614));
#14733=CARTESIAN_POINT('Ctrl Pts',(1.156521137048,2.119635939241,-2.481754111378));
#14734=CARTESIAN_POINT('Ctrl Pts',(1.315771137048,3.061979863765,-1.129624298873));
#14735=CARTESIAN_POINT('Ctrl Pts',(1.475021137048,3.223532154246,0.5105564866689));
#14736=CARTESIAN_POINT('Ctrl Pts',(1.634271137048,2.563047905408,2.020544571702));
#14737=CARTESIAN_POINT('Ctrl Pts',(1.793521137048,1.248968678135,3.015276776083));
#14738=CARTESIAN_POINT('Ctrl Pts',(1.952771137048,-0.383608261101,3.241089558554));
#14739=CARTESIAN_POINT('Ctrl Pts',(2.112021137048,-1.918361836065,2.640398557608));
#14740=CARTESIAN_POINT('Ctrl Pts',(2.271271137048,-2.963917875123,1.366384855545));
#14741=CARTESIAN_POINT('Ctrl Pts',(2.430521137048,-3.253651172662,-0.256067900963));
#14742=CARTESIAN_POINT('Ctrl Pts',(2.589771137048,-2.713677441724,-1.813221296591));
#14743=CARTESIAN_POINT('Ctrl Pts',(2.749021137048,-1.481694291113,-2.907988781792));
#14744=CARTESIAN_POINT('Ctrl Pts',(2.908271137048,0.1281327360592,-3.261195904774));
#14745=CARTESIAN_POINT('Ctrl Pts',(3.067521137048,1.705284892359,-2.782772028626));
#14746=CARTESIAN_POINT('Ctrl Pts',(3.226771137048,2.84757578293,-1.59471906236));
#14747=CARTESIAN_POINT('Ctrl Pts',(3.386021137048,3.263712108535,0.));
#14748=CARTESIAN_POINT('Ctrl Pts',(3.545271137048,2.84757578293,1.59471906236));
#14749=CARTESIAN_POINT('Ctrl Pts',(3.704521137048,1.705284892359,2.782772028626));
#14750=CARTESIAN_POINT('Ctrl Pts',(3.863771137048,0.1281327360592,3.261195904774));
#14751=CARTESIAN_POINT('Ctrl Pts',(4.023021137048,-1.481694291113,2.907988781792));
#14752=CARTESIAN_POINT('Ctrl Pts',(4.182271137048,-2.713677441724,1.813221296591));
#14753=CARTESIAN_POINT('Ctrl Pts',(4.341521137048,-3.253651172662,0.256067900963));
#14754=CARTESIAN_POINT('Ctrl Pts',(4.500771137048,-2.963917875123,-1.366384855545));
#14755=CARTESIAN_POINT('Ctrl Pts',(4.660021137048,-1.918361836065,-2.640398557608));
#14756=CARTESIAN_POINT('Ctrl Pts',(4.819271137048,-0.383608261101,-3.241089558554));
#14757=CARTESIAN_POINT('Ctrl Pts',(4.978521137048,1.248968678135,-3.015276776083));
#14758=CARTESIAN_POINT('Ctrl Pts',(5.137771137048,2.563047905408,-2.020544571702));
#14759=CARTESIAN_POINT('Ctrl Pts',(5.297021137048,3.223532154246,-0.510556486669));
#14760=CARTESIAN_POINT('Ctrl Pts',(5.456271137048,3.061979863765,1.129624298873));
#14761=CARTESIAN_POINT('Ctrl Pts',(5.615521137048,2.119635939241,2.481754111378));
#14762=CARTESIAN_POINT('Ctrl Pts',(5.774771137048,0.6366272854614,3.200971110614));
#14763=CARTESIAN_POINT('Ctrl Pts',(5.880937803715,-0.4599252670358,3.136380672689));
#14764=CARTESIAN_POINT('Ctrl Pts',(5.934021137048,-0.9656781074217,2.972051613422));
#14765=CARTESIAN_POINT('',(6.125,0.,3.125));
#14766=CARTESIAN_POINT('Ctrl Pts',(6.070978862952,0.9656781074217,2.972051613422));
#14767=CARTESIAN_POINT('Ctrl Pts',(6.124062196285,0.4599252670358,3.136380672689));
#14768=CARTESIAN_POINT('Ctrl Pts',(6.230228862952,-0.6366272854614,3.200971110614));
#14769=CARTESIAN_POINT('Ctrl Pts',(6.389478862952,-2.119635939241,2.481754111378));
#14770=CARTESIAN_POINT('Ctrl Pts',(6.548728862952,-3.061979863765,1.129624298873));
#14771=CARTESIAN_POINT('Ctrl Pts',(6.707978862952,-3.223532154246,-0.5105564866689));
#14772=CARTESIAN_POINT('Ctrl Pts',(6.867228862952,-2.563047905408,-2.020544571702));
#14773=CARTESIAN_POINT('Ctrl Pts',(7.026478862952,-1.248968678135,-3.015276776083));
#14774=CARTESIAN_POINT('Ctrl Pts',(7.185728862952,0.383608261101,-3.241089558554));
#14775=CARTESIAN_POINT('Ctrl Pts',(7.344978862952,1.918361836065,-2.640398557608));
#14776=CARTESIAN_POINT('Ctrl Pts',(7.504228862952,2.963917875123,-1.366384855545));
#14777=CARTESIAN_POINT('Ctrl Pts',(7.663478862952,3.253651172662,0.256067900963));
#14778=CARTESIAN_POINT('Ctrl Pts',(7.822728862952,2.713677441724,1.813221296591));
#14779=CARTESIAN_POINT('Ctrl Pts',(7.981978862952,1.481694291113,2.907988781792));
#14780=CARTESIAN_POINT('Ctrl Pts',(8.141228862952,-0.1281327360592,3.261195904774));
#14781=CARTESIAN_POINT('Ctrl Pts',(8.300478862952,-1.705284892359,2.782772028626));
#14782=CARTESIAN_POINT('Ctrl Pts',(8.459728862952,-2.84757578293,1.59471906236));
#14783=CARTESIAN_POINT('Ctrl Pts',(8.618978862952,-3.263712108535,0.));
#14784=CARTESIAN_POINT('Ctrl Pts',(8.778228862952,-2.84757578293,-1.59471906236));
#14785=CARTESIAN_POINT('Ctrl Pts',(8.937478862952,-1.705284892359,-2.782772028626));
#14786=CARTESIAN_POINT('Ctrl Pts',(9.096728862952,-0.1281327360592,-3.261195904774));
#14787=CARTESIAN_POINT('Ctrl Pts',(9.255978862952,1.481694291113,-2.907988781792));
#14788=CARTESIAN_POINT('Ctrl Pts',(9.415228862952,2.713677441724,-1.813221296591));
#14789=CARTESIAN_POINT('Ctrl Pts',(9.574478862952,3.253651172662,-0.256067900963));
#14790=CARTESIAN_POINT('Ctrl Pts',(9.733728862952,2.963917875123,1.366384855545));
#14791=CARTESIAN_POINT('Ctrl Pts',(9.892978862952,1.918361836065,2.640398557608));
#14792=CARTESIAN_POINT('Ctrl Pts',(10.05222886295,0.383608261101,3.241089558554));
#14793=CARTESIAN_POINT('Ctrl Pts',(10.21147886295,-1.248968678135,3.015276776083));
#14794=CARTESIAN_POINT('Ctrl Pts',(10.37072886295,-2.563047905408,2.020544571702));
#14795=CARTESIAN_POINT('Ctrl Pts',(10.52997886295,-3.223532154246,0.5105564866689));
#14796=CARTESIAN_POINT('Ctrl Pts',(10.68922886295,-3.061979863765,-1.129624298873));
#14797=CARTESIAN_POINT('Ctrl Pts',(10.84847886295,-2.119635939241,-2.481754111378));
#14798=CARTESIAN_POINT('Ctrl Pts',(11.00772886295,-0.6366272854614,-3.200971110614));
#14799=CARTESIAN_POINT('Ctrl Pts',(11.11389552962,0.4599252670358,-3.136380672689));
#14800=CARTESIAN_POINT('Ctrl Pts',(11.16697886295,0.9656781074217,-2.972051613422));
#14801=CARTESIAN_POINT('Ctrl Pts',(5.959992954317,0.9656781074217,2.972051613422));
#14802=CARTESIAN_POINT('Ctrl Pts',(6.013076287651,0.4599252670358,3.136380672689));
#14803=CARTESIAN_POINT('Ctrl Pts',(6.119242954317,-0.6366272854614,3.200971110614));
#14804=CARTESIAN_POINT('Ctrl Pts',(6.278492954317,-2.119635939241,2.481754111378));
#14805=CARTESIAN_POINT('Ctrl Pts',(6.437742954317,-3.061979863765,1.129624298873));
#14806=CARTESIAN_POINT('Ctrl Pts',(6.596992954317,-3.223532154246,-0.5105564866689));
#14807=CARTESIAN_POINT('Ctrl Pts',(6.756242954317,-2.563047905408,-2.020544571702));
#14808=CARTESIAN_POINT('Ctrl Pts',(6.915492954317,-1.248968678135,-3.015276776083));
#14809=CARTESIAN_POINT('Ctrl Pts',(7.074742954317,0.383608261101,-3.241089558554));
#14810=CARTESIAN_POINT('Ctrl Pts',(7.233992954317,1.918361836065,-2.640398557608));
#14811=CARTESIAN_POINT('Ctrl Pts',(7.393242954317,2.963917875123,-1.366384855545));
#14812=CARTESIAN_POINT('Ctrl Pts',(7.552492954317,3.253651172662,0.256067900963));
#14813=CARTESIAN_POINT('Ctrl Pts',(7.711742954317,2.713677441724,1.813221296591));
#14814=CARTESIAN_POINT('Ctrl Pts',(7.870992954317,1.481694291113,2.907988781792));
#14815=CARTESIAN_POINT('Ctrl Pts',(8.030242954317,-0.1281327360592,3.261195904774));
#14816=CARTESIAN_POINT('Ctrl Pts',(8.189492954317,-1.705284892359,2.782772028626));
#14817=CARTESIAN_POINT('Ctrl Pts',(8.348742954317,-2.84757578293,1.59471906236));
#14818=CARTESIAN_POINT('Ctrl Pts',(8.507992954317,-3.263712108535,0.));
#14819=CARTESIAN_POINT('Ctrl Pts',(8.667242954317,-2.84757578293,-1.59471906236));
#14820=CARTESIAN_POINT('Ctrl Pts',(8.826492954317,-1.705284892359,-2.782772028626));
#14821=CARTESIAN_POINT('Ctrl Pts',(8.985742954317,-0.1281327360592,-3.261195904774));
#14822=CARTESIAN_POINT('Ctrl Pts',(9.144992954317,1.481694291113,-2.907988781792));
#14823=CARTESIAN_POINT('Ctrl Pts',(9.304242954317,2.713677441724,-1.813221296591));
#14824=CARTESIAN_POINT('Ctrl Pts',(9.463492954317,3.253651172662,-0.256067900963));
#14825=CARTESIAN_POINT('Ctrl Pts',(9.622742954317,2.963917875123,1.366384855545));
#14826=CARTESIAN_POINT('Ctrl Pts',(9.781992954317,1.918361836065,2.640398557608));
#14827=CARTESIAN_POINT('Ctrl Pts',(9.941242954317,0.383608261101,3.241089558554));
#14828=CARTESIAN_POINT('Ctrl Pts',(10.10049295432,-1.248968678135,3.015276776083));
#14829=CARTESIAN_POINT('Ctrl Pts',(10.25974295432,-2.563047905408,2.020544571702));
#14830=CARTESIAN_POINT('Ctrl Pts',(10.41899295432,-3.223532154246,0.5105564866689));
#14831=CARTESIAN_POINT('Ctrl Pts',(10.57824295432,-3.061979863765,-1.129624298873));
#14832=CARTESIAN_POINT('Ctrl Pts',(10.73749295432,-2.119635939241,-2.481754111378));
#14833=CARTESIAN_POINT('Ctrl Pts',(10.89674295432,-0.6366272854614,-3.200971110614));
#14834=CARTESIAN_POINT('Ctrl Pts',(11.00290962098,0.4599252670358,-3.136380672689));
#14835=CARTESIAN_POINT('Ctrl Pts',(11.05599295432,0.9656781074217,-2.972051613422));
#14836=CARTESIAN_POINT('Ctrl Pts',(5.849007045683,0.9656781074217,2.972051613422));
#14837=CARTESIAN_POINT('Ctrl Pts',(5.902090379016,0.4599252670358,3.136380672689));
#14838=CARTESIAN_POINT('Ctrl Pts',(6.008257045683,-0.6366272854614,3.200971110614));
#14839=CARTESIAN_POINT('Ctrl Pts',(6.167507045683,-2.119635939241,2.481754111378));
#14840=CARTESIAN_POINT('Ctrl Pts',(6.326757045683,-3.061979863765,1.129624298873));
#14841=CARTESIAN_POINT('Ctrl Pts',(6.486007045683,-3.223532154246,-0.5105564866689));
#14842=CARTESIAN_POINT('Ctrl Pts',(6.645257045683,-2.563047905408,-2.020544571702));
#14843=CARTESIAN_POINT('Ctrl Pts',(6.804507045683,-1.248968678135,-3.015276776083));
#14844=CARTESIAN_POINT('Ctrl Pts',(6.963757045683,0.383608261101,-3.241089558554));
#14845=CARTESIAN_POINT('Ctrl Pts',(7.123007045683,1.918361836065,-2.640398557608));
#14846=CARTESIAN_POINT('Ctrl Pts',(7.282257045683,2.963917875123,-1.366384855545));
#14847=CARTESIAN_POINT('Ctrl Pts',(7.441507045683,3.253651172662,0.256067900963));
#14848=CARTESIAN_POINT('Ctrl Pts',(7.600757045683,2.713677441724,1.813221296591));
#14849=CARTESIAN_POINT('Ctrl Pts',(7.760007045683,1.481694291113,2.907988781792));
#14850=CARTESIAN_POINT('Ctrl Pts',(7.919257045683,-0.1281327360592,3.261195904774));
#14851=CARTESIAN_POINT('Ctrl Pts',(8.078507045683,-1.705284892359,2.782772028626));
#14852=CARTESIAN_POINT('Ctrl Pts',(8.237757045683,-2.84757578293,1.59471906236));
#14853=CARTESIAN_POINT('Ctrl Pts',(8.397007045683,-3.263712108535,0.));
#14854=CARTESIAN_POINT('Ctrl Pts',(8.556257045683,-2.84757578293,-1.59471906236));
#14855=CARTESIAN_POINT('Ctrl Pts',(8.715507045683,-1.705284892359,-2.782772028626));
#14856=CARTESIAN_POINT('Ctrl Pts',(8.874757045683,-0.1281327360592,-3.261195904774));
#14857=CARTESIAN_POINT('Ctrl Pts',(9.034007045683,1.481694291113,-2.907988781792));
#14858=CARTESIAN_POINT('Ctrl Pts',(9.193257045683,2.713677441724,-1.813221296591));
#14859=CARTESIAN_POINT('Ctrl Pts',(9.352507045683,3.253651172662,-0.256067900963));
#14860=CARTESIAN_POINT('Ctrl Pts',(9.511757045683,2.963917875123,1.366384855545));
#14861=CARTESIAN_POINT('Ctrl Pts',(9.671007045683,1.918361836065,2.640398557608));
#14862=CARTESIAN_POINT('Ctrl Pts',(9.830257045683,0.383608261101,3.241089558554));
#14863=CARTESIAN_POINT('Ctrl Pts',(9.989507045683,-1.248968678135,3.015276776083));
#14864=CARTESIAN_POINT('Ctrl Pts',(10.14875704568,-2.563047905408,2.020544571702));
#14865=CARTESIAN_POINT('Ctrl Pts',(10.30800704568,-3.223532154246,0.5105564866689));
#14866=CARTESIAN_POINT('Ctrl Pts',(10.46725704568,-3.061979863765,-1.129624298873));
#14867=CARTESIAN_POINT('Ctrl Pts',(10.62650704568,-2.119635939241,-2.481754111378));
#14868=CARTESIAN_POINT('Ctrl Pts',(10.78575704568,-0.6366272854614,-3.200971110614));
#14869=CARTESIAN_POINT('Ctrl Pts',(10.89192371235,0.4599252670358,-3.136380672689));
#14870=CARTESIAN_POINT('Ctrl Pts',(10.94500704568,0.9656781074217,-2.972051613422));
#14871=CARTESIAN_POINT('Ctrl Pts',(5.738021137048,0.9656781074217,2.972051613422));
#14872=CARTESIAN_POINT('Ctrl Pts',(5.791104470382,0.4599252670358,3.136380672689));
#14873=CARTESIAN_POINT('Ctrl Pts',(5.897271137048,-0.6366272854614,3.200971110614));
#14874=CARTESIAN_POINT('Ctrl Pts',(6.056521137048,-2.119635939241,2.481754111378));
#14875=CARTESIAN_POINT('Ctrl Pts',(6.215771137048,-3.061979863765,1.129624298873));
#14876=CARTESIAN_POINT('Ctrl Pts',(6.375021137048,-3.223532154246,-0.5105564866689));
#14877=CARTESIAN_POINT('Ctrl Pts',(6.534271137048,-2.563047905408,-2.020544571702));
#14878=CARTESIAN_POINT('Ctrl Pts',(6.693521137048,-1.248968678135,-3.015276776083));
#14879=CARTESIAN_POINT('Ctrl Pts',(6.852771137048,0.383608261101,-3.241089558554));
#14880=CARTESIAN_POINT('Ctrl Pts',(7.012021137048,1.918361836065,-2.640398557608));
#14881=CARTESIAN_POINT('Ctrl Pts',(7.171271137048,2.963917875123,-1.366384855545));
#14882=CARTESIAN_POINT('Ctrl Pts',(7.330521137048,3.253651172662,0.256067900963));
#14883=CARTESIAN_POINT('Ctrl Pts',(7.489771137048,2.713677441724,1.813221296591));
#14884=CARTESIAN_POINT('Ctrl Pts',(7.649021137048,1.481694291113,2.907988781792));
#14885=CARTESIAN_POINT('Ctrl Pts',(7.808271137048,-0.1281327360592,3.261195904774));
#14886=CARTESIAN_POINT('Ctrl Pts',(7.967521137048,-1.705284892359,2.782772028626));
#14887=CARTESIAN_POINT('Ctrl Pts',(8.126771137048,-2.84757578293,1.59471906236));
#14888=CARTESIAN_POINT('Ctrl Pts',(8.286021137048,-3.263712108535,0.));
#14889=CARTESIAN_POINT('Ctrl Pts',(8.445271137048,-2.84757578293,-1.59471906236));
#14890=CARTESIAN_POINT('Ctrl Pts',(8.604521137048,-1.705284892359,-2.782772028626));
#14891=CARTESIAN_POINT('Ctrl Pts',(8.763771137048,-0.1281327360592,-3.261195904774));
#14892=CARTESIAN_POINT('Ctrl Pts',(8.923021137048,1.481694291113,-2.907988781792));
#14893=CARTESIAN_POINT('Ctrl Pts',(9.082271137048,2.713677441724,-1.813221296591));
#14894=CARTESIAN_POINT('Ctrl Pts',(9.241521137048,3.253651172662,-0.256067900963));
#14895=CARTESIAN_POINT('Ctrl Pts',(9.400771137048,2.963917875123,1.366384855545));
#14896=CARTESIAN_POINT('Ctrl Pts',(9.560021137048,1.918361836065,2.640398557608));
#14897=CARTESIAN_POINT('Ctrl Pts',(9.719271137048,0.383608261101,3.241089558554));
#14898=CARTESIAN_POINT('Ctrl Pts',(9.878521137048,-1.248968678135,3.015276776083));
#14899=CARTESIAN_POINT('Ctrl Pts',(10.03777113705,-2.563047905408,2.020544571702));
#14900=CARTESIAN_POINT('Ctrl Pts',(10.19702113705,-3.223532154246,0.5105564866689));
#14901=CARTESIAN_POINT('Ctrl Pts',(10.35627113705,-3.061979863765,-1.129624298873));
#14902=CARTESIAN_POINT('Ctrl Pts',(10.51552113705,-2.119635939241,-2.481754111378));
#14903=CARTESIAN_POINT('Ctrl Pts',(10.67477113705,-0.6366272854614,-3.200971110614));
#14904=CARTESIAN_POINT('Ctrl Pts',(10.78093780372,0.4599252670358,-3.136380672689));
#14905=CARTESIAN_POINT('Ctrl Pts',(10.83402113705,0.9656781074217,-2.972051613422));
#14906=CARTESIAN_POINT('Ctrl Pts',(5.88,-3.21695909910602E-7,3.12449703095644));
#14907=CARTESIAN_POINT('Ctrl Pts',(5.895705128205,-0.157306535044492,3.12459764304402));
#14908=CARTESIAN_POINT('Ctrl Pts',(5.91141025641,-0.314639539052909,3.112929841749));
#14909=CARTESIAN_POINT('Ctrl Pts',(5.92711538461517,-0.470193579471061,
3.08937038670253));
#14910=CARTESIAN_POINT('Ctrl Pts',(5.93182698771779,-0.516860431844728,
3.08230245321972));
#14911=CARTESIAN_POINT('Ctrl Pts',(5.93653859082043,-0.563365438343652,
3.07416446995282));
#14912=CARTESIAN_POINT('Ctrl Pts',(5.94125019392308,-0.609657256300367,
3.06495400126008));
#14913=CARTESIAN_POINT('Ctrl Pts',(5.95224371902567,-0.717669381189642,
3.04346332885533));
#14914=CARTESIAN_POINT('Ctrl Pts',(5.9632372441283,-0.824520523417935,3.01613287001461));
#14915=CARTESIAN_POINT('Ctrl Pts',(5.97423076923084,-0.929617596829347,
2.98324879794399));
#14916=CARTESIAN_POINT('Ctrl Pts',(5.989935897436,-1.07975715593506,2.93627127590627));
#14917=CARTESIAN_POINT('Ctrl Pts',(6.00564102564099,-1.22632914373851,2.87796151164342));
#14918=CARTESIAN_POINT('Ctrl Pts',(6.02134615384615,-1.36775803719343,2.8091039241222));
#14919=CARTESIAN_POINT('Ctrl Pts',(6.03705128205133,-1.5091869306485,2.74024633660091));
#14920=CARTESIAN_POINT('Ctrl Pts',(6.05275641025667,-1.64548597437029,2.66083432711573));
#14921=CARTESIAN_POINT('Ctrl Pts',(6.06846153846185,-1.77506014945936,2.57161807835128));
#14922=CARTESIAN_POINT('Ctrl Pts',(6.07914097076807,-1.86317013579121,2.51095134091064));
#14923=CARTESIAN_POINT('Ctrl Pts',(6.08982040307421,-1.94817288076982,2.44574669164713));
#14924=CARTESIAN_POINT('Ctrl Pts',(6.10049983538033,-2.02952515103173,2.37626864249983));
#14925=CARTESIAN_POINT('Ctrl Pts',(6.10552553127922,-2.06780918704612,2.34357256496935));
#14926=CARTESIAN_POINT('Ctrl Pts',(6.1105512271781,-2.10528488988288,2.30993026036317));
#14927=CARTESIAN_POINT('Ctrl Pts',(6.11557692307699,-2.14191592065948,2.27539299236903));
#14928=CARTESIAN_POINT('Ctrl Pts',(6.13128205128199,-2.25638664196909,2.16746520831449));
#14929=CARTESIAN_POINT('Ctrl Pts',(6.14698717948701,-2.36259770943883,2.05080969082419));
#14930=CARTESIAN_POINT('Ctrl Pts',(6.16269230769218,-2.45953351178139,1.92692186650592));
#14931=CARTESIAN_POINT('Ctrl Pts',(6.17839743589734,-2.55646931412384,1.80303404218777));
#14932=CARTESIAN_POINT('Ctrl Pts',(6.19410256410266,-2.64414127751746,1.6719042538725));
#14933=CARTESIAN_POINT('Ctrl Pts',(6.20980769230782,-2.72154967470347,1.53495847225765));
#14934=CARTESIAN_POINT('Ctrl Pts',(6.22551282051299,-2.79895807188956,1.39801269064265));
#14935=CARTESIAN_POINT('Ctrl Pts',(6.24121794871801,-2.86610550760182,1.25523572060086));
#14936=CARTESIAN_POINT('Ctrl Pts',(6.25692307692301,-2.92192333127629,1.10813935100359));
#14937=CARTESIAN_POINT('Ctrl Pts',(6.25786539277047,-2.9252724296811,1.09931349244548));
#14938=CARTESIAN_POINT('Ctrl Pts',(6.25880770861792,-2.92858070337731,1.09047219858789));
#14939=CARTESIAN_POINT('Ctrl Pts',(6.25975002446537,-2.93184792475783,1.08161580336685));
#14940=CARTESIAN_POINT('Ctrl Pts',(6.27451283682291,-2.98303392179007,0.942866889013087));
#14941=CARTESIAN_POINT('Ctrl Pts',(6.28927564918046,-3.02414182613375,0.800411122418192));
#14942=CARTESIAN_POINT('Ctrl Pts',(6.30403846153816,-3.05502438429729,0.655798952752522));
#14943=CARTESIAN_POINT('Ctrl Pts',(6.31974358974334,-3.08787818772652,0.50195613408092));
#14944=CARTESIAN_POINT('Ctrl Pts',(6.33544871794871,-3.10916841598543,0.345660030799849));
#14945=CARTESIAN_POINT('Ctrl Pts',(6.3511538461539,-3.1187342224115,0.188648419769014));
#14946=CARTESIAN_POINT('Ctrl Pts',(6.36685897435902,-3.12830002883752,0.0316368087388328));
#14947=CARTESIAN_POINT('Ctrl Pts',(6.38256410256397,-3.12614026969898,-0.12610510103707));
#14948=CARTESIAN_POINT('Ctrl Pts',(6.39826923076908,-3.11205714799653,-0.282798238157188));
#14949=CARTESIAN_POINT('Ctrl Pts',(6.40517951072145,-3.10586055333675,-0.351743453374321));
#14950=CARTESIAN_POINT('Ctrl Pts',(6.41208979067384,-3.09735519217736,-0.420484489677447));
#14951=CARTESIAN_POINT('Ctrl Pts',(6.41900007062624,-3.0865260643595,-0.488857703250767));
#14952=CARTESIAN_POINT('Ctrl Pts',(6.42779491887912,-3.07274362189333,-0.575877627491321));
#14953=CARTESIAN_POINT('Ctrl Pts',(6.436589767132,-3.05519690668903,-0.66230164565767));
#14954=CARTESIAN_POINT('Ctrl Pts',(6.44538461538482,-3.0340200977109,-0.74781859016398));
#14955=CARTESIAN_POINT('Ctrl Pts',(6.46108974359,-2.99620426616755,-0.900527828411023));
#14956=CARTESIAN_POINT('Ctrl Pts',(6.476794871795,-2.94681582966476,-1.05034855944726));
#14957=CARTESIAN_POINT('Ctrl Pts',(6.4925,-2.88658577275698,-1.1956628320182));
#14958=CARTESIAN_POINT('Ctrl Pts',(6.508205128205,-2.82635571584919,-1.34097710458913));
#14959=CARTESIAN_POINT('Ctrl Pts',(6.52391025641,-2.75527937991822,-1.48179891776845));
#14960=CARTESIAN_POINT('Ctrl Pts',(6.53961538461517,-2.67404531641151,-1.61651716219695));
#14961=CARTESIAN_POINT('Ctrl Pts',(6.55249354986765,-2.60743359059155,-1.72698578057497));
#14962=CARTESIAN_POINT('Ctrl Pts',(6.56537171512024,-2.53398384454478,-1.83335602635669));
#14963=CARTESIAN_POINT('Ctrl Pts',(6.57824988037278,-2.45411540900217,-1.93466859159332));
#14964=CARTESIAN_POINT('Ctrl Pts',(6.58107684332547,-2.43658301180572,-1.9569083177461));
#14965=CARTESIAN_POINT('Ctrl Pts',(6.58390380627817,-2.41874138908149,-1.97890437133876));
#14966=CARTESIAN_POINT('Ctrl Pts',(6.58673076923086,-2.4005992967642,-2.00064999697506));
#14967=CARTESIAN_POINT('Ctrl Pts',(6.60243589743606,-2.29981131668746,-2.12145732421479));
#14968=CARTESIAN_POINT('Ctrl Pts',(6.61814102564111,-2.18976698077217,-2.23451450223418));
#14969=CARTESIAN_POINT('Ctrl Pts',(6.63384615384633,-2.07193616153301,-2.33873186210924));
#14970=CARTESIAN_POINT('Ctrl Pts',(6.64955128205139,-1.95410534229508,-2.44294922198321));
#14971=CARTESIAN_POINT('Ctrl Pts',(6.66525641025661,-1.82847988986133,-2.53833958057375));
#14972=CARTESIAN_POINT('Ctrl Pts',(6.68096153846167,-1.69644712969505,-2.62385329049029));
#14973=CARTESIAN_POINT('Ctrl Pts',(6.69666666666689,-1.56441436952739,-2.70936700040773));
#14974=CARTESIAN_POINT('Ctrl Pts',(6.71237179487195,-1.42595984987577,-2.78500861783667));
#14975=CARTESIAN_POINT('Ctrl Pts',(6.72807692307697,-1.28252819003516,-2.84966078036119));
#14976=CARTESIAN_POINT('Ctrl Pts',(6.73121799320022,-1.25384145182002,-2.86259139598291));
#14977=CARTESIAN_POINT('Ctrl Pts',(6.73435906332347,-1.22495656311743,-2.8750820037678));
#14978=CARTESIAN_POINT('Ctrl Pts',(6.73750013344671,-1.19588572614117,-2.887123539098));
#14979=CARTESIAN_POINT('Ctrl Pts',(6.75006419152849,-1.07960443666829,-2.93528882778825));
#14980=CARTESIAN_POINT('Ctrl Pts',(6.76262824961027,-0.960347655502351,
-2.97626761538678));
#14981=CARTESIAN_POINT('Ctrl Pts',(6.77519230769217,-0.83908019289306,-3.00992620370386));
#14982=CARTESIAN_POINT('Ctrl Pts',(6.79089743589734,-0.687495327956873,
-3.05199958805779));
#14983=CARTESIAN_POINT('Ctrl Pts',(6.80660256410267,-0.532757793114142,
-3.08264413157538));
#14984=CARTESIAN_POINT('Ctrl Pts',(6.82230769230783,-0.376606556598297,
-3.10163498008567));
#14985=CARTESIAN_POINT('Ctrl Pts',(6.838012820513,-0.220455320082452,-3.12062582859596));
#14986=CARTESIAN_POINT('Ctrl Pts',(6.853717948718,-0.0628756645481069,-3.12796387302098));
#14987=CARTESIAN_POINT('Ctrl Pts',(6.86942307692303,0.0943789619765832,
-3.12338542308761));
#14988=CARTESIAN_POINT('Ctrl Pts',(6.87853202085236,0.185586340671031,-3.12072993099726));
#14989=CARTESIAN_POINT('Ctrl Pts',(6.88764096478169,0.276685802602264,-3.11406434039434));
#14990=CARTESIAN_POINT('Ctrl Pts',(6.89674990871107,0.367304367055668,-3.1033389279845));
#14991=CARTESIAN_POINT('Ctrl Pts',(6.9033460929868,0.432925228768241,-3.09557218825737));
#14992=CARTESIAN_POINT('Ctrl Pts',(6.90994227726255,0.498293895125398,-3.08567670510919));
#14993=CARTESIAN_POINT('Ctrl Pts',(6.91653846153833,0.563276981103822,-3.07370359533634));
#14994=CARTESIAN_POINT('Ctrl Pts',(6.93224358974339,0.717997900620677,-3.04519632262622));
#14995=CARTESIAN_POINT('Ctrl Pts',(6.94794871794861,0.870526272338136,-3.00491480017493));
#14996=CARTESIAN_POINT('Ctrl Pts',(6.96365384615367,1.01920094228016,-2.95353305961266));
#14997=CARTESIAN_POINT('Ctrl Pts',(6.97935897435889,1.16787561222373,-2.90215131904986));
#14998=CARTESIAN_POINT('Ctrl Pts',(6.99506410256395,1.31271118268685,-2.83966664030563));
#14999=CARTESIAN_POINT('Ctrl Pts',(7.01076923076914,1.45207966320917,-2.76670577109897));
#15000=CARTESIAN_POINT('Ctrl Pts',(7.02584614949763,1.58587336592168,-2.69666335686228));
#15001=CARTESIAN_POINT('Ctrl Pts',(7.04092306822624,1.71463784791186,-2.61695511461419));
#15002=CARTESIAN_POINT('Ctrl Pts',(7.05599998695472,1.836828913414,-2.52817810742183));
#15003=CARTESIAN_POINT('Ctrl Pts',(7.05662819643142,1.84192024452083,-2.52447903878345));
#15004=CARTESIAN_POINT('Ctrl Pts',(7.05725640590813,1.8470001649315,-2.52076422913783));
#15005=CARTESIAN_POINT('Ctrl Pts',(7.05788461538484,1.85206859791098,-2.51703377008661));
#15006=CARTESIAN_POINT('Ctrl Pts',(7.07358974359,1.97877854529902,-2.42377293936711));
#15007=CARTESIAN_POINT('Ctrl Pts',(7.089294871795,2.09828043057227,-2.32075011669408));
#15008=CARTESIAN_POINT('Ctrl Pts',(7.105,2.20940661429584,-2.20940720229315));
#15009=CARTESIAN_POINT('Ctrl Pts',(7.120705128205,2.32053279801942,-2.09806428789222));
#15010=CARTESIAN_POINT('Ctrl Pts',(7.13641025641,2.42329735285879,-1.97839483543744));
#15011=CARTESIAN_POINT('Ctrl Pts',(7.15211538461517,2.51660034679189,-1.85174928324409));
#15012=CARTESIAN_POINT('Ctrl Pts',(7.16782051282033,2.60990334072498,-1.72510373105075));
#15013=CARTESIAN_POINT('Ctrl Pts',(7.18352564102567,2.69375117108915,-1.59146857523107));
#15014=CARTESIAN_POINT('Ctrl Pts',(7.19923076923086,2.76698261297629,-1.45222443021403));
#15015=CARTESIAN_POINT('Ctrl Pts',(7.20457056320872,2.79188153817257,-1.40488097415942));
#15016=CARTESIAN_POINT('Ctrl Pts',(7.20991035718657,2.81555228674541,-1.35689047491985));
#15017=CARTESIAN_POINT('Ctrl Pts',(7.21525015116441,2.83794741820317,-1.30831167980417));
#15018=CARTESIAN_POINT('Ctrl Pts',(7.2256154853917,2.88141969889172,-1.21401301400872));
#15019=CARTESIAN_POINT('Ctrl Pts',(7.23598081961898,2.9200846630212,-1.11749740512213));
#15020=CARTESIAN_POINT('Ctrl Pts',(7.24634615384633,2.95384328122046,-1.01930854475145));
#15021=CARTESIAN_POINT('Ctrl Pts',(7.26205128205139,3.00499295138218,-0.870536820983832));
#15022=CARTESIAN_POINT('Ctrl Pts',(7.27775641025661,3.04488646955175,-0.717917299307448));
#15023=CARTESIAN_POINT('Ctrl Pts',(7.29346153846167,3.07323267657502,-0.563190821606695));
#15024=CARTESIAN_POINT('Ctrl Pts',(7.30916666666689,3.10157888359859,-0.408464343904331));
#15025=CARTESIAN_POINT('Ctrl Pts',(7.32487179487195,3.11838067165169,-0.251616473021808));
#15026=CARTESIAN_POINT('Ctrl Pts',(7.34057692307697,3.12331108802163,-0.0943762077870904));
#15027=CARTESIAN_POINT('Ctrl Pts',(7.35188456103662,3.12686097074617,0.018836239048195));
#15028=CARTESIAN_POINT('Ctrl Pts',(7.36319219899625,3.12425420322951,0.132257831845049));
#15029=CARTESIAN_POINT('Ctrl Pts',(7.37449983695594,3.11536666791583,0.245184674149663));
#15030=CARTESIAN_POINT('Ctrl Pts',(7.37889732720134,3.11191034485466,0.289101422213974));
#15031=CARTESIAN_POINT('Ctrl Pts',(7.38329481744675,3.10750429091715,0.332943335439869));
#15032=CARTESIAN_POINT('Ctrl Pts',(7.38769230769217,3.10216193300488,0.37667061407462));
#15033=CARTESIAN_POINT('Ctrl Pts',(7.40339743589733,3.08308231912341,0.532837536272352));
#15034=CARTESIAN_POINT('Ctrl Pts',(7.41910256410267,3.05206338319806,0.687523279012142));
#15035=CARTESIAN_POINT('Ctrl Pts',(7.43480769230783,3.0097189125242,0.839021679403842));
#15036=CARTESIAN_POINT('Ctrl Pts',(7.450512820513,2.96737444185033,0.990520079795541));
#15037=CARTESIAN_POINT('Ctrl Pts',(7.466217948718,2.91370372918221,1.13884614555346));
#15038=CARTESIAN_POINT('Ctrl Pts',(7.48192307692303,2.84927329204631,1.28235426733883));
#15039=CARTESIAN_POINT('Ctrl Pts',(7.49762820512805,2.78484285491041,1.42586238912421));
#15040=CARTESIAN_POINT('Ctrl Pts',(7.51333333333311,2.70964227733817,1.56456383704047));
#15041=CARTESIAN_POINT('Ctrl Pts',(7.52903846153833,2.62426134529928,1.69671142476984));
#15042=CARTESIAN_POINT('Ctrl Pts',(7.5306089923509,2.61572315428164,1.70992633493315));
#15043=CARTESIAN_POINT('Ctrl Pts',(7.53217952316347,2.60708334093589,1.72307544280506));
#15044=CARTESIAN_POINT('Ctrl Pts',(7.53375005397604,2.59834253844517,1.7361569781865));
#15045=CARTESIAN_POINT('Ctrl Pts',(7.54788465136856,2.5196763173783,1.85388929799372));
#15046=CARTESIAN_POINT('Ctrl Pts',(7.56201924876118,2.4328286128156,1.96614691665661));
#15047=CARTESIAN_POINT('Ctrl Pts',(7.57615384615367,2.33882800562177,2.07202028766332));
#15048=CARTESIAN_POINT('Ctrl Pts',(7.59185897435889,2.23438275356725,2.18965751630222));
#15049=CARTESIAN_POINT('Ctrl Pts',(7.60756410256395,2.12110179310409,2.29942752308062));
#15050=CARTESIAN_POINT('Ctrl Pts',(7.62326923076914,2.00029920318409,2.40017868230316));
#15051=CARTESIAN_POINT('Ctrl Pts',(7.63897435897433,1.87949661326408,2.5009298415257));
#15052=CARTESIAN_POINT('Ctrl Pts',(7.65467948717967,1.75116000914845,2.59267025933498));
#15053=CARTESIAN_POINT('Ctrl Pts',(7.67038461538483,1.61660883785066,2.674197927153));
#15054=CARTESIAN_POINT('Ctrl Pts',(7.67792308497015,1.55202420668778,2.71333124947796));
#15055=CARTESIAN_POINT('Ctrl Pts',(7.68546155455542,1.48600787178097,2.75011066378684));
#15056=CARTESIAN_POINT('Ctrl Pts',(7.69300002414067,1.41872031168613,2.78439538808883));
#15057=CARTESIAN_POINT('Ctrl Pts',(7.70116668276046,1.34582560455246,2.82153709650612));
#15058=CARTESIAN_POINT('Ctrl Pts',(7.70933334138023,1.27143900290213,2.85575093945237));
#15059=CARTESIAN_POINT('Ctrl Pts',(7.7175,1.19582529175154,2.88697719853058));
#15060=CARTESIAN_POINT('Ctrl Pts',(7.733205128205,1.05041416549221,2.94702775592731));
#15061=CARTESIAN_POINT('Ctrl Pts',(7.74891025641,0.900465813463126,2.99603287482205));
#15062=CARTESIAN_POINT('Ctrl Pts',(7.76461538461517,0.747723396432291,3.03363235324925));
#15063=CARTESIAN_POINT('Ctrl Pts',(7.78032051282033,0.594980979401457,3.07123183167645));
#15064=CARTESIAN_POINT('Ctrl Pts',(7.79602564102567,0.439430544027183,3.09743052627249));
#15065=CARTESIAN_POINT('Ctrl Pts',(7.81173076923086,0.282778041871423,3.11184033086417));
#15066=CARTESIAN_POINT('Ctrl Pts',(7.82523715029811,0.148057181168531,3.12423273603125));
#15067=CARTESIAN_POINT('Ctrl Pts',(7.83874353136525,0.0125106239082456,
3.12790266438722));
#15068=CARTESIAN_POINT('Ctrl Pts',(7.85224991243248,-0.122686924247132,
3.12259073825233));
#15069=CARTESIAN_POINT('Ctrl Pts',(7.85444865957043,-0.144696167180856,
3.1217259927422));
#15070=CARTESIAN_POINT('Ctrl Pts',(7.85664740670837,-0.166696155154839,
3.12062326574181));
#15071=CARTESIAN_POINT('Ctrl Pts',(7.85884615384633,-0.1886819155548,3.11928401449904));
#15072=CARTESIAN_POINT('Ctrl Pts',(7.87455128205139,-0.345720976484957,
3.10971806118707));
#15073=CARTESIAN_POINT('Ctrl Pts',(7.89025641025661,-0.502004351790296,
3.08808590041721));
#15074=CARTESIAN_POINT('Ctrl Pts',(7.90596153846167,-0.655779338422631,
3.05493687313145));
#15075=CARTESIAN_POINT('Ctrl Pts',(7.92166666666689,-0.809554325056565,
3.02178784584535));
#15076=CARTESIAN_POINT('Ctrl Pts',(7.93737179487195,-0.960836126315138,
2.9771233215876));
#15077=CARTESIAN_POINT('Ctrl Pts',(7.95307692307697,-1.10796040920211,2.9214504428197));
#15078=CARTESIAN_POINT('Ctrl Pts',(7.968782051282,-1.25508469208908,2.86577756405179));
#15079=CARTESIAN_POINT('Ctrl Pts',(7.984487179487,-1.39806382918831,2.79908769904581));
#15080=CARTESIAN_POINT('Ctrl Pts',(8.00019230769217,-1.53515081641421,2.72188982514671));
#15081=CARTESIAN_POINT('Ctrl Pts',(8.00396158983553,-1.56805214178305,2.70336208288368));
#15082=CARTESIAN_POINT('Ctrl Pts',(8.00773087197889,-1.60061292833792,2.68422968792613));
#15083=CARTESIAN_POINT('Ctrl Pts',(8.01150015412227,-1.63280801473754,2.66450051360633));
#15084=CARTESIAN_POINT('Ctrl Pts',(8.02343600018412,-1.73475729329959,2.60202591535358));
#15085=CARTESIAN_POINT('Ctrl Pts',(8.03537184624603,-1.8330386668105,2.53356607404464));
#15086=CARTESIAN_POINT('Ctrl Pts',(8.04730769230783,-1.92707055798493,2.45972435726965));
#15087=CARTESIAN_POINT('Ctrl Pts',(8.063012820513,-2.05079726312352,2.36256378542284));
#15088=CARTESIAN_POINT('Ctrl Pts',(8.078717948718,-2.16717972241397,2.25608242363812));
#15089=CARTESIAN_POINT('Ctrl Pts',(8.09442307692303,-2.27501273852753,2.14155794469054));
#15090=CARTESIAN_POINT('Ctrl Pts',(8.11012820512806,-2.3828457546411,2.02703346574295));
#15091=CARTESIAN_POINT('Ctrl Pts',(8.12583333333311,-2.48213900530219,1.90445476333191));
#15092=CARTESIAN_POINT('Ctrl Pts',(8.14153846153833,-2.57165193077396,1.77508287620843));
#15093=CARTESIAN_POINT('Ctrl Pts',(8.15127559877096,-2.62714970373215,1.69487265426663));
#15094=CARTESIAN_POINT('Ctrl Pts',(8.16101273600365,-2.67888797642152,1.61204808608716));
#15095=CARTESIAN_POINT('Ctrl Pts',(8.17074987323633,-2.72655002210233,1.52694137967767));
#15096=CARTESIAN_POINT('Ctrl Pts',(8.17671786420879,-2.75576257724611,1.47477860910038));
#15097=CARTESIAN_POINT('Ctrl Pts',(8.18268585518124,-2.78344401079767,1.42175865550711));
#15098=CARTESIAN_POINT('Ctrl Pts',(8.18865384615367,-2.80956688241491,1.36798352909411));
#15099=CARTESIAN_POINT('Ctrl Pts',(8.20435897435889,-2.87831079468499,1.22647104047447));
#15100=CARTESIAN_POINT('Ctrl Pts',(8.22006410256395,-2.9362584893282,1.07973927060473));
#15101=CARTESIAN_POINT('Ctrl Pts',(8.23576923076914,-2.982977349702,0.929533639746724));
#15102=CARTESIAN_POINT('Ctrl Pts',(8.25147435897433,-3.0296962100758,0.779328008888721));
#15103=CARTESIAN_POINT('Ctrl Pts',(8.26717948717967,-3.06519301000169,0.625635251226046));
#15104=CARTESIAN_POINT('Ctrl Pts',(8.28288461538483,-3.08901983228559,0.470139769698067));
#15105=CARTESIAN_POINT('Ctrl Pts',(8.29858974359,-3.11284665456948,0.314644288170088));
#15106=CARTESIAN_POINT('Ctrl Pts',(8.314294871795,-3.125,0.157330906751383));
#15107=CARTESIAN_POINT('Ctrl Pts',(8.33,-3.125,0.));
#15108=CARTESIAN_POINT('Ctrl Pts',(8.345705128205,-3.125,-0.157330906751383));
#15109=CARTESIAN_POINT('Ctrl Pts',(8.36141025641,-3.11284665456948,-0.314644288170091));
#15110=CARTESIAN_POINT('Ctrl Pts',(8.37711538461517,-3.08901983228559,-0.47013976969807));
#15111=CARTESIAN_POINT('Ctrl Pts',(8.39282051282033,-3.06519301000169,-0.625635251226049));
#15112=CARTESIAN_POINT('Ctrl Pts',(8.40852564102567,-3.0296962100758,-0.779328008888722));
#15113=CARTESIAN_POINT('Ctrl Pts',(8.42423076923086,-2.982977349702,-0.929533639746725));
#15114=CARTESIAN_POINT('Ctrl Pts',(8.43993589743605,-2.9362584893282,-1.07973927060473));
#15115=CARTESIAN_POINT('Ctrl Pts',(8.45564102564111,-2.87831079468499,-1.22647104047447));
#15116=CARTESIAN_POINT('Ctrl Pts',(8.47134615384633,-2.80956688241491,-1.36798352909411));
#15117=CARTESIAN_POINT('Ctrl Pts',(8.47731414481876,-2.78344401079767,-1.42175865550711));
#15118=CARTESIAN_POINT('Ctrl Pts',(8.48328213579122,-2.75576257724611,-1.47477860910038));
#15119=CARTESIAN_POINT('Ctrl Pts',(8.48925012676368,-2.72655002210233,-1.52694137967767));
#15120=CARTESIAN_POINT('Ctrl Pts',(8.49898726399635,-2.67888797642152,-1.61204808608716));
#15121=CARTESIAN_POINT('Ctrl Pts',(8.50872440122904,-2.62714970373215,-1.69487265426663));
#15122=CARTESIAN_POINT('Ctrl Pts',(8.51846153846167,-2.57165193077395,-1.77508287620844));
#15123=CARTESIAN_POINT('Ctrl Pts',(8.53416666666689,-2.48213900530219,-1.90445476333191));
#15124=CARTESIAN_POINT('Ctrl Pts',(8.54987179487195,-2.3828457546411,-2.02703346574295));
#15125=CARTESIAN_POINT('Ctrl Pts',(8.56557692307697,-2.27501273852753,-2.14155794469054));
#15126=CARTESIAN_POINT('Ctrl Pts',(8.581282051282,-2.16717972241396,-2.25608242363812));
#15127=CARTESIAN_POINT('Ctrl Pts',(8.596987179487,-2.05079726312352,-2.36256378542284));
#15128=CARTESIAN_POINT('Ctrl Pts',(8.61269230769217,-1.92707055798493,-2.45972435726965));
#15129=CARTESIAN_POINT('Ctrl Pts',(8.62462815375398,-1.8330386668105,-2.53356607404464));
#15130=CARTESIAN_POINT('Ctrl Pts',(8.63656399981588,-1.73475729329959,-2.60202591535358));
#15131=CARTESIAN_POINT('Ctrl Pts',(8.64849984587773,-1.63280801473754,-2.66450051360633));
#15132=CARTESIAN_POINT('Ctrl Pts',(8.65226912802111,-1.60061292833792,-2.68422968792613));
#15133=CARTESIAN_POINT('Ctrl Pts',(8.65603841016448,-1.56805214178305,-2.70336208288368));
#15134=CARTESIAN_POINT('Ctrl Pts',(8.65980769230783,-1.53515081641421,-2.72188982514671));
#15135=CARTESIAN_POINT('Ctrl Pts',(8.675512820513,-1.39806382918831,-2.79908769904581));
#15136=CARTESIAN_POINT('Ctrl Pts',(8.691217948718,-1.25508469208908,-2.86577756405179));
#15137=CARTESIAN_POINT('Ctrl Pts',(8.70692307692303,-1.10796040920211,-2.92145044281969));
#15138=CARTESIAN_POINT('Ctrl Pts',(8.72262820512806,-0.960836126315141,
-2.9771233215876));
#15139=CARTESIAN_POINT('Ctrl Pts',(8.73833333333311,-0.809554325056562,
-3.02178784584535));
#15140=CARTESIAN_POINT('Ctrl Pts',(8.75403846153833,-0.655779338422628,
-3.05493687313145));
#15141=CARTESIAN_POINT('Ctrl Pts',(8.76974358974339,-0.502004351790293,
-3.08808590041721));
#15142=CARTESIAN_POINT('Ctrl Pts',(8.78544871794861,-0.345720976484962,
-3.10971806118707));
#15143=CARTESIAN_POINT('Ctrl Pts',(8.80115384615367,-0.188681915554805,
-3.11928401449904));
#15144=CARTESIAN_POINT('Ctrl Pts',(8.80335259329162,-0.166696155154845,
-3.12062326574181));
#15145=CARTESIAN_POINT('Ctrl Pts',(8.80555134042957,-0.144696167180862,
-3.1217259927422));
#15146=CARTESIAN_POINT('Ctrl Pts',(8.80775008756752,-0.122686924247137,
-3.12259073825233));
#15147=CARTESIAN_POINT('Ctrl Pts',(8.82125646863476,0.0125106239082456,
-3.12790266438722));
#15148=CARTESIAN_POINT('Ctrl Pts',(8.83476284970189,0.148057181168534,-3.12423273603126));
#15149=CARTESIAN_POINT('Ctrl Pts',(8.84826923076914,0.282778041871425,-3.11184033086417));
#15150=CARTESIAN_POINT('Ctrl Pts',(8.86397435897433,0.439430544027182,-3.09743052627249));
#15151=CARTESIAN_POINT('Ctrl Pts',(8.87967948717967,0.594980979401456,-3.07123183167645));
#15152=CARTESIAN_POINT('Ctrl Pts',(8.89538461538483,0.747723396432294,-3.03363235324925));
#15153=CARTESIAN_POINT('Ctrl Pts',(8.91108974359,0.900465813463131,-2.99603287482204));
#15154=CARTESIAN_POINT('Ctrl Pts',(8.926794871795,1.05041416549222,-2.94702775592731));
#15155=CARTESIAN_POINT('Ctrl Pts',(8.9425,1.19582529175154,-2.88697719853058));
#15156=CARTESIAN_POINT('Ctrl Pts',(8.95066665861977,1.27143900290213,-2.85575093945237));
#15157=CARTESIAN_POINT('Ctrl Pts',(8.95883331723954,1.34582560455246,-2.82153709650612));
#15158=CARTESIAN_POINT('Ctrl Pts',(8.96699997585933,1.41872031168613,-2.78439538808883));
#15159=CARTESIAN_POINT('Ctrl Pts',(8.97453844544458,1.48600787178097,-2.75011066378684));
#15160=CARTESIAN_POINT('Ctrl Pts',(8.98207691502986,1.55202420668778,-2.71333124947796));
#15161=CARTESIAN_POINT('Ctrl Pts',(8.98961538461517,1.61660883785066,-2.674197927153));
#15162=CARTESIAN_POINT('Ctrl Pts',(9.00532051282033,1.75116000914844,-2.59267025933498));
#15163=CARTESIAN_POINT('Ctrl Pts',(9.02102564102567,1.87949661326408,-2.5009298415257));
#15164=CARTESIAN_POINT('Ctrl Pts',(9.03673076923086,2.00029920318409,-2.40017868230316));
#15165=CARTESIAN_POINT('Ctrl Pts',(9.05243589743606,2.12110179310409,-2.29942752308062));
#15166=CARTESIAN_POINT('Ctrl Pts',(9.06814102564111,2.23438275356726,-2.18965751630222));
#15167=CARTESIAN_POINT('Ctrl Pts',(9.08384615384633,2.33882800562177,-2.07202028766331));
#15168=CARTESIAN_POINT('Ctrl Pts',(9.09798075123882,2.4328286128156,-1.9661469166566));
#15169=CARTESIAN_POINT('Ctrl Pts',(9.11211534863145,2.5196763173783,-1.85388929799372));
#15170=CARTESIAN_POINT('Ctrl Pts',(9.12624994602396,2.59834253844517,-1.7361569781865));
#15171=CARTESIAN_POINT('Ctrl Pts',(9.12782047683653,2.60708334093589,-1.72307544280507));
#15172=CARTESIAN_POINT('Ctrl Pts',(9.1293910076491,2.61572315428164,-1.70992633493316));
#15173=CARTESIAN_POINT('Ctrl Pts',(9.13096153846167,2.62426134529928,-1.69671142476984));
#15174=CARTESIAN_POINT('Ctrl Pts',(9.14666666666689,2.70964227733817,-1.56456383704048));
#15175=CARTESIAN_POINT('Ctrl Pts',(9.16237179487195,2.78484285491041,-1.42586238912421));
#15176=CARTESIAN_POINT('Ctrl Pts',(9.17807692307697,2.84927329204631,-1.28235426733883));
#15177=CARTESIAN_POINT('Ctrl Pts',(9.193782051282,2.91370372918221,-1.13884614555346));
#15178=CARTESIAN_POINT('Ctrl Pts',(9.209487179487,2.96737444185033,-0.990520079795544));
#15179=CARTESIAN_POINT('Ctrl Pts',(9.22519230769217,3.0097189125242,-0.839021679403841));
#15180=CARTESIAN_POINT('Ctrl Pts',(9.24089743589733,3.05206338319806,-0.687523279012144));
#15181=CARTESIAN_POINT('Ctrl Pts',(9.25660256410267,3.08308231912341,-0.532837536272352));
#15182=CARTESIAN_POINT('Ctrl Pts',(9.27230769230784,3.10216193300488,-0.376670614074617));
#15183=CARTESIAN_POINT('Ctrl Pts',(9.27670518255326,3.10750429091715,-0.332943335439869));
#15184=CARTESIAN_POINT('Ctrl Pts',(9.28110267279866,3.11191034485466,-0.289101422213986));
#15185=CARTESIAN_POINT('Ctrl Pts',(9.28550016304406,3.11536666791583,-0.245184674149674));
#15186=CARTESIAN_POINT('Ctrl Pts',(9.29680780100375,3.12425420322951,-0.132257831845052));
#15187=CARTESIAN_POINT('Ctrl Pts',(9.30811543896338,3.12686097074617,-0.0188362390481956));
#15188=CARTESIAN_POINT('Ctrl Pts',(9.31942307692303,3.12331108802163,0.0943762077871013));
#15189=CARTESIAN_POINT('Ctrl Pts',(9.33512820512805,3.11838067165169,0.251616473021838));
#15190=CARTESIAN_POINT('Ctrl Pts',(9.35083333333311,3.10157888359858,0.408464343904398));
#15191=CARTESIAN_POINT('Ctrl Pts',(9.36653846153833,3.07323267657501,0.563190821606759));
#15192=CARTESIAN_POINT('Ctrl Pts',(9.38224358974339,3.04488646955173,0.717917299307511));
#15193=CARTESIAN_POINT('Ctrl Pts',(9.39794871794861,3.00499295138217,0.87053682098386));
#15194=CARTESIAN_POINT('Ctrl Pts',(9.41365384615367,2.95384328122045,1.01930854475146));
#15195=CARTESIAN_POINT('Ctrl Pts',(9.42401918038102,2.9200846630212,1.11749740512214));
#15196=CARTESIAN_POINT('Ctrl Pts',(9.4343845146083,2.88141969889172,1.21401301400872));
#15197=CARTESIAN_POINT('Ctrl Pts',(9.44474984883559,2.83794741820317,1.30831167980417));
#15198=CARTESIAN_POINT('Ctrl Pts',(9.45008964281343,2.8155522867454,1.35689047491985));
#15199=CARTESIAN_POINT('Ctrl Pts',(9.45542943679128,2.79188153817257,1.40488097415943));
#15200=CARTESIAN_POINT('Ctrl Pts',(9.46076923076914,2.76698261297628,1.45222443021404));
#15201=CARTESIAN_POINT('Ctrl Pts',(9.47647435897433,2.69375117108915,1.59146857523107));
#15202=CARTESIAN_POINT('Ctrl Pts',(9.49217948717967,2.60990334072498,1.72510373105075));
#15203=CARTESIAN_POINT('Ctrl Pts',(9.50788461538483,2.51660034679189,1.8517492832441));
#15204=CARTESIAN_POINT('Ctrl Pts',(9.52358974359,2.42329735285879,1.97839483543744));
#15205=CARTESIAN_POINT('Ctrl Pts',(9.539294871795,2.32053279801942,2.09806428789222));
#15206=CARTESIAN_POINT('Ctrl Pts',(9.555,2.20940661429584,2.20940720229315));
#15207=CARTESIAN_POINT('Ctrl Pts',(9.570705128205,2.09828043057227,2.32075011669408));
#15208=CARTESIAN_POINT('Ctrl Pts',(9.58641025641,1.97877854529902,2.42377293936711));
#15209=CARTESIAN_POINT('Ctrl Pts',(9.60211538461517,1.85206859791098,2.51703377008662));
#15210=CARTESIAN_POINT('Ctrl Pts',(9.60274359409187,1.84700016493149,2.52076422913783));
#15211=CARTESIAN_POINT('Ctrl Pts',(9.60337180356858,1.84192024452082,2.52447903878346));
#15212=CARTESIAN_POINT('Ctrl Pts',(9.60400001304529,1.83682891341399,2.52817810742184));
#15213=CARTESIAN_POINT('Ctrl Pts',(9.61907693177376,1.71463784791186,2.61695511461419));
#15214=CARTESIAN_POINT('Ctrl Pts',(9.63415385050238,1.58587336592168,2.69666335686228));
#15215=CARTESIAN_POINT('Ctrl Pts',(9.64923076923086,1.45207966320917,2.76670577109897));
#15216=CARTESIAN_POINT('Ctrl Pts',(9.66493589743606,1.31271118268685,2.83966664030563));
#15217=CARTESIAN_POINT('Ctrl Pts',(9.68064102564111,1.16787561222373,2.90215131904986));
#15218=CARTESIAN_POINT('Ctrl Pts',(9.69634615384633,1.01920094228016,2.95353305961267));
#15219=CARTESIAN_POINT('Ctrl Pts',(9.71205128205139,0.870526272338138,3.00491480017493));
#15220=CARTESIAN_POINT('Ctrl Pts',(9.72775641025661,0.717997900620678,3.04519632262622));
#15221=CARTESIAN_POINT('Ctrl Pts',(9.74346153846167,0.563276981103821,3.07370359533634));
#15222=CARTESIAN_POINT('Ctrl Pts',(9.75005772273745,0.498293895125397,3.08567670510919));
#15223=CARTESIAN_POINT('Ctrl Pts',(9.7566539070132,0.432925228768243,3.09557218825737));
#15224=CARTESIAN_POINT('Ctrl Pts',(9.76325009128893,0.367304367055667,3.1033389279845));
#15225=CARTESIAN_POINT('Ctrl Pts',(9.77235903521831,0.276685802602259,3.11406434039434));
#15226=CARTESIAN_POINT('Ctrl Pts',(9.78146797914765,0.185586340671027,3.12072993099726));
#15227=CARTESIAN_POINT('Ctrl Pts',(9.79057692307697,0.0943789619765783,
3.12338542308761));
#15228=CARTESIAN_POINT('Ctrl Pts',(9.806282051282,-0.0628756645481118,3.12796387302098));
#15229=CARTESIAN_POINT('Ctrl Pts',(9.821987179487,-0.220455320082457,3.12062582859596));
#15230=CARTESIAN_POINT('Ctrl Pts',(9.83769230769217,-0.376606556598298,
3.10163498008567));
#15231=CARTESIAN_POINT('Ctrl Pts',(9.85339743589733,-0.53275779311414,3.08264413157538));
#15232=CARTESIAN_POINT('Ctrl Pts',(9.86910256410266,-0.687495327956871,
3.0519995880578));
#15233=CARTESIAN_POINT('Ctrl Pts',(9.88480769230783,-0.839080192893056,
3.00992620370386));
#15234=CARTESIAN_POINT('Ctrl Pts',(9.89737175038972,-0.960347655502346,
2.97626761538679));
#15235=CARTESIAN_POINT('Ctrl Pts',(9.90993580847151,-1.07960443666828,2.93528882778825));
#15236=CARTESIAN_POINT('Ctrl Pts',(9.92249986655329,-1.19588572614116,2.887123539098));
#15237=CARTESIAN_POINT('Ctrl Pts',(9.92564093667654,-1.22495656311742,2.8750820037678));
#15238=CARTESIAN_POINT('Ctrl Pts',(9.92878200679978,-1.25384145182002,2.86259139598291));
#15239=CARTESIAN_POINT('Ctrl Pts',(9.93192307692303,-1.28252819003516,2.84966078036119));
#15240=CARTESIAN_POINT('Ctrl Pts',(9.94762820512806,-1.42595984987577,2.78500861783667));
#15241=CARTESIAN_POINT('Ctrl Pts',(9.96333333333311,-1.56441436952739,2.70936700040773));
#15242=CARTESIAN_POINT('Ctrl Pts',(9.97903846153766,-1.69644712969505,2.62385329049029));
#15243=CARTESIAN_POINT('Ctrl Pts',(9.99474358974206,-1.82847988986133,2.53833958057375));
#15244=CARTESIAN_POINT('Ctrl Pts',(10.0104487179459,-1.95410534229508,2.44294922198321));
#15245=CARTESIAN_POINT('Ctrl Pts',(10.0261538461512,-2.07193616153301,2.33873186210924));
#15246=CARTESIAN_POINT('Ctrl Pts',(10.0418589743566,-2.18976698077217,2.23451450223419));
#15247=CARTESIAN_POINT('Ctrl Pts',(10.0575641025633,-2.29981131668746,2.12145732421479));
#15248=CARTESIAN_POINT('Ctrl Pts',(10.0732692307683,-2.40059929676421,2.00064999697506));
#15249=CARTESIAN_POINT('Ctrl Pts',(10.076096193721,-2.4187413890815,1.97890437133876));
#15250=CARTESIAN_POINT('Ctrl Pts',(10.0789231566736,-2.43658301180573,1.9569083177461));
#15251=CARTESIAN_POINT('Ctrl Pts',(10.0817501196261,-2.45411540900217,1.93466859159331));
#15252=CARTESIAN_POINT('Ctrl Pts',(10.0946282848781,-2.53398384454479,1.83335602635669));
#15253=CARTESIAN_POINT('Ctrl Pts',(10.1075064501293,-2.60743359059154,1.72698578057498));
#15254=CARTESIAN_POINT('Ctrl Pts',(10.1203846153817,-2.67404531641151,1.61651716219696));
#15255=CARTESIAN_POINT('Ctrl Pts',(10.1360897435867,-2.75527937991822,1.48179891776845));
#15256=CARTESIAN_POINT('Ctrl Pts',(10.1517948717933,-2.82635571584919,1.34097710458913));
#15257=CARTESIAN_POINT('Ctrl Pts',(10.1675,-2.88658577275698,1.1956628320182));
#15258=CARTESIAN_POINT('Ctrl Pts',(10.1832051282067,-2.94681582966476,1.05034855944727));
#15259=CARTESIAN_POINT('Ctrl Pts',(10.1989102564133,-2.99620426616754,0.900527828411019));
#15260=CARTESIAN_POINT('Ctrl Pts',(10.2146153846183,-3.03402009771087,0.747818590164109));
#15261=CARTESIAN_POINT('Ctrl Pts',(10.2234102328711,-3.05519690668902,0.662301645657736));
#15262=CARTESIAN_POINT('Ctrl Pts',(10.2322050811233,-3.07274362189332,0.575877627491373));
#15263=CARTESIAN_POINT('Ctrl Pts',(10.2409999293756,-3.0865260643595,0.488857703250772));
#15264=CARTESIAN_POINT('Ctrl Pts',(10.2479102093275,-3.09735519217732,0.420484489677666));
#15265=CARTESIAN_POINT('Ctrl Pts',(10.2548204892794,-3.10586055333669,0.351743453374736));
#15266=CARTESIAN_POINT('Ctrl Pts',(10.2617307692317,-3.11205714799648,0.282798238157759));
#15267=CARTESIAN_POINT('Ctrl Pts',(10.2774358974367,-3.12614026969902,0.126105101036856));
#15268=CARTESIAN_POINT('Ctrl Pts',(10.2931410256434,-3.12830002883756,-0.0316368087400947));
#15269=CARTESIAN_POINT('Ctrl Pts',(10.3088461538485,-3.11873422241136,-0.188648419771246));
#15270=CARTESIAN_POINT('Ctrl Pts',(10.3245512820534,-3.10916841598527,-0.345660030800766));
#15271=CARTESIAN_POINT('Ctrl Pts',(10.3402564102566,-3.08787818772652,-0.50195613408048));
#15272=CARTESIAN_POINT('Ctrl Pts',(10.3559615384615,-3.05502438429765,-0.65579895275087));
#15273=CARTESIAN_POINT('Ctrl Pts',(10.3707243508191,-3.02414182613406,-0.800411122417126));
#15274=CARTESIAN_POINT('Ctrl Pts',(10.3854871631782,-2.98303392179023,-0.942866889012677));
#15275=CARTESIAN_POINT('Ctrl Pts',(10.4002499755359,-2.93184792475783,-1.08161580336685));
#15276=CARTESIAN_POINT('Ctrl Pts',(10.4011922913834,-2.92858070337733,-1.09047219858785));
#15277=CARTESIAN_POINT('Ctrl Pts',(10.4021346072309,-2.92527242968113,-1.0993134924454));
#15278=CARTESIAN_POINT('Ctrl Pts',(10.4030769230783,-2.92192333127634,-1.10813935100346));
#15279=CARTESIAN_POINT('Ctrl Pts',(10.4187820512833,-2.8661055076018,-1.25523572060092));
#15280=CARTESIAN_POINT('Ctrl Pts',(10.4344871794867,-2.79895807188958,-1.3980126906426));
#15281=CARTESIAN_POINT('Ctrl Pts',(10.4501923076917,-2.72154967470354,-1.53495847225753));
#15282=CARTESIAN_POINT('Ctrl Pts',(10.4658974358967,-2.6441412775175,-1.67190425387246));
#15283=CARTESIAN_POINT('Ctrl Pts',(10.4816025641033,-2.55646931412381,-1.80303404218782));
#15284=CARTESIAN_POINT('Ctrl Pts',(10.4973076923083,-2.45953351178131,-1.92692186650602));
#15285=CARTESIAN_POINT('Ctrl Pts',(10.5130128205133,-2.3625977094388,-2.05080969082422));
#15286=CARTESIAN_POINT('Ctrl Pts',(10.5287179487167,-2.25638664196914,-2.16746520831446));
#15287=CARTESIAN_POINT('Ctrl Pts',(10.5444230769217,-2.14191592065938,-2.27539299236912));
#15288=CARTESIAN_POINT('Ctrl Pts',(10.5494487728206,-2.10528488988284,-2.30993026036321));
#15289=CARTESIAN_POINT('Ctrl Pts',(10.5544744687196,-2.0678091870461,-2.34357256496936));
#15290=CARTESIAN_POINT('Ctrl Pts',(10.5595001646187,-2.02952515103173,-2.37626864249984));
#15291=CARTESIAN_POINT('Ctrl Pts',(10.5701795969254,-1.94817288076942,-2.44574669164748));
#15292=CARTESIAN_POINT('Ctrl Pts',(10.5808590292323,-1.86317013579029,-2.51095134091135));
#15293=CARTESIAN_POINT('Ctrl Pts',(10.5915384615385,-1.7750601494579,-2.57161807835228));
#15294=CARTESIAN_POINT('Ctrl Pts',(10.6072435897434,-1.64548597436975,-2.66083432711599));
#15295=CARTESIAN_POINT('Ctrl Pts',(10.6229487179466,-1.509186930649,-2.74024633660057));
#15296=CARTESIAN_POINT('Ctrl Pts',(10.6386538461515,-1.36775803719504,-2.80910392412142));
#15297=CARTESIAN_POINT('Ctrl Pts',(10.6543589743566,-1.22632914373961,-2.87796151164299));
#15298=CARTESIAN_POINT('Ctrl Pts',(10.6700641025633,-1.07975715593558,-2.9362712759061));
#15299=CARTESIAN_POINT('Ctrl Pts',(10.6857692307683,-0.929617596829541,
-2.98324879794393));
#15300=CARTESIAN_POINT('Ctrl Pts',(10.6967627558707,-0.82452052341797,-3.01613287001461));
#15301=CARTESIAN_POINT('Ctrl Pts',(10.7077562809724,-0.717669381189646,
-3.04346332885533));
#15302=CARTESIAN_POINT('Ctrl Pts',(10.718749806074,-0.609657256300376,-3.06495400126008));
#15303=CARTESIAN_POINT('Ctrl Pts',(10.7234614091763,-0.563365438343646,
-3.07416446995282));
#15304=CARTESIAN_POINT('Ctrl Pts',(10.7281730122785,-0.516860431844721,
-3.08230245321972));
#15305=CARTESIAN_POINT('Ctrl Pts',(10.7328846153808,-0.470193579471047,
-3.08937038670253));
#15306=CARTESIAN_POINT('Ctrl Pts',(10.748589743585,-0.31463953905291,-3.112929841749));
#15307=CARTESIAN_POINT('Ctrl Pts',(10.76429487179,-0.157306535044493,-3.12459764304402));
#15308=CARTESIAN_POINT('Ctrl Pts',(10.78,-3.21695909424879E-7,-3.12449703095644));
#15309=CARTESIAN_POINT('Ctrl Pts',(5.825978862952,0.9656781074217,2.972051613422));
#15310=CARTESIAN_POINT('Ctrl Pts',(5.879062196285,0.4599252670358,3.136380672689));
#15311=CARTESIAN_POINT('Ctrl Pts',(5.985228862952,-0.6366272854614,3.200971110614));
#15312=CARTESIAN_POINT('Ctrl Pts',(6.144478862952,-2.119635939241,2.481754111378));
#15313=CARTESIAN_POINT('Ctrl Pts',(6.303728862952,-3.061979863765,1.129624298873));
#15314=CARTESIAN_POINT('Ctrl Pts',(6.462978862952,-3.223532154246,-0.5105564866689));
#15315=CARTESIAN_POINT('Ctrl Pts',(6.622228862952,-2.563047905408,-2.020544571702));
#15316=CARTESIAN_POINT('Ctrl Pts',(6.781478862952,-1.248968678135,-3.015276776083));
#15317=CARTESIAN_POINT('Ctrl Pts',(6.940728862952,0.383608261101,-3.241089558554));
#15318=CARTESIAN_POINT('Ctrl Pts',(7.099978862952,1.918361836065,-2.640398557608));
#15319=CARTESIAN_POINT('Ctrl Pts',(7.259228862952,2.963917875123,-1.366384855545));
#15320=CARTESIAN_POINT('Ctrl Pts',(7.418478862952,3.253651172662,0.256067900963));
#15321=CARTESIAN_POINT('Ctrl Pts',(7.577728862952,2.713677441724,1.813221296591));
#15322=CARTESIAN_POINT('Ctrl Pts',(7.736978862952,1.481694291113,2.907988781792));
#15323=CARTESIAN_POINT('Ctrl Pts',(7.896228862952,-0.1281327360592,3.261195904774));
#15324=CARTESIAN_POINT('Ctrl Pts',(8.055478862952,-1.705284892359,2.782772028626));
#15325=CARTESIAN_POINT('Ctrl Pts',(8.214728862952,-2.84757578293,1.59471906236));
#15326=CARTESIAN_POINT('Ctrl Pts',(8.373978862952,-3.263712108535,0.));
#15327=CARTESIAN_POINT('Ctrl Pts',(8.533228862952,-2.84757578293,-1.59471906236));
#15328=CARTESIAN_POINT('Ctrl Pts',(8.692478862952,-1.705284892359,-2.782772028626));
#15329=CARTESIAN_POINT('Ctrl Pts',(8.851728862952,-0.1281327360592,-3.261195904774));
#15330=CARTESIAN_POINT('Ctrl Pts',(9.010978862952,1.481694291113,-2.907988781792));
#15331=CARTESIAN_POINT('Ctrl Pts',(9.170228862952,2.713677441724,-1.813221296591));
#15332=CARTESIAN_POINT('Ctrl Pts',(9.329478862952,3.253651172662,-0.256067900963));
#15333=CARTESIAN_POINT('Ctrl Pts',(9.488728862952,2.963917875123,1.366384855545));
#15334=CARTESIAN_POINT('Ctrl Pts',(9.647978862952,1.918361836065,2.640398557608));
#15335=CARTESIAN_POINT('Ctrl Pts',(9.807228862952,0.383608261101,3.241089558554));
#15336=CARTESIAN_POINT('Ctrl Pts',(9.966478862952,-1.248968678135,3.015276776083));
#15337=CARTESIAN_POINT('Ctrl Pts',(10.12572886295,-2.563047905408,2.020544571702));
#15338=CARTESIAN_POINT('Ctrl Pts',(10.28497886295,-3.223532154246,0.5105564866689));
#15339=CARTESIAN_POINT('Ctrl Pts',(10.44422886295,-3.061979863765,-1.129624298873));
#15340=CARTESIAN_POINT('Ctrl Pts',(10.60347886295,-2.119635939241,-2.481754111378));
#15341=CARTESIAN_POINT('Ctrl Pts',(10.76272886295,-0.6366272854614,-3.200971110614));
#15342=CARTESIAN_POINT('Ctrl Pts',(10.86889552962,0.4599252670358,-3.136380672689));
#15343=CARTESIAN_POINT('Ctrl Pts',(10.92197886295,0.9656781074217,-2.972051613422));
#15344=CARTESIAN_POINT('Ctrl Pts',(5.714992954317,0.9656781074217,2.972051613422));
#15345=CARTESIAN_POINT('Ctrl Pts',(5.768076287651,0.4599252670358,3.136380672689));
#15346=CARTESIAN_POINT('Ctrl Pts',(5.874242954317,-0.6366272854614,3.200971110614));
#15347=CARTESIAN_POINT('Ctrl Pts',(6.033492954317,-2.119635939241,2.481754111378));
#15348=CARTESIAN_POINT('Ctrl Pts',(6.192742954317,-3.061979863765,1.129624298873));
#15349=CARTESIAN_POINT('Ctrl Pts',(6.351992954317,-3.223532154246,-0.5105564866689));
#15350=CARTESIAN_POINT('Ctrl Pts',(6.511242954317,-2.563047905408,-2.020544571702));
#15351=CARTESIAN_POINT('Ctrl Pts',(6.670492954317,-1.248968678135,-3.015276776083));
#15352=CARTESIAN_POINT('Ctrl Pts',(6.829742954317,0.383608261101,-3.241089558554));
#15353=CARTESIAN_POINT('Ctrl Pts',(6.988992954317,1.918361836065,-2.640398557608));
#15354=CARTESIAN_POINT('Ctrl Pts',(7.148242954317,2.963917875123,-1.366384855545));
#15355=CARTESIAN_POINT('Ctrl Pts',(7.307492954317,3.253651172662,0.256067900963));
#15356=CARTESIAN_POINT('Ctrl Pts',(7.466742954317,2.713677441724,1.813221296591));
#15357=CARTESIAN_POINT('Ctrl Pts',(7.625992954317,1.481694291113,2.907988781792));
#15358=CARTESIAN_POINT('Ctrl Pts',(7.785242954317,-0.1281327360592,3.261195904774));
#15359=CARTESIAN_POINT('Ctrl Pts',(7.944492954317,-1.705284892359,2.782772028626));
#15360=CARTESIAN_POINT('Ctrl Pts',(8.103742954317,-2.84757578293,1.59471906236));
#15361=CARTESIAN_POINT('Ctrl Pts',(8.262992954317,-3.263712108535,0.));
#15362=CARTESIAN_POINT('Ctrl Pts',(8.422242954317,-2.84757578293,-1.59471906236));
#15363=CARTESIAN_POINT('Ctrl Pts',(8.581492954317,-1.705284892359,-2.782772028626));
#15364=CARTESIAN_POINT('Ctrl Pts',(8.740742954317,-0.1281327360592,-3.261195904774));
#15365=CARTESIAN_POINT('Ctrl Pts',(8.899992954317,1.481694291113,-2.907988781792));
#15366=CARTESIAN_POINT('Ctrl Pts',(9.059242954317,2.713677441724,-1.813221296591));
#15367=CARTESIAN_POINT('Ctrl Pts',(9.218492954317,3.253651172662,-0.256067900963));
#15368=CARTESIAN_POINT('Ctrl Pts',(9.377742954317,2.963917875123,1.366384855545));
#15369=CARTESIAN_POINT('Ctrl Pts',(9.536992954317,1.918361836065,2.640398557608));
#15370=CARTESIAN_POINT('Ctrl Pts',(9.696242954317,0.383608261101,3.241089558554));
#15371=CARTESIAN_POINT('Ctrl Pts',(9.855492954317,-1.248968678135,3.015276776083));
#15372=CARTESIAN_POINT('Ctrl Pts',(10.01474295432,-2.563047905408,2.020544571702));
#15373=CARTESIAN_POINT('Ctrl Pts',(10.17399295432,-3.223532154246,0.5105564866689));
#15374=CARTESIAN_POINT('Ctrl Pts',(10.33324295432,-3.061979863765,-1.129624298873));
#15375=CARTESIAN_POINT('Ctrl Pts',(10.49249295432,-2.119635939241,-2.481754111378));
#15376=CARTESIAN_POINT('Ctrl Pts',(10.65174295432,-0.6366272854614,-3.200971110614));
#15377=CARTESIAN_POINT('Ctrl Pts',(10.75790962098,0.4599252670358,-3.136380672689));
#15378=CARTESIAN_POINT('Ctrl Pts',(10.81099295432,0.9656781074217,-2.972051613422));
#15379=CARTESIAN_POINT('Ctrl Pts',(5.604007045683,0.9656781074217,2.972051613422));
#15380=CARTESIAN_POINT('Ctrl Pts',(5.657090379016,0.4599252670358,3.136380672689));
#15381=CARTESIAN_POINT('Ctrl Pts',(5.763257045683,-0.6366272854614,3.200971110614));
#15382=CARTESIAN_POINT('Ctrl Pts',(5.922507045683,-2.119635939241,2.481754111378));
#15383=CARTESIAN_POINT('Ctrl Pts',(6.081757045683,-3.061979863765,1.129624298873));
#15384=CARTESIAN_POINT('Ctrl Pts',(6.241007045683,-3.223532154246,-0.5105564866689));
#15385=CARTESIAN_POINT('Ctrl Pts',(6.400257045683,-2.563047905408,-2.020544571702));
#15386=CARTESIAN_POINT('Ctrl Pts',(6.559507045683,-1.248968678135,-3.015276776083));
#15387=CARTESIAN_POINT('Ctrl Pts',(6.718757045683,0.383608261101,-3.241089558554));
#15388=CARTESIAN_POINT('Ctrl Pts',(6.878007045683,1.918361836065,-2.640398557608));
#15389=CARTESIAN_POINT('Ctrl Pts',(7.037257045683,2.963917875123,-1.366384855545));
#15390=CARTESIAN_POINT('Ctrl Pts',(7.196507045683,3.253651172662,0.256067900963));
#15391=CARTESIAN_POINT('Ctrl Pts',(7.355757045683,2.713677441724,1.813221296591));
#15392=CARTESIAN_POINT('Ctrl Pts',(7.515007045683,1.481694291113,2.907988781792));
#15393=CARTESIAN_POINT('Ctrl Pts',(7.674257045683,-0.1281327360592,3.261195904774));
#15394=CARTESIAN_POINT('Ctrl Pts',(7.833507045683,-1.705284892359,2.782772028626));
#15395=CARTESIAN_POINT('Ctrl Pts',(7.992757045683,-2.84757578293,1.59471906236));
#15396=CARTESIAN_POINT('Ctrl Pts',(8.152007045683,-3.263712108535,0.));
#15397=CARTESIAN_POINT('Ctrl Pts',(8.311257045683,-2.84757578293,-1.59471906236));
#15398=CARTESIAN_POINT('Ctrl Pts',(8.470507045683,-1.705284892359,-2.782772028626));
#15399=CARTESIAN_POINT('Ctrl Pts',(8.629757045683,-0.1281327360592,-3.261195904774));
#15400=CARTESIAN_POINT('Ctrl Pts',(8.789007045683,1.481694291113,-2.907988781792));
#15401=CARTESIAN_POINT('Ctrl Pts',(8.948257045683,2.713677441724,-1.813221296591));
#15402=CARTESIAN_POINT('Ctrl Pts',(9.107507045683,3.253651172662,-0.256067900963));
#15403=CARTESIAN_POINT('Ctrl Pts',(9.266757045683,2.963917875123,1.366384855545));
#15404=CARTESIAN_POINT('Ctrl Pts',(9.426007045683,1.918361836065,2.640398557608));
#15405=CARTESIAN_POINT('Ctrl Pts',(9.585257045683,0.383608261101,3.241089558554));
#15406=CARTESIAN_POINT('Ctrl Pts',(9.744507045683,-1.248968678135,3.015276776083));
#15407=CARTESIAN_POINT('Ctrl Pts',(9.903757045683,-2.563047905408,2.020544571702));
#15408=CARTESIAN_POINT('Ctrl Pts',(10.06300704568,-3.223532154246,0.5105564866689));
#15409=CARTESIAN_POINT('Ctrl Pts',(10.22225704568,-3.061979863765,-1.129624298873));
#15410=CARTESIAN_POINT('Ctrl Pts',(10.38150704568,-2.119635939241,-2.481754111378));
#15411=CARTESIAN_POINT('Ctrl Pts',(10.54075704568,-0.6366272854614,-3.200971110614));
#15412=CARTESIAN_POINT('Ctrl Pts',(10.64692371235,0.4599252670358,-3.136380672689));
#15413=CARTESIAN_POINT('Ctrl Pts',(10.70000704568,0.9656781074217,-2.972051613422));
#15414=CARTESIAN_POINT('Ctrl Pts',(5.493021137048,0.9656781074217,2.972051613422));
#15415=CARTESIAN_POINT('Ctrl Pts',(5.546104470382,0.4599252670358,3.136380672689));
#15416=CARTESIAN_POINT('Ctrl Pts',(5.652271137048,-0.6366272854614,3.200971110614));
#15417=CARTESIAN_POINT('Ctrl Pts',(5.811521137048,-2.119635939241,2.481754111378));
#15418=CARTESIAN_POINT('Ctrl Pts',(5.970771137048,-3.061979863765,1.129624298873));
#15419=CARTESIAN_POINT('Ctrl Pts',(6.130021137048,-3.223532154246,-0.5105564866689));
#15420=CARTESIAN_POINT('Ctrl Pts',(6.289271137048,-2.563047905408,-2.020544571702));
#15421=CARTESIAN_POINT('Ctrl Pts',(6.448521137048,-1.248968678135,-3.015276776083));
#15422=CARTESIAN_POINT('Ctrl Pts',(6.607771137048,0.383608261101,-3.241089558554));
#15423=CARTESIAN_POINT('Ctrl Pts',(6.767021137048,1.918361836065,-2.640398557608));
#15424=CARTESIAN_POINT('Ctrl Pts',(6.926271137048,2.963917875123,-1.366384855545));
#15425=CARTESIAN_POINT('Ctrl Pts',(7.085521137048,3.253651172662,0.256067900963));
#15426=CARTESIAN_POINT('Ctrl Pts',(7.244771137048,2.713677441724,1.813221296591));
#15427=CARTESIAN_POINT('Ctrl Pts',(7.404021137048,1.481694291113,2.907988781792));
#15428=CARTESIAN_POINT('Ctrl Pts',(7.563271137048,-0.1281327360592,3.261195904774));
#15429=CARTESIAN_POINT('Ctrl Pts',(7.722521137048,-1.705284892359,2.782772028626));
#15430=CARTESIAN_POINT('Ctrl Pts',(7.881771137048,-2.84757578293,1.59471906236));
#15431=CARTESIAN_POINT('Ctrl Pts',(8.041021137048,-3.263712108535,0.));
#15432=CARTESIAN_POINT('Ctrl Pts',(8.200271137048,-2.84757578293,-1.59471906236));
#15433=CARTESIAN_POINT('Ctrl Pts',(8.359521137048,-1.705284892359,-2.782772028626));
#15434=CARTESIAN_POINT('Ctrl Pts',(8.518771137048,-0.1281327360592,-3.261195904774));
#15435=CARTESIAN_POINT('Ctrl Pts',(8.678021137048,1.481694291113,-2.907988781792));
#15436=CARTESIAN_POINT('Ctrl Pts',(8.837271137048,2.713677441724,-1.813221296591));
#15437=CARTESIAN_POINT('Ctrl Pts',(8.996521137048,3.253651172662,-0.256067900963));
#15438=CARTESIAN_POINT('Ctrl Pts',(9.155771137048,2.963917875123,1.366384855545));
#15439=CARTESIAN_POINT('Ctrl Pts',(9.315021137048,1.918361836065,2.640398557608));
#15440=CARTESIAN_POINT('Ctrl Pts',(9.474271137048,0.383608261101,3.241089558554));
#15441=CARTESIAN_POINT('Ctrl Pts',(9.633521137048,-1.248968678135,3.015276776083));
#15442=CARTESIAN_POINT('Ctrl Pts',(9.792771137048,-2.563047905408,2.020544571702));
#15443=CARTESIAN_POINT('Ctrl Pts',(9.952021137048,-3.223532154246,0.5105564866689));
#15444=CARTESIAN_POINT('Ctrl Pts',(10.11127113705,-3.061979863765,-1.129624298873));
#15445=CARTESIAN_POINT('Ctrl Pts',(10.27052113705,-2.119635939241,-2.481754111378));
#15446=CARTESIAN_POINT('Ctrl Pts',(10.42977113705,-0.6366272854614,-3.200971110614));
#15447=CARTESIAN_POINT('Ctrl Pts',(10.53593780372,0.4599252670358,-3.136380672689));
#15448=CARTESIAN_POINT('Ctrl Pts',(10.58902113705,0.9656781074217,-2.972051613422));
#15449=CARTESIAN_POINT('Origin',(32.48,0.,0.));
#15450=CARTESIAN_POINT('',(32.48,-1.1719681554584,0.434730540210171));
#15451=CARTESIAN_POINT('',(32.48,0.,-1.25));
#15452=CARTESIAN_POINT('Origin',(32.48,0.,0.));
#15453=CARTESIAN_POINT('',(32.48,-2.14581966314199E-13,-1.01129910075941));
#15454=CARTESIAN_POINT('',(32.48,0.,-1.25));
#15455=CARTESIAN_POINT('',(32.4802091864294,-1.17417484703353,0.42767483665679));
#15456=CARTESIAN_POINT('Ctrl Pts',(32.48,-1.17383720045579,0.427540834752428));
#15457=CARTESIAN_POINT('Ctrl Pts',(32.48,-1.20334957755843,0.312634815856706));
#15458=CARTESIAN_POINT('Ctrl Pts',(32.4800000000088,-1.21675226571292,0.19356365786419));
#15459=CARTESIAN_POINT('Ctrl Pts',(32.4800000000088,-1.20746725502762,-0.0403383382890132));
#15460=CARTESIAN_POINT('Ctrl Pts',(32.4800000000088,-1.18562847337316,-0.154733104489758));
#15461=CARTESIAN_POINT('Ctrl Pts',(32.4800000000088,-1.10111226718253,-0.400206118254704));
#15462=CARTESIAN_POINT('Ctrl Pts',(32.4800000000088,-1.02915837108193,-0.528561609151227));
#15463=CARTESIAN_POINT('Ctrl Pts',(32.4800000000088,-0.830791286197287,
-0.76065705947605));
#15464=CARTESIAN_POINT('Ctrl Pts',(32.4800000000088,-0.714027251240835,
-0.842690493865625));
#15465=CARTESIAN_POINT('Ctrl Pts',(32.4800000000088,-0.51664509754878,-0.946705547829938));
#15466=CARTESIAN_POINT('Ctrl Pts',(32.4800000000088,-0.414397116935866,
-0.982897616104408));
#15467=CARTESIAN_POINT('Ctrl Pts',(32.4800000000088,-0.20674106525062,-1.02124569796361));
#15468=CARTESIAN_POINT('Ctrl Pts',(32.48,-0.103645908104796,-1.02416362464409));
#15469=CARTESIAN_POINT('Ctrl Pts',(32.48,-2.15071016551605E-13,-1.0112991007594));
#15470=CARTESIAN_POINT('Ctrl Pts',(32.4802091864294,-1.17451603719175,0.427799109839404));
#15471=CARTESIAN_POINT('Ctrl Pts',(32.4801394576196,-1.17367357079685,0.430112088685898));
#15472=CARTESIAN_POINT('Ctrl Pts',(32.4800697288098,-1.17282427194519,0.43242257891675));
#15473=CARTESIAN_POINT('Ctrl Pts',(32.48,-1.1719681554584,0.434730540210171));
#15474=CARTESIAN_POINT('Origin',(32.48,0.,0.));
#15475=CARTESIAN_POINT('',(32.1675060170811,-9.34798452714434E-6,-1.24978906897538));
#15476=CARTESIAN_POINT('Ctrl Pts',(32.1676274246727,-1.60399786011158E-5,
-1.24999999989709));
#15477=CARTESIAN_POINT('Ctrl Pts',(32.173598380776,0.101438842794184,-1.25000130176441));
#15478=CARTESIAN_POINT('Ctrl Pts',(32.1795714326686,0.202526354544554,-1.2376506761652));
#15479=CARTESIAN_POINT('Ctrl Pts',(32.1896850767944,0.374326908675496,-1.19502535756305));
#15480=CARTESIAN_POINT('Ctrl Pts',(32.1938937983711,0.445845258510437,-1.1702260433228));
#15481=CARTESIAN_POINT('Ctrl Pts',(32.2022210789359,0.582164826348471,-1.10863277573242));
#15482=CARTESIAN_POINT('Ctrl Pts',(32.206334668102,0.646791699941685,-1.07221388529247));
#15483=CARTESIAN_POINT('Ctrl Pts',(32.2162391802242,0.787720814155092,-0.975394050833982));
#15484=CARTESIAN_POINT('Ctrl Pts',(32.2220182599191,0.860966724127556,-0.911391666503034));
#15485=CARTESIAN_POINT('Ctrl Pts',(32.2349867690631,1.01056382152689,-0.746379439126566));
#15486=CARTESIAN_POINT('Ctrl Pts',(32.2419708632708,1.08050014479524,-0.640970847678421));
#15487=CARTESIAN_POINT('Ctrl Pts',(32.2526890486056,1.16157362526215,-0.466556119290835));
#15488=CARTESIAN_POINT('Ctrl Pts',(32.256422258516,1.18475666984318,-0.40407812892699));
#15489=CARTESIAN_POINT('Ctrl Pts',(32.2659674336806,1.22941045910993,-0.246123517505284));
#15490=CARTESIAN_POINT('Ctrl Pts',(32.271780145632,1.24487129761986,-0.149410654725891));
#15491=CARTESIAN_POINT('Ctrl Pts',(32.2859186906479,1.25497749106622,0.0938655035164218));
#15492=CARTESIAN_POINT('Ctrl Pts',(32.2938682048,1.23547411642577,0.239545986671451));
#15493=CARTESIAN_POINT('Ctrl Pts',(32.3059208801052,1.17059722602897,0.44370420020077));
#15494=CARTESIAN_POINT('Ctrl Pts',(32.3098837877495,1.14459344270278,0.507025730539694));
#15495=CARTESIAN_POINT('Ctrl Pts',(32.3173248114395,1.08715439549203,0.619653609883257));
#15496=CARTESIAN_POINT('Ctrl Pts',(32.3207565858864,1.05718301811824,0.669506992419299));
#15497=CARTESIAN_POINT('Ctrl Pts',(32.3310964721333,0.955559897167941,0.814602243645237));
#15498=CARTESIAN_POINT('Ctrl Pts',(32.337764005247,0.873685600999364,0.901858257853645));
#15499=CARTESIAN_POINT('Ctrl Pts',(32.3492547954888,0.712478996094717,1.03077898081134));
#15500=CARTESIAN_POINT('Ctrl Pts',(32.354132063387,0.638731111457185,1.07803216370618));
#15501=CARTESIAN_POINT('Ctrl Pts',(32.3677278070184,0.430804719901573,1.18237689339029));
#15502=CARTESIAN_POINT('Ctrl Pts',(32.3763140626297,0.290556856108505,1.22441585209194));
#15503=CARTESIAN_POINT('Ctrl Pts',(32.3899887212276,0.0499212726420179,
1.25276221308346));
#15504=CARTESIAN_POINT('Ctrl Pts',(32.3952913518613,-0.0473830247951738,
1.25286037601624));
#15505=CARTESIAN_POINT('Ctrl Pts',(32.4046759695241,-0.212324572615296,
1.23377004596013));
#15506=CARTESIAN_POINT('Ctrl Pts',(32.4087137640163,-0.280149151477129,
1.22015755740893));
#15507=CARTESIAN_POINT('Ctrl Pts',(32.4201985488141,-0.4674169888626,1.16613067923734));
#15508=CARTESIAN_POINT('Ctrl Pts',(32.42752145001,-0.582393583035011,1.1131771414791));
#15509=CARTESIAN_POINT('Ctrl Pts',(32.4400656595717,-0.768674742918102,
0.990495494343983));
#15510=CARTESIAN_POINT('Ctrl Pts',(32.4453720504446,-0.843314336264057,
0.927772317335062));
#15511=CARTESIAN_POINT('Ctrl Pts',(32.4552603593318,-0.962519242690118,
0.801211161419528));
#15512=CARTESIAN_POINT('Ctrl Pts',(32.4597919513534,-1.00985081030901,0.740662982862584));
#15513=CARTESIAN_POINT('Ctrl Pts',(32.4696271054798,-1.10014034401452,0.600277310531608));
#15514=CARTESIAN_POINT('Ctrl Pts',(32.4748779535446,-1.14058809545123,0.519326462610753));
#15515=CARTESIAN_POINT('Ctrl Pts',(32.48,-1.1719681554584,0.434730540210171));
#15516=CARTESIAN_POINT('',(32.48,0.,-1.25));
#15517=CARTESIAN_POINT('Origin',(32.48,0.,-1.25));
#15518=CARTESIAN_POINT('',(32.3083865332472,-1.15233060718194E-10,-1.00548172098699));
#15519=CARTESIAN_POINT('Ctrl Pts',(32.3083865336658,6.75598583770804E-18,
-1.00548172122881));
#15520=CARTESIAN_POINT('Ctrl Pts',(32.2848226217472,2.79433020236803E-15,
-1.04627458705313));
#15521=CARTESIAN_POINT('Ctrl Pts',(32.2612587098288,2.84235642030823E-12,
-1.08706745287754));
#15522=CARTESIAN_POINT('Ctrl Pts',(32.2142255996871,2.84235642030823E-12,
-1.16848922011001));
#15523=CARTESIAN_POINT('Ctrl Pts',(32.1907564014637,1.40940692139627E-14,
-1.20911812151808));
#15524=CARTESIAN_POINT('Ctrl Pts',(32.1672872032404,4.46512479480176E-17,
-1.24974702292624));
#15525=CARTESIAN_POINT('',(32.4766396034691,1.02451809110596E-10,-1.00548172094448));
#15526=CARTESIAN_POINT('Ctrl Pts',(32.4766396034691,1.97433788701479E-19,
-1.00548172051374));
#15527=CARTESIAN_POINT('Ctrl Pts',(32.4485930689794,2.17707619891981E-17,
-1.00548172051374));
#15528=CARTESIAN_POINT('Ctrl Pts',(32.4205465344897,1.80411241501588E-15,
-1.00548172051374));
#15529=CARTESIAN_POINT('Ctrl Pts',(32.3644621777491,1.80411241501588E-15,
-1.00548172051374));
#15530=CARTESIAN_POINT('Ctrl Pts',(32.3364243554981,2.28527355790286E-17,
-1.00548172051374));
#15531=CARTESIAN_POINT('Ctrl Pts',(32.3083865332471,2.17567656864905E-19,
-1.00548172051374));
#15532=CARTESIAN_POINT('Ctrl Pts',(32.48,-4.28248633902167E-13,-1.01129910075941));
#15533=CARTESIAN_POINT('Ctrl Pts',(32.4795160656876,-1.34558093608641E-12,
-1.01046133377316));
#15534=CARTESIAN_POINT('Ctrl Pts',(32.4790321313751,-3.41777979044421E-12,
-1.00962356678695));
#15535=CARTESIAN_POINT('Ctrl Pts',(32.4779119990709,-3.41777979044421E-12,
-1.00768444025543));
#15536=CARTESIAN_POINT('Ctrl Pts',(32.4772758010794,-1.44173449374501E-13,
-1.00658308071008));
#15537=CARTESIAN_POINT('Ctrl Pts',(32.4766396030876,-4.57272161567443E-15,
-1.00548172116484));
#15538=CARTESIAN_POINT('Ctrl Pts',(32.66948943148,0.523912106125,-1.17672585665));
#15539=CARTESIAN_POINT('Ctrl Pts',(32.65323943148,0.2569214784303,-1.295597742809));
#15540=CARTESIAN_POINT('Ctrl Pts',(32.62073943148,-0.3599776781819,-1.343968209978));
#15541=CARTESIAN_POINT('Ctrl Pts',(32.57198943148,-1.125748737002,-0.8178925633062));
#15542=CARTESIAN_POINT('Ctrl Pts',(32.52323943148,-1.389532103288,0.07282787068193));
#15543=CARTESIAN_POINT('Ctrl Pts',(32.47448943148,-1.034052055861,0.9310606109295));
#15544=CARTESIAN_POINT('Ctrl Pts',(32.42573943148,-0.2176699703233,1.374319545129));
#15545=CARTESIAN_POINT('Ctrl Pts',(32.37698943148,0.6957249084782,1.205031167107));
#15546=CARTESIAN_POINT('Ctrl Pts',(32.32823943148,1.299030774048,0.4986511981073));
#15547=CARTESIAN_POINT('Ctrl Pts',(32.27948943148,1.323347810262,-0.4299817804464));
#15548=CARTESIAN_POINT('Ctrl Pts',(32.23073943148,0.7578381246551,-1.166968368163));
#15549=CARTESIAN_POINT('Ctrl Pts',(32.18198943148,-0.14544615728,-1.383827738746));
#15550=CARTESIAN_POINT('Ctrl Pts',(32.13323943148,-0.9839039059594,-0.9839039061246));
#15551=CARTESIAN_POINT('Ctrl Pts',(32.08448943148,-1.383827738331,-0.1454461562038));
#15552=CARTESIAN_POINT('Ctrl Pts',(32.03573943148,-1.166968369989,0.7578381205155));
#15553=CARTESIAN_POINT('Ctrl Pts',(31.98698943148,-0.4299817735579,1.323347825744));
#15554=CARTESIAN_POINT('Ctrl Pts',(31.93823943148,0.4986511723795,1.299030716259));
#15555=CARTESIAN_POINT('Ctrl Pts',(31.88948943148,1.20503126313,0.69572512415));
#15556=CARTESIAN_POINT('Ctrl Pts',(31.84073943148,1.374319186766,-0.217670775222));
#15557=CARTESIAN_POINT('Ctrl Pts',(31.79198943148,0.9310619483586,-1.034049051938));
#15558=CARTESIAN_POINT('Ctrl Pts',(31.74323943148,0.07282287932824,-1.389543314081));
#15559=CARTESIAN_POINT('Ctrl Pts',(31.69448943148,-0.8178739353206,-1.125706897754));
#15560=CARTESIAN_POINT('Ctrl Pts',(31.64573943148,-1.344037730566,-0.3601338243812));
#15561=CARTESIAN_POINT('Ctrl Pts',(31.59698943148,-1.271153054855,0.5659538022856));
#15562=CARTESIAN_POINT('Ctrl Pts',(31.54823943148,-0.6317051899145,1.239791251989));
#15563=CARTESIAN_POINT('Ctrl Pts',(31.49948943148,0.2892987601002,1.361043711953));
#15564=CARTESIAN_POINT('Ctrl Pts',(31.45073943148,1.081359992212,0.8756680515693));
#15565=CARTESIAN_POINT('Ctrl Pts',(31.40198943148,1.391450057306,-1.387658967178E-7));
#15566=CARTESIAN_POINT('Ctrl Pts',(31.35323943148,1.081360653838,-0.8756674965057));
#15567=CARTESIAN_POINT('Ctrl Pts',(31.30448943148,0.2892961135977,-1.361045654676));
#15568=CARTESIAN_POINT('Ctrl Pts',(31.25573943148,-0.6316952655301,-1.239784036163));
#15569=CARTESIAN_POINT('Ctrl Pts',(31.20698943148,-1.271190105891,-0.5659807228689));
#15570=CARTESIAN_POINT('Ctrl Pts',(31.15823943148,-1.34389945081,0.360234290888));
#15571=CARTESIAN_POINT('Ctrl Pts',(31.12573943148,-0.9935598191429,0.8702993985029));
#15572=CARTESIAN_POINT('Ctrl Pts',(31.10948943148,-0.7571184320868,1.04208412158));
#15573=CARTESIAN_POINT('Ctrl Pts',(32.6078719886,0.4805033243013,-1.079228136364));
#15574=CARTESIAN_POINT('Ctrl Pts',(32.5916219886,0.2356342276251,-1.18825088235));
#15575=CARTESIAN_POINT('Ctrl Pts',(32.5591219886,-0.330151697238,-1.232613610374));
#15576=CARTESIAN_POINT('Ctrl Pts',(32.5103719886,-1.032474730272,-0.7501260058613));
#15577=CARTESIAN_POINT('Ctrl Pts',(32.4616219886,-1.274402303455,0.06679371130261));
#15578=CARTESIAN_POINT('Ctrl Pts',(32.4128719886,-0.9483755853946,0.8539175053361));
#15579=CARTESIAN_POINT('Ctrl Pts',(32.3641219886,-0.199634906539,1.260450183087));
#15580=CARTESIAN_POINT('Ctrl Pts',(32.3153719886,0.6380805623973,1.105188207931));
#15581=CARTESIAN_POINT('Ctrl Pts',(32.2666219886,1.191399469495,0.457335410952));
#15582=CARTESIAN_POINT('Ctrl Pts',(32.2178719886,1.21370171562,-0.3943556036939));
#15583=CARTESIAN_POINT('Ctrl Pts',(32.1691219886,0.6950473827993,-1.07027910541));
#15584=CARTESIAN_POINT('Ctrl Pts',(32.1203719886,-0.1333952036284,-1.269170574518));
#15585=CARTESIAN_POINT('Ctrl Pts',(32.0716219886,-0.902382464691,-0.9023824648425));
#15586=CARTESIAN_POINT('Ctrl Pts',(32.0228719886,-1.269170574137,-0.1333952026413));
#15587=CARTESIAN_POINT('Ctrl Pts',(31.9741219886,-1.070279107084,0.6950473790027));
#15588=CARTESIAN_POINT('Ctrl Pts',(31.9253719886,-0.3943555973762,1.213701729819));
#15589=CARTESIAN_POINT('Ctrl Pts',(31.8766219886,0.4573353873559,1.191399416495));
#15590=CARTESIAN_POINT('Ctrl Pts',(31.8278719886,1.105188295998,0.6380807601996));
#15591=CARTESIAN_POINT('Ctrl Pts',(31.7791219886,1.260449854417,-0.1996356447478));
#15592=CARTESIAN_POINT('Ctrl Pts',(31.7303719886,0.8539187319524,-0.948372830362));
#15593=CARTESIAN_POINT('Ctrl Pts',(31.6816219886,0.06678913350795,-1.274412585376));
#15594=CARTESIAN_POINT('Ctrl Pts',(31.6328719886,-0.7501089212991,-1.032436357618));
#15595=CARTESIAN_POINT('Ctrl Pts',(31.5841219886,-1.232677370829,-0.3302949059307));
#15596=CARTESIAN_POINT('Ctrl Pts',(31.5353719886,-1.165831561083,0.519061652174));
#15597=CARTESIAN_POINT('Ctrl Pts',(31.4866219886,-0.5793652030249,1.137068243043));
#15598=CARTESIAN_POINT('Ctrl Pts',(31.4378719886,0.2653288868863,1.248274320191));
#15599=CARTESIAN_POINT('Ctrl Pts',(31.3891219886,0.9917638186823,0.8031145011624));
#15600=CARTESIAN_POINT('Ctrl Pts',(31.3403719886,1.27616134523,-1.272684365758E-7));
#15601=CARTESIAN_POINT('Ctrl Pts',(31.2916219886,0.9917644254889,-0.8031139920886));
#15602=CARTESIAN_POINT('Ctrl Pts',(31.2428719886,0.26532645966,-1.248276101949));
#15603=CARTESIAN_POINT('Ctrl Pts',(31.1941219886,-0.5793561009262,-1.137061625084));
#15604=CARTESIAN_POINT('Ctrl Pts',(31.1453719886,-1.165865542251,-0.5190863422501));
#15605=CARTESIAN_POINT('Ctrl Pts',(31.0966219886,-1.232550548254,0.3303870482766));
#15606=CARTESIAN_POINT('Ctrl Pts',(31.0641219886,-0.9112383363718,0.7981906682994));
#15607=CARTESIAN_POINT('Ctrl Pts',(31.0478719886,-0.6943873204195,0.9557421536299));
#15608=CARTESIAN_POINT('Ctrl Pts',(32.54625454572,0.4370945424777,-0.9817304160777));
#15609=CARTESIAN_POINT('Ctrl Pts',(32.53000454572,0.2143469768198,-1.080904021891));
#15610=CARTESIAN_POINT('Ctrl Pts',(32.49750454572,-0.300325716294,-1.121259010771));
#15611=CARTESIAN_POINT('Ctrl Pts',(32.44875454572,-0.9392007235413,-0.6823594484165));
#15612=CARTESIAN_POINT('Ctrl Pts',(32.40000454572,-1.159272503621,0.06075955192328));
#15613=CARTESIAN_POINT('Ctrl Pts',(32.35125454572,-0.8626991149286,0.7767743997427));
#15614=CARTESIAN_POINT('Ctrl Pts',(32.30250454572,-0.1815998427547,1.146580821045));
#15615=CARTESIAN_POINT('Ctrl Pts',(32.25375454572,0.5804362163164,1.005345248755));
#15616=CARTESIAN_POINT('Ctrl Pts',(32.20500454572,1.083768164943,0.4160196237966));
#15617=CARTESIAN_POINT('Ctrl Pts',(32.15625454572,1.104055620977,-0.3587294269415));
#15618=CARTESIAN_POINT('Ctrl Pts',(32.10750454572,0.6322566409435,-0.9735898426565));
#15619=CARTESIAN_POINT('Ctrl Pts',(32.05875454572,-0.1213442499767,-1.154513410291));
#15620=CARTESIAN_POINT('Ctrl Pts',(32.01000454572,-0.8208610234226,-0.8208610235605));
#15621=CARTESIAN_POINT('Ctrl Pts',(31.96125454572,-1.154513409944,-0.1213442490788));
#15622=CARTESIAN_POINT('Ctrl Pts',(31.91250454572,-0.9735898441798,0.6322566374899));
#15623=CARTESIAN_POINT('Ctrl Pts',(31.86375454572,-0.3587294211945,1.104055633894));
#15624=CARTESIAN_POINT('Ctrl Pts',(31.81500454572,0.4160196023322,1.083768116731));
#15625=CARTESIAN_POINT('Ctrl Pts',(31.76625454572,1.005345328866,0.5804363962492));
#15626=CARTESIAN_POINT('Ctrl Pts',(31.71750454572,1.146580522067,-0.1816005142735));
#15627=CARTESIAN_POINT('Ctrl Pts',(31.66875454572,0.7767755155462,-0.8626966087863));
#15628=CARTESIAN_POINT('Ctrl Pts',(31.62000454572,0.06075538768766,-1.159281856671));
#15629=CARTESIAN_POINT('Ctrl Pts',(31.57125454572,-0.6823439072776,-0.9391658174822));
#15630=CARTESIAN_POINT('Ctrl Pts',(31.52250454572,-1.121317011091,-0.3004559874802));
#15631=CARTESIAN_POINT('Ctrl Pts',(31.47375454572,-1.06051006731,0.4721695020624));
#15632=CARTESIAN_POINT('Ctrl Pts',(31.42500454572,-0.5270252161353,1.034345234097));
#15633=CARTESIAN_POINT('Ctrl Pts',(31.37625454572,0.2413590136724,1.135504928428));
#15634=CARTESIAN_POINT('Ctrl Pts',(31.32750454572,0.9021676451524,0.7305609507554));
#15635=CARTESIAN_POINT('Ctrl Pts',(31.27875454572,1.160872633154,-1.157709766638E-7));
#15636=CARTESIAN_POINT('Ctrl Pts',(31.23000454572,0.9021681971399,-0.7305604876715));
#15637=CARTESIAN_POINT('Ctrl Pts',(31.18125454572,0.2413568057222,-1.135506549222));
#15638=CARTESIAN_POINT('Ctrl Pts',(31.13250454572,-0.5270169363223,-1.034339214006));
#15639=CARTESIAN_POINT('Ctrl Pts',(31.08375454572,-1.060540978612,-0.4721919616313));
#15640=CARTESIAN_POINT('Ctrl Pts',(31.03500454572,-1.121201645697,0.3005398056652));
#15641=CARTESIAN_POINT('Ctrl Pts',(31.00250454572,-0.8289168536006,0.7260819380959));
#15642=CARTESIAN_POINT('Ctrl Pts',(30.98625454572,-0.6316562087523,0.86940018568));
#15643=CARTESIAN_POINT('Ctrl Pts',(32.48463710284,0.393685760654,-0.8842326957913));
#15644=CARTESIAN_POINT('Ctrl Pts',(32.46838710284,0.1930597260145,-0.9735571614325));
#15645=CARTESIAN_POINT('Ctrl Pts',(32.43588710284,-0.2704997353501,-1.009904411168));
#15646=CARTESIAN_POINT('Ctrl Pts',(32.38713710284,-0.845926716811,-0.6145928909716));
#15647=CARTESIAN_POINT('Ctrl Pts',(32.33838710284,-1.044142703787,0.05472539254396));
#15648=CARTESIAN_POINT('Ctrl Pts',(32.28963710284,-0.7770226444626,0.6996312941493));
#15649=CARTESIAN_POINT('Ctrl Pts',(32.24088710284,-0.1635647789704,1.032711459003));
#15650=CARTESIAN_POINT('Ctrl Pts',(32.19213710284,0.5227918702356,0.905502289579));
#15651=CARTESIAN_POINT('Ctrl Pts',(32.14338710284,0.9761368603912,0.3747038366413));
#15652=CARTESIAN_POINT('Ctrl Pts',(32.09463710284,0.994409526335,-0.323103250189));
#15653=CARTESIAN_POINT('Ctrl Pts',(32.04588710284,0.5694658990877,-0.8769005799032));
#15654=CARTESIAN_POINT('Ctrl Pts',(31.99713710284,-0.109293296325,-1.039856246063));
#15655=CARTESIAN_POINT('Ctrl Pts',(31.94838710284,-0.7393395821542,-0.7393395822784));
#15656=CARTESIAN_POINT('Ctrl Pts',(31.89963710284,-1.039856245751,-0.1092932955163));
#15657=CARTESIAN_POINT('Ctrl Pts',(31.85088710284,-0.8769005812753,0.5694658959771));
#15658=CARTESIAN_POINT('Ctrl Pts',(31.80213710284,-0.3231032450128,0.9944095379687));
#15659=CARTESIAN_POINT('Ctrl Pts',(31.75338710284,0.3747038173086,0.9761368169669));
#15660=CARTESIAN_POINT('Ctrl Pts',(31.70463710284,0.9055023617337,0.5227920322988));
#15661=CARTESIAN_POINT('Ctrl Pts',(31.65588710284,1.032711189717,-0.1635653837993));
#15662=CARTESIAN_POINT('Ctrl Pts',(31.60713710284,0.69963229914,-0.7770203872106));
#15663=CARTESIAN_POINT('Ctrl Pts',(31.55838710284,0.05472164186737,-1.044151127966));
#15664=CARTESIAN_POINT('Ctrl Pts',(31.50963710284,-0.614578893256,-0.8458952773463));
#15665=CARTESIAN_POINT('Ctrl Pts',(31.46088710284,-1.009956651354,-0.2706170690297));
#15666=CARTESIAN_POINT('Ctrl Pts',(31.41213710284,-0.9551885735371,0.4252773519508));
#15667=CARTESIAN_POINT('Ctrl Pts',(31.36338710284,-0.4746852292457,0.9316222251505));
#15668=CARTESIAN_POINT('Ctrl Pts',(31.31463710284,0.2173891404585,1.022735536666));
#15669=CARTESIAN_POINT('Ctrl Pts',(31.26588710284,0.8125714716225,0.6580074003485));
#15670=CARTESIAN_POINT('Ctrl Pts',(31.21713710284,1.045583921078,-1.042735165158E-7));
#15671=CARTESIAN_POINT('Ctrl Pts',(31.16838710284,0.8125719687909,-0.6580069832544));
#15672=CARTESIAN_POINT('Ctrl Pts',(31.11963710284,0.2173871517845,-1.022736996495));
#15673=CARTESIAN_POINT('Ctrl Pts',(31.07088710284,-0.4746777717184,-0.9316168029278));
#15674=CARTESIAN_POINT('Ctrl Pts',(31.02213710284,-0.9552164149722,-0.4252975810124));
#15675=CARTESIAN_POINT('Ctrl Pts',(30.97338710284,-1.00985274314,0.2706925630538));
#15676=CARTESIAN_POINT('Ctrl Pts',(30.94088710284,-0.7465953708295,0.6539732078925));
#15677=CARTESIAN_POINT('Ctrl Pts',(30.92463710284,-0.568925097085,0.7830582177302));
#15678=CARTESIAN_POINT('',(30.9766265277784,-0.871221485969368,0.50299995921493));
#15679=CARTESIAN_POINT('Ctrl Pts',(32.4766396027226,1.54919549294486E-10,
-1.0054817205135));
#15680=CARTESIAN_POINT('Ctrl Pts',(32.4691053139096,-0.10582508315099,-1.00564870419041));
#15681=CARTESIAN_POINT('Ctrl Pts',(32.4603459018315,-0.229977486211365,
-0.98986838296787));
#15682=CARTESIAN_POINT('Ctrl Pts',(32.4413683240352,-0.478121855944446,
-0.893142660574254));
#15683=CARTESIAN_POINT('Ctrl Pts',(32.4325422614636,-0.585319685046669,
-0.82656883687245));
#15684=CARTESIAN_POINT('Ctrl Pts',(32.4142572992228,-0.775641550295082,
-0.654100595091286));
#15685=CARTESIAN_POINT('Ctrl Pts',(32.4050118930799,-0.85418371112365,-0.547761809504575));
#15686=CARTESIAN_POINT('Ctrl Pts',(32.3863010258111,-0.965161319461717,
-0.309559370165476));
#15687=CARTESIAN_POINT('Ctrl Pts',(32.3770681843843,-0.997469062168772,
-0.181353499720047));
#15688=CARTESIAN_POINT('Ctrl Pts',(32.3568701808033,-1.01283629382345,0.101717750507541));
#15689=CARTESIAN_POINT('Ctrl Pts',(32.3475047473001,-0.984367566826271,
0.232947114591686));
#15690=CARTESIAN_POINT('Ctrl Pts',(32.3306589696044,-0.904804400397718,
0.45589393306715));
#15691=CARTESIAN_POINT('Ctrl Pts',(32.3216600150562,-0.840300871347811,
0.56722203459221));
#15692=CARTESIAN_POINT('Ctrl Pts',(32.3025520369028,-0.663919325666475,
0.769080055430503));
#15693=CARTESIAN_POINT('Ctrl Pts',(32.2930478380112,-0.553320416471912,
0.848600935605224));
#15694=CARTESIAN_POINT('Ctrl Pts',(32.2764607849827,-0.34391489168562,0.950970008765668));
#15695=CARTESIAN_POINT('Ctrl Pts',(32.267274142459,-0.219359775122067,0.993525782886256));
#15696=CARTESIAN_POINT('Ctrl Pts',(32.2471250024671,0.0627872995112071,
1.01225002509461));
#15697=CARTESIAN_POINT('Ctrl Pts',(32.2377136687343,0.196496573752308,0.994659351660526));
#15698=CARTESIAN_POINT('Ctrl Pts',(32.218820619244,0.448119147312156,0.910386233646112));
#15699=CARTESIAN_POINT('Ctrl Pts',(32.2095672963117,0.562777737133873,0.844344677318313));
#15700=CARTESIAN_POINT('Ctrl Pts',(32.190863687752,0.759894331709125,0.670695233562694));
#15701=CARTESIAN_POINT('Ctrl Pts',(32.1816445339917,0.840830374658885,0.566410881442963));
#15702=CARTESIAN_POINT('Ctrl Pts',(32.1614385161676,0.968593109628251,0.31323629661574));
#15703=CARTESIAN_POINT('Ctrl Pts',(32.152059805267,0.995103645636241,0.181385312576402));
#15704=CARTESIAN_POINT('Ctrl Pts',(32.1352540053896,1.01170308102003,-0.0541913934911884));
#15705=CARTESIAN_POINT('Ctrl Pts',(32.126269951113,0.997390470348591,-0.181830481509641));
#15706=CARTESIAN_POINT('Ctrl Pts',(32.1077447657716,0.919423226898876,-0.429745166292925));
#15707=CARTESIAN_POINT('Ctrl Pts',(32.0982393193792,0.852869094566033,-0.54854223882289));
#15708=CARTESIAN_POINT('Ctrl Pts',(32.0810552458601,0.696891195219596,-0.73288046123264));
#15709=CARTESIAN_POINT('Ctrl Pts',(32.0718646719204,0.599816161628677,-0.821842509043154));
#15710=CARTESIAN_POINT('Ctrl Pts',(32.0517249713863,0.349028087285563,-0.952204354992639));
#15711=CARTESIAN_POINT('Ctrl Pts',(32.0423217182128,0.219635000613399,-0.989799618535102));
#15712=CARTESIAN_POINT('Ctrl Pts',(32.0234223525948,-0.0447199889143717,
-1.01375940902337));
#15713=CARTESIAN_POINT('Ctrl Pts',(32.0141578837072,-0.176402393566581,
-0.99923740432607));
#15714=CARTESIAN_POINT('Ctrl Pts',(31.9954668431444,-0.426500714921258,
-0.919407894705325));
#15715=CARTESIAN_POINT('Ctrl Pts',(31.9862599642796,-0.542364539351686,
-0.856538059210492));
#15716=CARTESIAN_POINT('Ctrl Pts',(31.9660429991874,-0.761220467435554,
-0.675972386498989));
#15717=CARTESIAN_POINT('Ctrl Pts',(31.9566507719093,-0.838493771813703,
-0.565639342750785));
#15718=CARTESIAN_POINT('Ctrl Pts',(31.9398838938876,-0.948125656391315,
-0.357081831558934));
#15719=CARTESIAN_POINT('Ctrl Pts',(31.9309137064797,-0.986297530771061,
-0.234667590561075));
#15720=CARTESIAN_POINT('Ctrl Pts',(31.9124152715538,-1.01458386847578,0.023295661735757));
#15721=CARTESIAN_POINT('Ctrl Pts',(31.9029118555964,-1.00153559313095,0.158814096445736));
#15722=CARTESIAN_POINT('Ctrl Pts',(31.8856873106528,-0.932797546195448,
0.390887587624591));
#15723=CARTESIAN_POINT('Ctrl Pts',(31.8764931007021,-0.879593330129118,
0.511383216351955));
#15724=CARTESIAN_POINT('Ctrl Pts',(31.8563616071714,-0.70241886040258,0.731471621586331));
#15725=CARTESIAN_POINT('Ctrl Pts',(31.8469659290911,-0.599170684072269,
0.817877985664088));
#15726=CARTESIAN_POINT('Ctrl Pts',(31.8280621443435,-0.366747863090102,
0.946194878116315));
#15727=CARTESIAN_POINT('Ctrl Pts',(31.818786283051,-0.240163206787939,0.985835062226092));
#15728=CARTESIAN_POINT('Ctrl Pts',(31.8001078040911,0.0207603676706945,
1.01327765451514));
#15729=CARTESIAN_POINT('Ctrl Pts',(31.7909121905271,0.15195887892012,1.00235989692945));
#15730=CARTESIAN_POINT('Ctrl Pts',(31.7706842229678,0.425111210006055,0.925080808596332));
#15731=CARTESIAN_POINT('Ctrl Pts',(31.761279437479,0.540347644379315,0.854950472866657));
#15732=CARTESIAN_POINT('Ctrl Pts',(31.7445489336977,0.724235313103983,0.708453750739634));
#15733=CARTESIAN_POINT('Ctrl Pts',(31.7355913796315,0.808338952205113,0.611915865043628));
#15734=CARTESIAN_POINT('Ctrl Pts',(31.7176616890085,0.934104160209125,0.394084134956314));
#15735=CARTESIAN_POINT('Ctrl Pts',(31.7087041349354,0.975656602098998,0.272979304096005));
#15736=CARTESIAN_POINT('Ctrl Pts',(31.691973631154,1.01058265066987,0.0404795504744009));
#15737=CARTESIAN_POINT('Ctrl Pts',(31.6825688456652,1.01369908580113,-0.0943832969990357));
#15738=CARTESIAN_POINT('Ctrl Pts',(31.6623408781059,0.944048573936179,-0.369579698988473));
#15739=CARTESIAN_POINT('Ctrl Pts',(31.6531452645421,0.887904373733188,-0.488659821461777));
#15740=CARTESIAN_POINT('Ctrl Pts',(31.6344667855823,0.733676604436161,-0.700904969244626));
#15741=CARTESIAN_POINT('Ctrl Pts',(31.6251909242898,0.63605486983531,-0.790710405276932));
#15742=CARTESIAN_POINT('Ctrl Pts',(31.6062871395422,0.408717770745883,-0.927836026440967));
#15743=CARTESIAN_POINT('Ctrl Pts',(31.5968914614619,0.282263576240687,-0.974048387998723));
#15744=CARTESIAN_POINT('Ctrl Pts',(31.5767599679311,0.00307419136583881,
-1.01744177706707));
#15745=CARTESIAN_POINT('Ctrl Pts',(31.5675657579804,-0.127880192190321,
-1.00327016540539));
#15746=CARTESIAN_POINT('Ctrl Pts',(31.5503412130368,-0.363230754564002,
-0.946762314668816));
#15747=CARTESIAN_POINT('Ctrl Pts',(31.5408377970794,-0.487117299376366,
-0.890303235238142));
#15748=CARTESIAN_POINT('Ctrl Pts',(31.5223393621535,-0.696376860255655,
-0.736824922057749));
#15749=CARTESIAN_POINT('Ctrl Pts',(31.5133691747455,-0.783304765554694,
-0.642559988636202));
#15750=CARTESIAN_POINT('Ctrl Pts',(31.4966022967237,-0.909104926108206,
-0.443337235931506));
#15751=CARTESIAN_POINT('Ctrl Pts',(31.4872100694454,-0.966019492682179,
-0.321250069431272));
#15752=CARTESIAN_POINT('Ctrl Pts',(31.4669931043532,-1.01296598826022,-0.0414324395852803));
#15753=CARTESIAN_POINT('Ctrl Pts',(31.4577862254883,-1.00948095071539,0.0903434934989293));
#15754=CARTESIAN_POINT('Ctrl Pts',(31.4390951849256,-0.953566173341268,
0.346849748046573));
#15755=CARTESIAN_POINT('Ctrl Pts',(31.429830716038,-0.900301395996993,0.46815105805527));
#15756=CARTESIAN_POINT('Ctrl Pts',(31.4109313504202,-0.747374114001067,
0.685109299359023));
#15757=CARTESIAN_POINT('Ctrl Pts',(31.4015280972467,-0.650119117375387,
0.778369367719778));
#15758=CARTESIAN_POINT('Ctrl Pts',(31.3813883967126,-0.411828409927458,
0.930377288092368));
#15759=CARTESIAN_POINT('Ctrl Pts',(31.3721978227729,-0.286247499755309,
0.969965709350148));
#15760=CARTESIAN_POINT('Ctrl Pts',(31.3550137492538,-0.0486169665865881,
1.01287742140833));
#15761=CARTESIAN_POINT('Ctrl Pts',(31.3455083028614,0.0875413822861097,
1.01111645447045));
#15762=CARTESIAN_POINT('Ctrl Pts',(31.3269831175199,0.341225419004652,0.95468072556934));
#15763=CARTESIAN_POINT('Ctrl Pts',(31.3179990632433,0.458920417080284,0.903256265996064));
#15764=CARTESIAN_POINT('Ctrl Pts',(31.3011932633659,0.654636111382735,0.771092380231486));
#15765=CARTESIAN_POINT('Ctrl Pts',(31.2918145524653,0.755567145070677,0.682208090561066));
#15766=CARTESIAN_POINT('Ctrl Pts',(31.2716085346413,0.91094139963879,0.444975024007283));
#15767=CARTESIAN_POINT('Ctrl Pts',(31.2623893808811,0.960786276316755,0.322740178671269));
#15768=CARTESIAN_POINT('Ctrl Pts',(31.2436857723214,1.0126128086746,0.0652074783839398));
#15769=CARTESIAN_POINT('Ctrl Pts',(31.2344324493892,1.01247717924913,-0.0671105513276969));
#15770=CARTESIAN_POINT('Ctrl Pts',(31.2155393998991,0.959648553525894,-0.327158651203486));
#15771=CARTESIAN_POINT('Ctrl Pts',(31.2061280661664,0.908027886468966,-0.451749616134968));
#15772=CARTESIAN_POINT('Ctrl Pts',(31.1859789261745,0.750738679733246,-0.686734029267041));
#15773=CARTESIAN_POINT('Ctrl Pts',(31.1767922836507,0.651606739985219,-0.77332403732232));
#15774=CARTESIAN_POINT('Ctrl Pts',(31.1602052306222,0.458249759673342,-0.903490004899917));
#15775=CARTESIAN_POINT('Ctrl Pts',(31.1507010317304,0.334083202713468,-0.959511029806068));
#15776=CARTESIAN_POINT('Ctrl Pts',(31.1315930535769,0.0710782558689687,
-1.0113329187058));
#15777=CARTESIAN_POINT('Ctrl Pts',(31.1225940990287,-0.057586472731709,
-1.01153056273425));
#15778=CARTESIAN_POINT('Ctrl Pts',(31.1057483213329,-0.290445664438458,
-0.968960876829247));
#15779=CARTESIAN_POINT('Ctrl Pts',(31.0963828878297,-0.418327990956272,
-0.928000835580201));
#15780=CARTESIAN_POINT('Ctrl Pts',(31.0761848842486,-0.655791268906789,
-0.773156797467833));
#15781=CARTESIAN_POINT('Ctrl Pts',(31.0669520428219,-0.750666938273188,
-0.681074536322006));
#15782=CARTESIAN_POINT('Ctrl Pts',(31.0482411755532,-0.90146749781528,-0.465863888580594));
#15783=CARTESIAN_POINT('Ctrl Pts',(31.0389957694103,-0.954288507126772,
-0.344674989241539));
#15784=CARTESIAN_POINT('Ctrl Pts',(31.0207107777182,-1.0084895405317,-0.0936168937762394));
#15785=CARTESIAN_POINT('Ctrl Pts',(31.0118846856426,-1.01254518840658,0.0325064994311476));
#15786=CARTESIAN_POINT('Ctrl Pts',(30.9929071645996,-0.972239729359772,
0.295767848335958));
#15787=CARTESIAN_POINT('Ctrl Pts',(30.9841478114738,-0.923830150460078,
0.411176385780254));
#15788=CARTESIAN_POINT('Ctrl Pts',(30.9766135577662,-0.870773359785341,
0.502739744071684));
#15789=CARTESIAN_POINT('',(31.1173426729392,-1.08229570837348,0.624863720382711));
#15790=CARTESIAN_POINT('',(31.1175,-1.082531754731,0.625));
#15791=CARTESIAN_POINT('Ctrl Pts',(31.1176143539202,-1.0821587115325,0.624802327952216));
#15792=CARTESIAN_POINT('Ctrl Pts',(31.1240060784292,-1.13782712827631,0.52886389959531));
#15793=CARTESIAN_POINT('Ctrl Pts',(31.1300982973054,-1.18011004660292,0.426676775976404));
#15794=CARTESIAN_POINT('Ctrl Pts',(31.1424052132346,-1.23534331762511,0.21651293345668));
#15795=CARTESIAN_POINT('Ctrl Pts',(31.1486181844907,-1.2490007937033,0.109811579967974));
#15796=CARTESIAN_POINT('Ctrl Pts',(31.1603920217383,-1.24950055350359,-0.0923920289202056));
#15797=CARTESIAN_POINT('Ctrl Pts',(31.1659562556459,-1.23898620331907,-0.188034416053155));
#15798=CARTESIAN_POINT('Ctrl Pts',(31.1772172324692,-1.19486152256834,-0.380931227675896));
#15799=CARTESIAN_POINT('Ctrl Pts',(31.1828002272484,-1.15990323431092,-0.476842290221254));
#15800=CARTESIAN_POINT('Ctrl Pts',(31.1933799224953,-1.07536359567061,-0.641674010671896));
#15801=CARTESIAN_POINT('Ctrl Pts',(31.1982004972963,-1.03015647433166,-0.711636089145887));
#15802=CARTESIAN_POINT('Ctrl Pts',(31.2086891642593,-0.918145662538923,
-0.852744715825088));
#15803=CARTESIAN_POINT('Ctrl Pts',(31.2143622631548,-0.848874078215494,
-0.922071107489431));
#15804=CARTESIAN_POINT('Ctrl Pts',(31.2258599403578,-0.690519777314687,
-1.04711607636139));
#15805=CARTESIAN_POINT('Ctrl Pts',(31.2315605712696,-0.601200097977752,
-1.10079838963472));
#15806=CARTESIAN_POINT('Ctrl Pts',(31.2422685234014,-0.429696982034391,
-1.17621321895925));
#15807=CARTESIAN_POINT('Ctrl Pts',(31.2470893694738,-0.350510236428935,
-1.20198149126957));
#15808=CARTESIAN_POINT('Ctrl Pts',(31.257554879535,-0.174979519772436,-1.24075076547737));
#15809=CARTESIAN_POINT('Ctrl Pts',(31.2632039529516,-0.0778867945370573,
-1.25086298378607));
#15810=CARTESIAN_POINT('Ctrl Pts',(31.2746485393151,0.123010454844053,-1.24821216732933));
#15811=CARTESIAN_POINT('Ctrl Pts',(31.280322861262,0.225730991441402,-1.23375161025498));
#15812=CARTESIAN_POINT('Ctrl Pts',(31.2910025371402,0.406028058762192,-1.18459423747141));
#15813=CARTESIAN_POINT('Ctrl Pts',(31.2958233857599,0.483792934919275,-1.15480128143035));
#15814=CARTESIAN_POINT('Ctrl Pts',(31.306290559336,0.644644376904782,-1.07448615399174));
#15815=CARTESIAN_POINT('Ctrl Pts',(31.3119413766805,0.726493363522555,-1.02124287488531));
#15816=CARTESIAN_POINT('Ctrl Pts',(31.3233905059103,0.88102312030248,-0.892733274001985));
#15817=CARTESIAN_POINT('Ctrl Pts',(31.3290672187261,0.951788897338445,-0.816826100609883));
#15818=CARTESIAN_POINT('Ctrl Pts',(31.3397493385164,1.06100281479554,-0.665128305607395));
#15819=CARTESIAN_POINT('Ctrl Pts',(31.3445701692346,1.10269161128873,-0.593037192331211));
#15820=CARTESIAN_POINT('Ctrl Pts',(31.3550382895877,1.17716691157256,-0.429381154761996));
#15821=CARTESIAN_POINT('Ctrl Pts',(31.3606900786588,1.20727587186345,-0.336478776281032));
#15822=CARTESIAN_POINT('Ctrl Pts',(31.3721410948635,1.24650146600664,-0.139327470567408));
#15823=CARTESIAN_POINT('Ctrl Pts',(31.3778186949677,1.25372629203966,-0.035786170497328));
#15824=CARTESIAN_POINT('Ctrl Pts',(31.3885018209641,1.24312755487409,0.150850910489866));
#15825=CARTESIAN_POINT('Ctrl Pts',(31.3933226590061,1.23015474858233,0.233110994982595));
#15826=CARTESIAN_POINT('Ctrl Pts',(31.4037902649713,1.18503744542128,0.407154197277295));
#15827=CARTESIAN_POINT('Ctrl Pts',(31.4094415234133,1.14997227807196,0.498292066471131));
#15828=CARTESIAN_POINT('Ctrl Pts',(31.4208914267738,1.05639139383983,0.676175349247458));
#15829=CARTESIAN_POINT('Ctrl Pts',(31.4265684855878,0.996851073617742,0.761180763904621));
#15830=CARTESIAN_POINT('Ctrl Pts',(31.4372510169724,0.871167832851708,0.899549283902962));
#15831=CARTESIAN_POINT('Ctrl Pts',(31.4420718532523,0.809318617397264,0.955314077686334));
#15832=CARTESIAN_POINT('Ctrl Pts',(31.4525396054238,0.664726021980267,1.0621808370084));
#15833=CARTESIAN_POINT('Ctrl Pts',(31.4581910150401,0.580118583972387,1.11094290951632));
#15834=CARTESIAN_POINT('Ctrl Pts',(31.4696412461842,0.395442457324174,1.19029483163864));
#15835=CARTESIAN_POINT('Ctrl Pts',(31.4753184665817,0.295672522154359,1.21888744119676));
#15836=CARTESIAN_POINT('Ctrl Pts',(31.4860011732024,0.110917242357187,1.24732498968612));
#15837=CARTESIAN_POINT('Ctrl Pts',(31.4908220096922,0.0277574696957337,
1.25173922866526));
#15838=CARTESIAN_POINT('Ctrl Pts',(31.5012897379625,-0.15186508887469,1.24379488711698));
#15839=CARTESIAN_POINT('Ctrl Pts',(31.5069411227735,-0.248303974134931,
1.22844486123761));
#15840=CARTESIAN_POINT('Ctrl Pts',(31.5183912843764,-0.441760912948824,
1.17389252414083));
#15841=CARTESIAN_POINT('Ctrl Pts',(31.5240684642586,-0.537289934727339,
1.13332616886551));
#15842=CARTESIAN_POINT('Ctrl Pts',(31.5347511268285,-0.698767508389034,
1.0391565055413));
#15843=CARTESIAN_POINT('Ctrl Pts',(31.5395719634338,-0.766172796318229,
0.990252910469221));
#15844=CARTESIAN_POINT('Ctrl Pts',(31.5500396974053,-0.900766349841046,
0.871038877426934));
#15845=CARTESIAN_POINT('Ctrl Pts',(31.5556910879605,-0.966053452853213,
0.7984186752522));
#15846=CARTESIAN_POINT('Ctrl Pts',(31.5671400108157,-1.08205433820025,0.634294972400312));
#15847=CARTESIAN_POINT('Ctrl Pts',(31.5728160323226,-1.13075742314166,0.542671102597745));
#15848=CARTESIAN_POINT('Ctrl Pts',(31.5834973753672,-1.1969878201771,0.367889849781088));
#15849=CARTESIAN_POINT('Ctrl Pts',(31.5883182192493,-1.2185997646116,0.287465667522941));
#15850=CARTESIAN_POINT('Ctrl Pts',(31.598786552775,-1.24818537041361,0.110107752503061));
#15851=CARTESIAN_POINT('Ctrl Pts',(31.6044385452042,-1.25322589302514,0.0125749161587526));
#15852=CARTESIAN_POINT('Ctrl Pts',(31.6159555432532,-1.24001667228593,-0.189166648342859));
#15853=CARTESIAN_POINT('Ctrl Pts',(31.6216943443875,-1.21983388555358,-0.292146062416069));
#15854=CARTESIAN_POINT('Ctrl Pts',(31.6324470241272,-1.16044909634215,-0.470588581982704));
#15855=CARTESIAN_POINT('Ctrl Pts',(31.6372674296349,-1.12643871032578,-0.546572117435137));
#15856=CARTESIAN_POINT('Ctrl Pts',(31.6468960985306,-1.04454265279206,-0.690254795732879));
#15857=CARTESIAN_POINT('Ctrl Pts',(31.6517073727424,-0.996655408805599,
-0.758051863175031));
#15858=CARTESIAN_POINT('Ctrl Pts',(31.6627702280804,-0.870203186990777,
-0.903984876539052));
#15859=CARTESIAN_POINT('Ctrl Pts',(31.6687898996599,-0.787576654254936,
-0.976889895296161));
#15860=CARTESIAN_POINT('Ctrl Pts',(31.6807821982022,-0.612473709547305,
-1.09370200728453));
#15861=CARTESIAN_POINT('Ctrl Pts',(31.6866153652929,-0.522536100534752,
-1.13912678752826));
#15862=CARTESIAN_POINT('Ctrl Pts',(31.6972573121406,-0.350845141361402,
-1.20189911231689));
#15863=CARTESIAN_POINT('Ctrl Pts',(31.7020725410413,-0.270255071154068,
-1.22276105030124));
#15864=CARTESIAN_POINT('Ctrl Pts',(31.7124537496761,-0.0904768146807791,
-1.25056862608197));
#15865=CARTESIAN_POINT('Ctrl Pts',(31.7178677208251,0.00831050603654517,
-1.25382693514982));
#15866=CARTESIAN_POINT('Ctrl Pts',(31.729120122559,0.205231055039715,-1.23651351800787));
#15867=CARTESIAN_POINT('Ctrl Pts',(31.7348690777854,0.302474923897132,-1.21611008967196));
#15868=CARTESIAN_POINT('Ctrl Pts',(31.7454278233989,0.474492182767166,-1.1586462038913));
#15869=CARTESIAN_POINT('Ctrl Pts',(31.750242280751,0.550446956570973,-1.12477176898818));
#15870=CARTESIAN_POINT('Ctrl Pts',(31.7608499067484,0.711610456908466,-1.03269615084912));
#15871=CARTESIAN_POINT('Ctrl Pts',(31.7664634133186,0.793642254012398,-0.971112508038292));
#15872=CARTESIAN_POINT('Ctrl Pts',(31.7779463101776,0.938547998489703,-0.83081467824553));
#15873=CARTESIAN_POINT('Ctrl Pts',(31.7837105565754,1.00135228378256,-0.753492673524034));
#15874=CARTESIAN_POINT('Ctrl Pts',(31.7942844843864,1.09879427128859,-0.600219979330559));
#15875=CARTESIAN_POINT('Ctrl Pts',(31.7990991412107,1.13640400067532,-0.526026457330732));
#15876=CARTESIAN_POINT('Ctrl Pts',(31.8096636675788,1.2031922306065,-0.353603390264143));
#15877=CARTESIAN_POINT('Ctrl Pts',(31.8152390244176,1.22794792049913,-0.254795958429211));
#15878=CARTESIAN_POINT('Ctrl Pts',(31.8266767980405,1.25221837372775,-0.0553556296855275));
#15879=CARTESIAN_POINT('Ctrl Pts',(31.8324371127675,1.25239511254884,0.0441936568360541));
#15880=CARTESIAN_POINT('Ctrl Pts',(31.8430071391335,1.23173787374873,0.224571567295447));
#15881=CARTESIAN_POINT('Ctrl Pts',(31.8478217466123,1.21430563356015,0.305901969734969));
#15882=CARTESIAN_POINT('Ctrl Pts',(31.8583971447548,1.15771387015253,0.482122034532278));
#15883=CARTESIAN_POINT('Ctrl Pts',(31.8639821116929,1.11471121147059,0.574659728153018));
#15884=CARTESIAN_POINT('Ctrl Pts',(31.8754311002046,1.00794890665499,0.745088064977724));
#15885=CARTESIAN_POINT('Ctrl Pts',(31.8811922595378,0.945424033184498,0.822570520864649));
#15886=CARTESIAN_POINT('Ctrl Pts',(31.8917631287764,0.815834206434843,0.949750247331783));
#15887=CARTESIAN_POINT('Ctrl Pts',(31.8965777506294,0.751099014735883,1.00198063352227));
#15888=CARTESIAN_POINT('Ctrl Pts',(31.9071510987955,0.596239547185957,1.10328359862058));
#15889=CARTESIAN_POINT('Ctrl Pts',(31.9127342708902,0.504612837395904,1.14811746123603));
#15890=CARTESIAN_POINT('Ctrl Pts',(31.9241816068141,0.31441684083408,1.21336736868684));
#15891=CARTESIAN_POINT('Ctrl Pts',(31.9299430459614,0.217059917363251,1.23423457381753));
#15892=CARTESIAN_POINT('Ctrl Pts',(31.940514178841,0.0363079555188546,1.25151630287605));
#15893=CARTESIAN_POINT('Ctrl Pts',(31.9453287907012,-0.0468705932600383,
1.25136661001164));
#15894=CARTESIAN_POINT('Ctrl Pts',(31.9559012836347,-0.230957182723031,
1.23263628126962));
#15895=CARTESIAN_POINT('Ctrl Pts',(31.9614836845859,-0.330365926848818,
1.20981945349652));
#15896=CARTESIAN_POINT('Ctrl Pts',(31.9729289302278,-0.519206939191319,
1.14084976837166));
#15897=CARTESIAN_POINT('Ctrl Pts',(31.9786890867423,-0.607981980552158,
1.09581189621577));
#15898=CARTESIAN_POINT('Ctrl Pts',(31.989258961414,-0.759316621509383,0.995514496023265));
#15899=CARTESIAN_POINT('Ctrl Pts',(31.9940735831732,-0.823867341779562,
0.943057378399203));
#15900=CARTESIAN_POINT('Ctrl Pts',(32.0046456557463,-0.955144999347304,
0.812668022846102));
#15901=CARTESIAN_POINT('Ctrl Pts',(32.0102275063711,-1.01804215831405,0.732388520580651));
#15902=CARTESIAN_POINT('Ctrl Pts',(32.0216724868892,-1.12141355965134,0.559953017256065));
#15903=CARTESIAN_POINT('Ctrl Pts',(32.0274331903612,-1.16207374523845,0.469074231388383));
#15904=CARTESIAN_POINT('Ctrl Pts',(32.0380037184577,-1.21657777222981,0.295881156004739));
#15905=CARTESIAN_POINT('Ctrl Pts',(32.0428183840667,-1.23373564079806,0.214493035986958));
#15906=CARTESIAN_POINT('Ctrl Pts',(32.053413281656,-1.25375520199998,0.0301660896758291));
#15907=CARTESIAN_POINT('Ctrl Pts',(32.0590165684404,-1.25206833167091,-0.0721904279698692));
#15908=CARTESIAN_POINT('Ctrl Pts',(32.0705013141532,-1.22362856901582,-0.271848294976713));
#15909=CARTESIAN_POINT('Ctrl Pts',(32.0762777295109,-1.19786641608811,-0.368269230476531));
#15910=CARTESIAN_POINT('Ctrl Pts',(32.086862971512,-1.13089974332563,-0.537309623191031));
#15911=CARTESIAN_POINT('Ctrl Pts',(32.0916772316598,-1.09290030489865,-0.611319008202032));
#15912=CARTESIAN_POINT('Ctrl Pts',(32.1021452017923,-0.993359558816285,
-0.76525346609263));
#15913=CARTESIAN_POINT('Ctrl Pts',(32.1076315891951,-0.92906785585012,-0.842177783760152));
#15914=CARTESIAN_POINT('Ctrl Pts',(32.118894750487,-0.7844446704897,-0.977499920442658));
#15915=CARTESIAN_POINT('Ctrl Pts',(32.1245780698579,-0.705266920519248,
-1.03574779176174));
#15916=CARTESIAN_POINT('Ctrl Pts',(32.136451253582,-0.528303136599548,-1.13705498101773));
#15917=CARTESIAN_POINT('Ctrl Pts',(32.1426442566818,-0.429344998410457,
-1.17836741706458));
#15918=CARTESIAN_POINT('Ctrl Pts',(32.1549206773639,-0.22019628775875,-1.23538794982945));
#15919=CARTESIAN_POINT('Ctrl Pts',(32.1610033640657,-0.110740339667427,
-1.24981720394665));
#15920=CARTESIAN_POINT('Ctrl Pts',(32.1673846094894,-2.65599045317292E-6,
-1.24957813805368));
#15921=CARTESIAN_POINT('Ctrl Pts',(32.36036289716,0.393685760654,-0.8842326957913));
#15922=CARTESIAN_POINT('Ctrl Pts',(32.34411289716,0.1930597260145,-0.9735571614325));
#15923=CARTESIAN_POINT('Ctrl Pts',(32.31161289716,-0.27049973535,-1.009904411168));
#15924=CARTESIAN_POINT('Ctrl Pts',(32.26286289716,-0.845926716811,-0.6145928909716));
#15925=CARTESIAN_POINT('Ctrl Pts',(32.21411289716,-1.044142703787,0.05472539254397));
#15926=CARTESIAN_POINT('Ctrl Pts',(32.16536289716,-0.7770226444626,0.6996312941492));
#15927=CARTESIAN_POINT('Ctrl Pts',(32.11661289716,-0.1635647789704,1.032711459003));
#15928=CARTESIAN_POINT('Ctrl Pts',(32.06786289716,0.5227918702356,0.905502289579));
#15929=CARTESIAN_POINT('Ctrl Pts',(32.01911289716,0.9761368603912,0.3747038366413));
#15930=CARTESIAN_POINT('Ctrl Pts',(31.97036289716,0.994409526335,-0.323103250189));
#15931=CARTESIAN_POINT('Ctrl Pts',(31.92161289716,0.5694658990877,-0.8769005799032));
#15932=CARTESIAN_POINT('Ctrl Pts',(31.87286289716,-0.109293296325,-1.039856246063));
#15933=CARTESIAN_POINT('Ctrl Pts',(31.82411289716,-0.7393395821542,-0.7393395822784));
#15934=CARTESIAN_POINT('Ctrl Pts',(31.77536289716,-1.039856245751,-0.1092932955163));
#15935=CARTESIAN_POINT('Ctrl Pts',(31.72661289716,-0.8769005812753,0.5694658959771));
#15936=CARTESIAN_POINT('Ctrl Pts',(31.67786289716,-0.3231032450128,0.9944095379687));
#15937=CARTESIAN_POINT('Ctrl Pts',(31.62911289716,0.3747038173086,0.9761368169669));
#15938=CARTESIAN_POINT('Ctrl Pts',(31.58036289716,0.9055023617337,0.5227920322988));
#15939=CARTESIAN_POINT('Ctrl Pts',(31.53161289716,1.032711189717,-0.1635653837993));
#15940=CARTESIAN_POINT('Ctrl Pts',(31.48286289716,0.69963229914,-0.7770203872106));
#15941=CARTESIAN_POINT('Ctrl Pts',(31.43411289716,0.05472164186737,-1.044151127966));
#15942=CARTESIAN_POINT('Ctrl Pts',(31.38536289716,-0.614578893256,-0.8458952773463));
#15943=CARTESIAN_POINT('Ctrl Pts',(31.33661289716,-1.009956651354,-0.2706170690297));
#15944=CARTESIAN_POINT('Ctrl Pts',(31.28786289716,-0.9551885735371,0.4252773519508));
#15945=CARTESIAN_POINT('Ctrl Pts',(31.23911289716,-0.4746852292457,0.9316222251505));
#15946=CARTESIAN_POINT('Ctrl Pts',(31.19036289716,0.2173891404585,1.022735536666));
#15947=CARTESIAN_POINT('Ctrl Pts',(31.14161289716,0.8125714716225,0.6580074003485));
#15948=CARTESIAN_POINT('Ctrl Pts',(31.09286289716,1.045583921078,-1.042735165158E-7));
#15949=CARTESIAN_POINT('Ctrl Pts',(31.04411289716,0.8125719687909,-0.6580069832544));
#15950=CARTESIAN_POINT('Ctrl Pts',(30.99536289716,0.2173871517845,-1.022736996495));
#15951=CARTESIAN_POINT('Ctrl Pts',(30.94661289716,-0.4746777717184,-0.9316168029278));
#15952=CARTESIAN_POINT('Ctrl Pts',(30.89786289716,-0.9552164149722,-0.4252975810124));
#15953=CARTESIAN_POINT('Ctrl Pts',(30.84911289716,-1.00985274314,0.2706925630538));
#15954=CARTESIAN_POINT('Ctrl Pts',(30.81661289716,-0.7465953708295,0.6539732078925));
#15955=CARTESIAN_POINT('Ctrl Pts',(30.80036289716,-0.568925097085,0.7830582177302));
#15956=CARTESIAN_POINT('Ctrl Pts',(32.29874545428,0.4370945424777,-0.9817304160777));
#15957=CARTESIAN_POINT('Ctrl Pts',(32.28249545428,0.2143469768198,-1.080904021891));
#15958=CARTESIAN_POINT('Ctrl Pts',(32.24999545428,-0.300325716294,-1.121259010771));
#15959=CARTESIAN_POINT('Ctrl Pts',(32.20124545428,-0.9392007235413,-0.6823594484165));
#15960=CARTESIAN_POINT('Ctrl Pts',(32.15249545428,-1.159272503621,0.06075955192329));
#15961=CARTESIAN_POINT('Ctrl Pts',(32.10374545428,-0.8626991149286,0.7767743997427));
#15962=CARTESIAN_POINT('Ctrl Pts',(32.05499545428,-0.1815998427547,1.146580821045));
#15963=CARTESIAN_POINT('Ctrl Pts',(32.00624545428,0.5804362163164,1.005345248755));
#15964=CARTESIAN_POINT('Ctrl Pts',(31.95749545428,1.083768164943,0.4160196237966));
#15965=CARTESIAN_POINT('Ctrl Pts',(31.90874545428,1.104055620977,-0.3587294269415));
#15966=CARTESIAN_POINT('Ctrl Pts',(31.85999545428,0.6322566409435,-0.9735898426565));
#15967=CARTESIAN_POINT('Ctrl Pts',(31.81124545428,-0.1213442499767,-1.154513410291));
#15968=CARTESIAN_POINT('Ctrl Pts',(31.76249545428,-0.8208610234226,-0.8208610235605));
#15969=CARTESIAN_POINT('Ctrl Pts',(31.71374545428,-1.154513409944,-0.1213442490788));
#15970=CARTESIAN_POINT('Ctrl Pts',(31.66499545428,-0.9735898441798,0.6322566374899));
#15971=CARTESIAN_POINT('Ctrl Pts',(31.61624545428,-0.3587294211945,1.104055633894));
#15972=CARTESIAN_POINT('Ctrl Pts',(31.56749545428,0.4160196023322,1.083768116731));
#15973=CARTESIAN_POINT('Ctrl Pts',(31.51874545428,1.005345328866,0.5804363962492));
#15974=CARTESIAN_POINT('Ctrl Pts',(31.46999545428,1.146580522067,-0.1816005142735));
#15975=CARTESIAN_POINT('Ctrl Pts',(31.42124545428,0.7767755155462,-0.8626966087863));
#15976=CARTESIAN_POINT('Ctrl Pts',(31.37249545428,0.06075538768766,-1.159281856671));
#15977=CARTESIAN_POINT('Ctrl Pts',(31.32374545428,-0.6823439072776,-0.9391658174822));
#15978=CARTESIAN_POINT('Ctrl Pts',(31.27499545428,-1.121317011091,-0.3004559874802));
#15979=CARTESIAN_POINT('Ctrl Pts',(31.22624545428,-1.06051006731,0.4721695020624));
#15980=CARTESIAN_POINT('Ctrl Pts',(31.17749545428,-0.5270252161353,1.034345234097));
#15981=CARTESIAN_POINT('Ctrl Pts',(31.12874545428,0.2413590136724,1.135504928428));
#15982=CARTESIAN_POINT('Ctrl Pts',(31.07999545428,0.9021676451524,0.7305609507554));
#15983=CARTESIAN_POINT('Ctrl Pts',(31.03124545428,1.160872633154,-1.157709766729E-7));
#15984=CARTESIAN_POINT('Ctrl Pts',(30.98249545428,0.9021681971399,-0.7305604876715));
#15985=CARTESIAN_POINT('Ctrl Pts',(30.93374545428,0.2413568057222,-1.135506549222));
#15986=CARTESIAN_POINT('Ctrl Pts',(30.88499545428,-0.5270169363223,-1.034339214006));
#15987=CARTESIAN_POINT('Ctrl Pts',(30.83624545428,-1.060540978612,-0.4721919616312));
#15988=CARTESIAN_POINT('Ctrl Pts',(30.78749545428,-1.121201645697,0.3005398056652));
#15989=CARTESIAN_POINT('Ctrl Pts',(30.75499545428,-0.8289168536006,0.7260819380959));
#15990=CARTESIAN_POINT('Ctrl Pts',(30.73874545428,-0.6316562087523,0.86940018568));
#15991=CARTESIAN_POINT('Ctrl Pts',(32.2371280114,0.4805033243013,-1.079228136364));
#15992=CARTESIAN_POINT('Ctrl Pts',(32.2208780114,0.2356342276251,-1.18825088235));
#15993=CARTESIAN_POINT('Ctrl Pts',(32.1883780114,-0.330151697238,-1.232613610374));
#15994=CARTESIAN_POINT('Ctrl Pts',(32.1396280114,-1.032474730272,-0.7501260058613));
#15995=CARTESIAN_POINT('Ctrl Pts',(32.0908780114,-1.274402303455,0.06679371130262));
#15996=CARTESIAN_POINT('Ctrl Pts',(32.0421280114,-0.9483755853946,0.8539175053361));
#15997=CARTESIAN_POINT('Ctrl Pts',(31.9933780114,-0.199634906539,1.260450183087));
#15998=CARTESIAN_POINT('Ctrl Pts',(31.9446280114,0.6380805623973,1.105188207931));
#15999=CARTESIAN_POINT('Ctrl Pts',(31.8958780114,1.191399469495,0.457335410952));
#16000=CARTESIAN_POINT('Ctrl Pts',(31.8471280114,1.21370171562,-0.3943556036939));
#16001=CARTESIAN_POINT('Ctrl Pts',(31.7983780114,0.6950473827993,-1.07027910541));
#16002=CARTESIAN_POINT('Ctrl Pts',(31.7496280114,-0.1333952036284,-1.269170574518));
#16003=CARTESIAN_POINT('Ctrl Pts',(31.7008780114,-0.902382464691,-0.9023824648425));
#16004=CARTESIAN_POINT('Ctrl Pts',(31.6521280114,-1.269170574137,-0.1333952026413));
#16005=CARTESIAN_POINT('Ctrl Pts',(31.6033780114,-1.070279107084,0.6950473790027));
#16006=CARTESIAN_POINT('Ctrl Pts',(31.5546280114,-0.3943555973762,1.213701729819));
#16007=CARTESIAN_POINT('Ctrl Pts',(31.5058780114,0.4573353873559,1.191399416495));
#16008=CARTESIAN_POINT('Ctrl Pts',(31.4571280114,1.105188295998,0.6380807601996));
#16009=CARTESIAN_POINT('Ctrl Pts',(31.4083780114,1.260449854417,-0.1996356447478));
#16010=CARTESIAN_POINT('Ctrl Pts',(31.3596280114,0.8539187319524,-0.948372830362));
#16011=CARTESIAN_POINT('Ctrl Pts',(31.3108780114,0.06678913350795,-1.274412585376));
#16012=CARTESIAN_POINT('Ctrl Pts',(31.2621280114,-0.7501089212991,-1.032436357618));
#16013=CARTESIAN_POINT('Ctrl Pts',(31.2133780114,-1.232677370829,-0.3302949059307));
#16014=CARTESIAN_POINT('Ctrl Pts',(31.1646280114,-1.165831561083,0.519061652174));
#16015=CARTESIAN_POINT('Ctrl Pts',(31.1158780114,-0.5793652030249,1.137068243043));
#16016=CARTESIAN_POINT('Ctrl Pts',(31.0671280114,0.2653288868863,1.248274320191));
#16017=CARTESIAN_POINT('Ctrl Pts',(31.0183780114,0.9917638186823,0.8031145011624));
#16018=CARTESIAN_POINT('Ctrl Pts',(30.9696280114,1.27616134523,-1.272684367085E-7));
#16019=CARTESIAN_POINT('Ctrl Pts',(30.9208780114,0.9917644254889,-0.8031139920886));
#16020=CARTESIAN_POINT('Ctrl Pts',(30.8721280114,0.26532645966,-1.248276101949));
#16021=CARTESIAN_POINT('Ctrl Pts',(30.8233780114,-0.5793561009262,-1.137061625084));
#16022=CARTESIAN_POINT('Ctrl Pts',(30.7746280114,-1.165865542251,-0.5190863422501));
#16023=CARTESIAN_POINT('Ctrl Pts',(30.7258780114,-1.232550548254,0.3303870482766));
#16024=CARTESIAN_POINT('Ctrl Pts',(30.6933780114,-0.9112383363718,0.7981906682994));
#16025=CARTESIAN_POINT('Ctrl Pts',(30.6771280114,-0.6943873204195,0.9557421536299));
#16026=CARTESIAN_POINT('Ctrl Pts',(32.17551056852,0.523912106125,-1.17672585665));
#16027=CARTESIAN_POINT('Ctrl Pts',(32.15926056852,0.2569214784303,-1.295597742809));
#16028=CARTESIAN_POINT('Ctrl Pts',(32.12676056852,-0.3599776781819,-1.343968209978));
#16029=CARTESIAN_POINT('Ctrl Pts',(32.07801056852,-1.125748737002,-0.8178925633062));
#16030=CARTESIAN_POINT('Ctrl Pts',(32.02926056852,-1.389532103288,0.07282787068194));
#16031=CARTESIAN_POINT('Ctrl Pts',(31.98051056852,-1.034052055861,0.9310606109295));
#16032=CARTESIAN_POINT('Ctrl Pts',(31.93176056852,-0.2176699703234,1.374319545129));
#16033=CARTESIAN_POINT('Ctrl Pts',(31.88301056852,0.6957249084782,1.205031167107));
#16034=CARTESIAN_POINT('Ctrl Pts',(31.83426056852,1.299030774048,0.4986511981073));
#16035=CARTESIAN_POINT('Ctrl Pts',(31.78551056852,1.323347810262,-0.4299817804464));
#16036=CARTESIAN_POINT('Ctrl Pts',(31.73676056852,0.7578381246551,-1.166968368163));
#16037=CARTESIAN_POINT('Ctrl Pts',(31.68801056852,-0.14544615728,-1.383827738746));
#16038=CARTESIAN_POINT('Ctrl Pts',(31.63926056852,-0.9839039059594,-0.9839039061246));
#16039=CARTESIAN_POINT('Ctrl Pts',(31.59051056852,-1.383827738331,-0.1454461562038));
#16040=CARTESIAN_POINT('Ctrl Pts',(31.54176056852,-1.166968369989,0.7578381205155));
#16041=CARTESIAN_POINT('Ctrl Pts',(31.49301056852,-0.4299817735579,1.323347825744));
#16042=CARTESIAN_POINT('Ctrl Pts',(31.44426056852,0.4986511723795,1.299030716259));
#16043=CARTESIAN_POINT('Ctrl Pts',(31.39551056852,1.20503126313,0.69572512415));
#16044=CARTESIAN_POINT('Ctrl Pts',(31.34676056852,1.374319186766,-0.217670775222));
#16045=CARTESIAN_POINT('Ctrl Pts',(31.29801056852,0.9310619483586,-1.034049051938));
#16046=CARTESIAN_POINT('Ctrl Pts',(31.24926056852,0.07282287932824,-1.389543314081));
#16047=CARTESIAN_POINT('Ctrl Pts',(31.20051056852,-0.8178739353206,-1.125706897754));
#16048=CARTESIAN_POINT('Ctrl Pts',(31.15176056852,-1.344037730566,-0.3601338243812));
#16049=CARTESIAN_POINT('Ctrl Pts',(31.10301056852,-1.271153054855,0.5659538022856));
#16050=CARTESIAN_POINT('Ctrl Pts',(31.05426056852,-0.6317051899145,1.239791251989));
#16051=CARTESIAN_POINT('Ctrl Pts',(31.00551056852,0.2892987601002,1.361043711953));
#16052=CARTESIAN_POINT('Ctrl Pts',(30.95676056852,1.081359992212,0.8756680515693));
#16053=CARTESIAN_POINT('Ctrl Pts',(30.90801056852,1.391450057306,-1.387658968566E-7));
#16054=CARTESIAN_POINT('Ctrl Pts',(30.85926056852,1.081360653838,-0.8756674965057));
#16055=CARTESIAN_POINT('Ctrl Pts',(30.81051056852,0.2892961135977,-1.361045654676));
#16056=CARTESIAN_POINT('Ctrl Pts',(30.76176056852,-0.6316952655301,-1.239784036163));
#16057=CARTESIAN_POINT('Ctrl Pts',(30.71301056852,-1.271190105891,-0.5659807228689));
#16058=CARTESIAN_POINT('Ctrl Pts',(30.66426056852,-1.34389945081,0.360234290888));
#16059=CARTESIAN_POINT('Ctrl Pts',(30.63176056852,-0.9935598191429,0.8702993985029));
#16060=CARTESIAN_POINT('Ctrl Pts',(30.61551056852,-0.7571184320868,1.04208412158));
#16061=CARTESIAN_POINT('',(30.6676573270714,-1.08229570995281,0.624863717659191));
#16062=CARTESIAN_POINT('Ctrl Pts',(31.1176273419681,-1.08213858864712,0.62479197410143));
#16063=CARTESIAN_POINT('Ctrl Pts',(31.1107147429913,-1.02303331417979,0.727024583856292));
#16064=CARTESIAN_POINT('Ctrl Pts',(31.1036652880828,-0.949354002246978,
0.821167118675191));
#16065=CARTESIAN_POINT('Ctrl Pts',(31.0914707967952,-0.793986411015714,
0.96976959435426));
#16066=CARTESIAN_POINT('Ctrl Pts',(31.0861831561242,-0.716601260523713,
1.02825175920507));
#16067=CARTESIAN_POINT('Ctrl Pts',(31.074597198985,-0.539033774835006,1.1326861784073));
#16068=CARTESIAN_POINT('Ctrl Pts',(31.0681881308309,-0.437716166441462,
1.17534812713065));
#16069=CARTESIAN_POINT('Ctrl Pts',(31.0562672659825,-0.24255605393822,1.22931251285163));
#16070=CARTESIAN_POINT('Ctrl Pts',(31.0508051636701,-0.149571656505103,
1.24420676722394));
#16071=CARTESIAN_POINT('Ctrl Pts',(31.0418623888304,0.00919625518616045,
1.2512800440883));
#16072=CARTESIAN_POINT('Ctrl Pts',(31.0382746672938,0.0741691752309933,
1.24910986516245));
#16073=CARTESIAN_POINT('Ctrl Pts',(31.0251896685361,0.306806851999765,1.22316153355839));
#16074=CARTESIAN_POINT('Ctrl Pts',(31.016360185823,0.449029898248617,1.17281102777512));
#16075=CARTESIAN_POINT('Ctrl Pts',(30.99912749308,0.711896397089818,1.04065123262023));
#16076=CARTESIAN_POINT('Ctrl Pts',(30.9909450788194,0.82899352376291,0.944182238937826));
#16077=CARTESIAN_POINT('Ctrl Pts',(30.9774634344618,0.991793696766178,0.767975237832159));
#16078=CARTESIAN_POINT('Ctrl Pts',(30.9711100347715,1.05467900915692,0.678676212367285));
#16079=CARTESIAN_POINT('Ctrl Pts',(30.959202210651,1.14908717222668,0.499730244100428));
#16080=CARTESIAN_POINT('Ctrl Pts',(30.9537007807284,1.18369135429807,0.411566765861706));
#16081=CARTESIAN_POINT('Ctrl Pts',(30.9438229027414,1.22863151928554,0.242012696805622));
#16082=CARTESIAN_POINT('Ctrl Pts',(30.9393693749073,1.24172722685384,0.161905228300936));
#16083=CARTESIAN_POINT('Ctrl Pts',(30.928625116135,1.25416164465956,-0.028878966128762));
#16084=CARTESIAN_POINT('Ctrl Pts',(30.9221845557975,1.24653514576959,-0.139280723297152));
#16085=CARTESIAN_POINT('Ctrl Pts',(30.9104528390688,1.20718822105003,-0.33471427577669));
#16086=CARTESIAN_POINT('Ctrl Pts',(30.9052034580452,1.180076443489,-0.42084528229441));
#16087=CARTESIAN_POINT('Ctrl Pts',(30.897142254913,1.12250736390062,-0.551664921075211));
#16088=CARTESIAN_POINT('Ctrl Pts',(30.8942079540235,1.09821626001909,-0.598579294719281));
#16089=CARTESIAN_POINT('Ctrl Pts',(30.8870456269382,1.0319671908342,-0.708770188829124));
#16090=CARTESIAN_POINT('Ctrl Pts',(30.8828141613499,0.987150554639301,-0.769988214526295));
#16091=CARTESIAN_POINT('Ctrl Pts',(30.8740840162147,0.887207752238275,-0.883080681038765));
#16092=CARTESIAN_POINT('Ctrl Pts',(30.8696447196692,0.832425385282746,-0.934834990540918));
#16093=CARTESIAN_POINT('Ctrl Pts',(30.8549499340359,0.636142316174003,-1.08965651088435));
#16094=CARTESIAN_POINT('Ctrl Pts',(30.8460582886474,0.488207161417728,-1.15990237222862));
#16095=CARTESIAN_POINT('Ctrl Pts',(30.8310695387291,0.231609455004719,-1.23364856654246));
#16096=CARTESIAN_POINT('Ctrl Pts',(30.8241653576879,0.114175065965537,-1.24976891671705));
#16097=CARTESIAN_POINT('Ctrl Pts',(30.8117487577039,-0.0969174534092562,
-1.24928985471921));
#16098=CARTESIAN_POINT('Ctrl Pts',(30.8063060980654,-0.190566114444294,
-1.23860282577024));
#16099=CARTESIAN_POINT('Ctrl Pts',(30.7964788123334,-0.361099480681787,
-1.1990421161748));
#16100=CARTESIAN_POINT('Ctrl Pts',(30.7920242842892,-0.438035516948806,
-1.17312939535201));
#16101=CARTESIAN_POINT('Ctrl Pts',(30.7821347361325,-0.598054952684592,
-1.10128766414562));
#16102=CARTESIAN_POINT('Ctrl Pts',(30.7766219444153,-0.679463409247483,
-1.05282931385649));
#16103=CARTESIAN_POINT('Ctrl Pts',(30.7645953465248,-0.842366488971656,
-0.929432657525112));
#16104=CARTESIAN_POINT('Ctrl Pts',(30.7581474996506,-0.921522622038355,
-0.851300688675754));
#16105=CARTESIAN_POINT('Ctrl Pts',(30.7473757956398,-1.03884531089792,-0.699249054330331));
#16106=CARTESIAN_POINT('Ctrl Pts',(30.7429074217849,-1.08209144506206,-0.630271416060541));
#16107=CARTESIAN_POINT('Ctrl Pts',(30.7330205452947,-1.16020648864805,-0.473609586532843));
#16108=CARTESIAN_POINT('Ctrl Pts',(30.7275265553958,-1.19235173606669,-0.385071099146812));
#16109=CARTESIAN_POINT('Ctrl Pts',(30.7159283777517,-1.23871500251242,-0.193658268460273));
#16110=CARTESIAN_POINT('Ctrl Pts',(30.7098661712449,-1.25070029183962,-0.0900484640374073));
#16111=CARTESIAN_POINT('Ctrl Pts',(30.6953712902796,-1.24780339486507,0.167826800855185));
#16112=CARTESIAN_POINT('Ctrl Pts',(30.6862525691742,-1.21748631584923,0.333552517175049));
#16113=CARTESIAN_POINT('Ctrl Pts',(30.6729396636004,-1.12715505203218,0.541344630190737));
#16114=CARTESIAN_POINT('Ctrl Pts',(30.6701455790125,-1.10581562102616,0.58372568895839));
#16115=CARTESIAN_POINT('Ctrl Pts',(30.6673726659358,-1.08215508341737,0.62476340416037));
#16116=CARTESIAN_POINT('',(30.8083734681527,-0.871221485874862,0.502999959144598));
#16117=CARTESIAN_POINT('',(30.80837346568,-0.8712215562071,0.503));
#16118=CARTESIAN_POINT('Ctrl Pts',(32.3083865340664,-1.74310513141563E-10,
-1.00548172051402));
#16119=CARTESIAN_POINT('Ctrl Pts',(32.3008522416291,-0.105825134387246,
-1.00564870423719));
#16120=CARTESIAN_POINT('Ctrl Pts',(32.292092822766,-0.229977637746814,-0.989868369579392));
#16121=CARTESIAN_POINT('Ctrl Pts',(32.2731152412578,-0.478122027735569,
-0.89314255386251));
#16122=CARTESIAN_POINT('Ctrl Pts',(32.2642891857646,-0.585319758593422,
-0.82656877022494));
#16123=CARTESIAN_POINT('Ctrl Pts',(32.2460042305897,-0.775641550295093,
-0.654100595091272));
#16124=CARTESIAN_POINT('Ctrl Pts',(32.2367588244469,-0.854183711123656,
-0.547761809504565));
#16125=CARTESIAN_POINT('Ctrl Pts',(32.2180479571783,-0.96516131946172,-0.309559370165468));
#16126=CARTESIAN_POINT('Ctrl Pts',(32.2088151157516,-0.997469062168773,
-0.18135349972004));
#16127=CARTESIAN_POINT('Ctrl Pts',(32.1886171121706,-1.01283629382345,0.101717750507548));
#16128=CARTESIAN_POINT('Ctrl Pts',(32.1792516786673,-0.984367566826269,
0.232947114591695));
#16129=CARTESIAN_POINT('Ctrl Pts',(32.1624059009715,-0.904804400397712,
0.455893933067162));
#16130=CARTESIAN_POINT('Ctrl Pts',(32.1534069464232,-0.8403008713478,0.567222034592228));
#16131=CARTESIAN_POINT('Ctrl Pts',(32.1342989682696,-0.663919325666452,
0.769080055430524));
#16132=CARTESIAN_POINT('Ctrl Pts',(32.1247947693777,-0.553320416471879,
0.848600935605247));
#16133=CARTESIAN_POINT('Ctrl Pts',(32.1082077163491,-0.343914891685575,
0.950970008765684));
#16134=CARTESIAN_POINT('Ctrl Pts',(32.0990210738252,-0.219359775122022,
0.993525782886267));
#16135=CARTESIAN_POINT('Ctrl Pts',(32.0788719338334,0.0627872995112449,
1.01225002509461));
#16136=CARTESIAN_POINT('Ctrl Pts',(32.0694606001008,0.196496573752336,0.99465935166052));
#16137=CARTESIAN_POINT('Ctrl Pts',(32.0505675506108,0.448119147312173,0.910386233646103));
#16138=CARTESIAN_POINT('Ctrl Pts',(32.0413142276786,0.562777737133885,0.844344677318304));
#16139=CARTESIAN_POINT('Ctrl Pts',(32.022610619119,0.75989433170913,0.670695233562689));
#16140=CARTESIAN_POINT('Ctrl Pts',(32.0133914653588,0.840830374658887,0.566410881442958));
#16141=CARTESIAN_POINT('Ctrl Pts',(31.9931854475348,0.968593109628251,0.313236296615739));
#16142=CARTESIAN_POINT('Ctrl Pts',(31.9838067366341,0.995103645636241,0.181385312576401));
#16143=CARTESIAN_POINT('Ctrl Pts',(31.9670009367567,1.01170308102003,-0.0541913934911888));
#16144=CARTESIAN_POINT('Ctrl Pts',(31.9580168824801,0.997390470348591,-0.181830481509643));
#16145=CARTESIAN_POINT('Ctrl Pts',(31.9394916971386,0.919423226898875,-0.429745166292926));
#16146=CARTESIAN_POINT('Ctrl Pts',(31.9299862507461,0.852869094566032,-0.548542238822891));
#16147=CARTESIAN_POINT('Ctrl Pts',(31.9128021772271,0.696891195219597,-0.732880461232638));
#16148=CARTESIAN_POINT('Ctrl Pts',(31.9036116032874,0.599816161628682,-0.82184250904315));
#16149=CARTESIAN_POINT('Ctrl Pts',(31.8834719027534,0.349028087285575,-0.952204354992635));
#16150=CARTESIAN_POINT('Ctrl Pts',(31.87406864958,0.219635000613414,-0.989799618535099));
#16151=CARTESIAN_POINT('Ctrl Pts',(31.8551692839622,-0.0447199889143614,
-1.01375940902338));
#16152=CARTESIAN_POINT('Ctrl Pts',(31.8459048150744,-0.176402393566575,
-0.999237404326071));
#16153=CARTESIAN_POINT('Ctrl Pts',(31.8272137745116,-0.426500714921257,
-0.919407894705326));
#16154=CARTESIAN_POINT('Ctrl Pts',(31.8180068956466,-0.54236453935169,-0.856538059210491));
#16155=CARTESIAN_POINT('Ctrl Pts',(31.7977899305543,-0.76122046743556,-0.675972386498982));
#16156=CARTESIAN_POINT('Ctrl Pts',(31.7883977032762,-0.83849377181371,-0.565639342750775));
#16157=CARTESIAN_POINT('Ctrl Pts',(31.7716308252545,-0.948125656391319,
-0.357081831558923));
#16158=CARTESIAN_POINT('Ctrl Pts',(31.7626606378466,-0.986297530771064,
-0.234667590561064));
#16159=CARTESIAN_POINT('Ctrl Pts',(31.7441622029207,-1.01458386847578,0.023295661735769));
#16160=CARTESIAN_POINT('Ctrl Pts',(31.7346587869633,-1.00153559313095,0.158814096445749));
#16161=CARTESIAN_POINT('Ctrl Pts',(31.7174342420197,-0.932797546195441,
0.390887587624608));
#16162=CARTESIAN_POINT('Ctrl Pts',(31.7082400320689,-0.879593330129108,
0.511383216351974));
#16163=CARTESIAN_POINT('Ctrl Pts',(31.6881085385382,-0.702418860402563,
0.731471621586348));
#16164=CARTESIAN_POINT('Ctrl Pts',(31.6787128604578,-0.599170684072249,
0.817877985664102));
#16165=CARTESIAN_POINT('Ctrl Pts',(31.6598090757102,-0.366747863090086,
0.94619487811632));
#16166=CARTESIAN_POINT('Ctrl Pts',(31.6505332144177,-0.240163206787929,
0.985835062226094));
#16167=CARTESIAN_POINT('Ctrl Pts',(31.631854735458,0.0207603676707009,1.01327765451514));
#16168=CARTESIAN_POINT('Ctrl Pts',(31.6226591218942,0.151958878920123,1.00235989692945));
#16169=CARTESIAN_POINT('Ctrl Pts',(31.6024311543349,0.425111210006055,0.925080808596332));
#16170=CARTESIAN_POINT('Ctrl Pts',(31.5930263688461,0.540347644379315,0.854950472866657));
#16171=CARTESIAN_POINT('Ctrl Pts',(31.5762958650647,0.724235313103979,0.708453750739638));
#16172=CARTESIAN_POINT('Ctrl Pts',(31.5673383109915,0.808338952205112,0.61191586504363));
#16173=CARTESIAN_POINT('Ctrl Pts',(31.5494086203685,0.934104160209125,0.394084134956314));
#16174=CARTESIAN_POINT('Ctrl Pts',(31.5404510663023,0.975656602098998,0.272979304096006));
#16175=CARTESIAN_POINT('Ctrl Pts',(31.5237205625209,1.01058265066987,0.0404795504743948));
#16176=CARTESIAN_POINT('Ctrl Pts',(31.5143157770322,1.01369908580113,-0.0943832969990423));
#16177=CARTESIAN_POINT('Ctrl Pts',(31.4940878094729,0.944048573936176,-0.36957969898848));
#16178=CARTESIAN_POINT('Ctrl Pts',(31.484892195909,0.887904373733185,-0.488659821461784));
#16179=CARTESIAN_POINT('Ctrl Pts',(31.4662137169492,0.733676604436153,-0.700904969244634));
#16180=CARTESIAN_POINT('Ctrl Pts',(31.4569378556567,0.636054869835301,-0.790710405276939));
#16181=CARTESIAN_POINT('Ctrl Pts',(31.438034070909,0.408717770745871,-0.927836026440972));
#16182=CARTESIAN_POINT('Ctrl Pts',(31.4286383928287,0.282263576240673,-0.974048387998727));
#16183=CARTESIAN_POINT('Ctrl Pts',(31.408506899298,0.0030741913658229,-1.01744177706707));
#16184=CARTESIAN_POINT('Ctrl Pts',(31.3993126893472,-0.127880192190337,
-1.00327016540538));
#16185=CARTESIAN_POINT('Ctrl Pts',(31.3820881444036,-0.363230754564014,
-0.946762314668811));
#16186=CARTESIAN_POINT('Ctrl Pts',(31.3725847284462,-0.487117299376376,
-0.890303235238137));
#16187=CARTESIAN_POINT('Ctrl Pts',(31.3540862935205,-0.696376860255659,
-0.736824922057744));
#16188=CARTESIAN_POINT('Ctrl Pts',(31.3451161061127,-0.783304765554694,
-0.642559988636201));
#16189=CARTESIAN_POINT('Ctrl Pts',(31.328349228091,-0.909104926108205,-0.443337235931508));
#16190=CARTESIAN_POINT('Ctrl Pts',(31.318957000813,-0.966019492682176,-0.321250069431278));
#16191=CARTESIAN_POINT('Ctrl Pts',(31.2987400357208,-1.01296598826022,-0.0414324395852903));
#16192=CARTESIAN_POINT('Ctrl Pts',(31.2895331568557,-1.00948095071539,0.0903434934989204));
#16193=CARTESIAN_POINT('Ctrl Pts',(31.2708421162928,-0.953566173341271,
0.346849748046566));
#16194=CARTESIAN_POINT('Ctrl Pts',(31.261577647405,-0.900301395996995,0.468151058055271));
#16195=CARTESIAN_POINT('Ctrl Pts',(31.2426782817871,-0.74737411400106,0.685109299359031));
#16196=CARTESIAN_POINT('Ctrl Pts',(31.2332750286137,-0.650119117375376,
0.778369367719788));
#16197=CARTESIAN_POINT('Ctrl Pts',(31.2131353280796,-0.411828409927442,
0.930377288092374));
#16198=CARTESIAN_POINT('Ctrl Pts',(31.20394475414,-0.286247499755294,0.969965709350153));
#16199=CARTESIAN_POINT('Ctrl Pts',(31.1867606806209,-0.048616966586575,
1.01287742140833));
#16200=CARTESIAN_POINT('Ctrl Pts',(31.1772552342285,0.0875413822861211,
1.01111645447045));
#16201=CARTESIAN_POINT('Ctrl Pts',(31.158730048887,0.341225419004663,0.954680725569337));
#16202=CARTESIAN_POINT('Ctrl Pts',(31.1497459946104,0.458920417080296,0.903256265996058));
#16203=CARTESIAN_POINT('Ctrl Pts',(31.132940194733,0.654636111382746,0.771092380231476));
#16204=CARTESIAN_POINT('Ctrl Pts',(31.1235614838323,0.755567145070688,0.682208090561055));
#16205=CARTESIAN_POINT('Ctrl Pts',(31.1033554660083,0.910941399638799,0.444975024007267));
#16206=CARTESIAN_POINT('Ctrl Pts',(31.094136312248,0.960786276316762,0.322740178671249));
#16207=CARTESIAN_POINT('Ctrl Pts',(31.0754327036884,1.0126128086746,0.0652074783839158));
#16208=CARTESIAN_POINT('Ctrl Pts',(31.0661793807561,1.01247717924913,-0.0671105513277207));
#16209=CARTESIAN_POINT('Ctrl Pts',(31.0472863312659,0.959648553525886,-0.327158651203511));
#16210=CARTESIAN_POINT('Ctrl Pts',(31.0378749975333,0.908027886468954,-0.451749616134993));
#16211=CARTESIAN_POINT('Ctrl Pts',(31.0177258575413,0.750738679733226,-0.686734029267063));
#16212=CARTESIAN_POINT('Ctrl Pts',(31.0085392150175,0.651606739985195,-0.773324037322341));
#16213=CARTESIAN_POINT('Ctrl Pts',(30.9919521619889,0.458249759673328,-0.903490004899922));
#16214=CARTESIAN_POINT('Ctrl Pts',(30.9824479630971,0.334083202713453,-0.959511029806077));
#16215=CARTESIAN_POINT('Ctrl Pts',(30.9633399849436,0.0710782558689305,
-1.0113329187058));
#16216=CARTESIAN_POINT('Ctrl Pts',(30.9543410303954,-0.0575864727317485,
-1.01153056273425));
#16217=CARTESIAN_POINT('Ctrl Pts',(30.9374952526997,-0.290445664438498,
-0.968960876829235));
#16218=CARTESIAN_POINT('Ctrl Pts',(30.9281298191965,-0.418327990956307,
-0.928000835580185));
#16219=CARTESIAN_POINT('Ctrl Pts',(30.9079318156155,-0.655791268906815,
-0.773156797467811));
#16220=CARTESIAN_POINT('Ctrl Pts',(30.8986989741888,-0.750666938273209,
-0.681074536321982));
#16221=CARTESIAN_POINT('Ctrl Pts',(30.8799881069201,-0.901467497815293,
-0.465863888580567));
#16222=CARTESIAN_POINT('Ctrl Pts',(30.8707427007773,-0.954288507126781,
-0.344674989241513));
#16223=CARTESIAN_POINT('Ctrl Pts',(30.8524577090853,-1.00848954053165,-0.0936168937764534));
#16224=CARTESIAN_POINT('Ctrl Pts',(30.8436316170097,-1.01254518840657,0.0325064994306721));
#16225=CARTESIAN_POINT('Ctrl Pts',(30.8246540986637,-0.972239735087881,
0.295767810922606));
#16226=CARTESIAN_POINT('Ctrl Pts',(30.8158947475416,-0.923830175985573,
0.411176324318523));
#16227=CARTESIAN_POINT('Ctrl Pts',(30.8083604951405,-0.870773402088998,
0.502739671065661));
#16228=CARTESIAN_POINT('Ctrl Pts',(32.55060539727,0.4091770629343,-0.9190267303885));
#16229=CARTESIAN_POINT('Ctrl Pts',(32.53435539727,0.2006565122657,-1.011866061022));
#16230=CARTESIAN_POINT('Ctrl Pts',(32.50185539727,-0.2811437402541,-1.049643553578));
#16231=CARTESIAN_POINT('Ctrl Pts',(32.45310539727,-0.8792134337482,-0.6387767584235));
#16232=CARTESIAN_POINT('Ctrl Pts',(32.40435539727,-1.0852291028,0.05687880443496));
#16233=CARTESIAN_POINT('Ctrl Pts',(32.35560539727,-0.8075980268285,0.7271613725661));
#16234=CARTESIAN_POINT('Ctrl Pts',(32.30685539727,-0.170000956467,1.073348045283));
#16235=CARTESIAN_POINT('Ctrl Pts',(32.25810539727,0.5433634217137,0.9411332701358));
#16236=CARTESIAN_POINT('Ctrl Pts',(32.20935539727,1.014547269612,0.3894482114171));
#16237=CARTESIAN_POINT('Ctrl Pts',(32.16060539727,1.033538954174,-0.3358171723489));
#16238=CARTESIAN_POINT('Ctrl Pts',(32.11185539727,0.5918740460484,-0.9114061000685));
#16239=CARTESIAN_POINT('Ctrl Pts',(32.06310539727,-0.1135939230171,-1.080773975495));
#16240=CARTESIAN_POINT('Ctrl Pts',(32.01435539727,-0.7684321582634,-0.7684321583925));
#16241=CARTESIAN_POINT('Ctrl Pts',(31.96560539727,-1.080773975171,-0.1135939221766));
#16242=CARTESIAN_POINT('Ctrl Pts',(31.91685539727,-0.9114061014946,0.5918740428154));
#16243=CARTESIAN_POINT('Ctrl Pts',(31.86810539727,-0.3358171669691,1.033538966266));
#16244=CARTESIAN_POINT('Ctrl Pts',(31.81935539727,0.3894481913237,1.014547224479));
#16245=CARTESIAN_POINT('Ctrl Pts',(31.77060539727,0.9411333451298,0.543363590154));
#16246=CARTESIAN_POINT('Ctrl Pts',(31.72185539727,1.0733477654,-0.1700015850955));
#16247=CARTESIAN_POINT('Ctrl Pts',(31.67310539727,0.7271624171027,-0.807595680755));
#16248=CARTESIAN_POINT('Ctrl Pts',(31.62435539727,0.05687490617145,-1.085237858466));
#16249=CARTESIAN_POINT('Ctrl Pts',(31.57560539727,-0.6387622099061,-0.8791807571591));
#16250=CARTESIAN_POINT('Ctrl Pts',(31.52685539727,-1.049697849384,-0.2812656909448));
#16251=CARTESIAN_POINT('Ctrl Pts',(31.47810539727,-0.9927746800367,0.4420117646994));
#16252=CARTESIAN_POINT('Ctrl Pts',(31.42935539727,-0.4933638127992,0.9682810097529));
#16253=CARTESIAN_POINT('Ctrl Pts',(31.38060539727,0.2259432748059,1.06297957629));
#16254=CARTESIAN_POINT('Ctrl Pts',(31.33185539727,0.8445456793518,0.6838996031158));
#16255=CARTESIAN_POINT('Ctrl Pts',(31.28310539727,1.086727031141,-1.083766177912E-7));
#16256=CARTESIAN_POINT('Ctrl Pts',(31.23435539727,0.8445461960836,-0.6838991696094));
#16257=CARTESIAN_POINT('Ctrl Pts',(31.18560539727,0.2259412078788,-1.062981093563));
#16258=CARTESIAN_POINT('Ctrl Pts',(31.13685539727,-0.4933560618227,-0.9682753741689));
#16259=CARTESIAN_POINT('Ctrl Pts',(31.08810539727,-0.9928036170159,-0.4420327897627));
#16260=CARTESIAN_POINT('Ctrl Pts',(31.03935539727,-1.049589852444,0.2813441556141));
#16261=CARTESIAN_POINT('Ctrl Pts',(31.00685539727,-0.7759734579398,0.6797066675681));
#16262=CARTESIAN_POINT('Ctrl Pts',(30.99060539727,-0.5913119638062,0.8138710963412));
#16263=CARTESIAN_POINT('Ctrl Pts',(32.46520179909,0.4091770629343,-0.9190267303885));
#16264=CARTESIAN_POINT('Ctrl Pts',(32.44895179909,0.2006565122657,-1.011866061022));
#16265=CARTESIAN_POINT('Ctrl Pts',(32.41645179909,-0.2811437402541,-1.049643553578));
#16266=CARTESIAN_POINT('Ctrl Pts',(32.36770179909,-0.8792134337482,-0.6387767584235));
#16267=CARTESIAN_POINT('Ctrl Pts',(32.31895179909,-1.0852291028,0.05687880443496));
#16268=CARTESIAN_POINT('Ctrl Pts',(32.27020179909,-0.8075980268285,0.7271613725661));
#16269=CARTESIAN_POINT('Ctrl Pts',(32.22145179909,-0.170000956467,1.073348045283));
#16270=CARTESIAN_POINT('Ctrl Pts',(32.17270179909,0.5433634217137,0.9411332701358));
#16271=CARTESIAN_POINT('Ctrl Pts',(32.12395179909,1.014547269612,0.3894482114171));
#16272=CARTESIAN_POINT('Ctrl Pts',(32.07520179909,1.033538954174,-0.3358171723489));
#16273=CARTESIAN_POINT('Ctrl Pts',(32.02645179909,0.5918740460484,-0.9114061000685));
#16274=CARTESIAN_POINT('Ctrl Pts',(31.97770179909,-0.1135939230171,-1.080773975495));
#16275=CARTESIAN_POINT('Ctrl Pts',(31.92895179909,-0.7684321582634,-0.7684321583925));
#16276=CARTESIAN_POINT('Ctrl Pts',(31.88020179909,-1.080773975171,-0.1135939221766));
#16277=CARTESIAN_POINT('Ctrl Pts',(31.83145179909,-0.9114061014946,0.5918740428154));
#16278=CARTESIAN_POINT('Ctrl Pts',(31.78270179909,-0.3358171669691,1.033538966266));
#16279=CARTESIAN_POINT('Ctrl Pts',(31.73395179909,0.3894481913237,1.014547224479));
#16280=CARTESIAN_POINT('Ctrl Pts',(31.68520179909,0.9411333451298,0.543363590154));
#16281=CARTESIAN_POINT('Ctrl Pts',(31.63645179909,1.0733477654,-0.1700015850955));
#16282=CARTESIAN_POINT('Ctrl Pts',(31.58770179909,0.7271624171027,-0.807595680755));
#16283=CARTESIAN_POINT('Ctrl Pts',(31.53895179909,0.05687490617145,-1.085237858466));
#16284=CARTESIAN_POINT('Ctrl Pts',(31.49020179909,-0.6387622099061,-0.8791807571591));
#16285=CARTESIAN_POINT('Ctrl Pts',(31.44145179909,-1.049697849384,-0.2812656909448));
#16286=CARTESIAN_POINT('Ctrl Pts',(31.39270179909,-0.9927746800367,0.4420117646994));
#16287=CARTESIAN_POINT('Ctrl Pts',(31.34395179909,-0.4933638127992,0.9682810097529));
#16288=CARTESIAN_POINT('Ctrl Pts',(31.29520179909,0.2259432748059,1.06297957629));
#16289=CARTESIAN_POINT('Ctrl Pts',(31.24645179909,0.8445456793518,0.6838996031158));
#16290=CARTESIAN_POINT('Ctrl Pts',(31.19770179909,1.086727031141,-1.083766177912E-7));
#16291=CARTESIAN_POINT('Ctrl Pts',(31.14895179909,0.8445461960836,-0.6838991696094));
#16292=CARTESIAN_POINT('Ctrl Pts',(31.10020179909,0.2259412078788,-1.062981093563));
#16293=CARTESIAN_POINT('Ctrl Pts',(31.05145179909,-0.4933560618227,-0.9682753741689));
#16294=CARTESIAN_POINT('Ctrl Pts',(31.00270179909,-0.9928036170159,-0.4420327897627));
#16295=CARTESIAN_POINT('Ctrl Pts',(30.95395179909,-1.049589852444,0.2813441556141));
#16296=CARTESIAN_POINT('Ctrl Pts',(30.92145179909,-0.7759734579398,0.6797066675681));
#16297=CARTESIAN_POINT('Ctrl Pts',(30.90520179909,-0.5913119638062,0.8138710963412));
#16298=CARTESIAN_POINT('Ctrl Pts',(32.37979820091,0.4091770629343,-0.9190267303885));
#16299=CARTESIAN_POINT('Ctrl Pts',(32.36354820091,0.2006565122657,-1.011866061022));
#16300=CARTESIAN_POINT('Ctrl Pts',(32.33104820091,-0.2811437402541,-1.049643553578));
#16301=CARTESIAN_POINT('Ctrl Pts',(32.28229820091,-0.8792134337482,-0.6387767584235));
#16302=CARTESIAN_POINT('Ctrl Pts',(32.23354820091,-1.0852291028,0.05687880443496));
#16303=CARTESIAN_POINT('Ctrl Pts',(32.18479820091,-0.8075980268285,0.7271613725661));
#16304=CARTESIAN_POINT('Ctrl Pts',(32.13604820091,-0.170000956467,1.073348045283));
#16305=CARTESIAN_POINT('Ctrl Pts',(32.08729820091,0.5433634217137,0.9411332701358));
#16306=CARTESIAN_POINT('Ctrl Pts',(32.03854820091,1.014547269612,0.3894482114171));
#16307=CARTESIAN_POINT('Ctrl Pts',(31.98979820091,1.033538954174,-0.3358171723489));
#16308=CARTESIAN_POINT('Ctrl Pts',(31.94104820091,0.5918740460484,-0.9114061000685));
#16309=CARTESIAN_POINT('Ctrl Pts',(31.89229820091,-0.1135939230171,-1.080773975495));
#16310=CARTESIAN_POINT('Ctrl Pts',(31.84354820091,-0.7684321582634,-0.7684321583925));
#16311=CARTESIAN_POINT('Ctrl Pts',(31.79479820091,-1.080773975171,-0.1135939221766));
#16312=CARTESIAN_POINT('Ctrl Pts',(31.74604820091,-0.9114061014946,0.5918740428154));
#16313=CARTESIAN_POINT('Ctrl Pts',(31.69729820091,-0.3358171669691,1.033538966266));
#16314=CARTESIAN_POINT('Ctrl Pts',(31.64854820091,0.3894481913237,1.014547224479));
#16315=CARTESIAN_POINT('Ctrl Pts',(31.59979820091,0.9411333451298,0.543363590154));
#16316=CARTESIAN_POINT('Ctrl Pts',(31.55104820091,1.0733477654,-0.1700015850955));
#16317=CARTESIAN_POINT('Ctrl Pts',(31.50229820091,0.7271624171027,-0.807595680755));
#16318=CARTESIAN_POINT('Ctrl Pts',(31.45354820091,0.05687490617145,-1.085237858466));
#16319=CARTESIAN_POINT('Ctrl Pts',(31.40479820091,-0.6387622099061,-0.8791807571591));
#16320=CARTESIAN_POINT('Ctrl Pts',(31.35604820091,-1.049697849384,-0.2812656909448));
#16321=CARTESIAN_POINT('Ctrl Pts',(31.30729820091,-0.9927746800367,0.4420117646994));
#16322=CARTESIAN_POINT('Ctrl Pts',(31.25854820091,-0.4933638127992,0.9682810097529));
#16323=CARTESIAN_POINT('Ctrl Pts',(31.20979820091,0.2259432748059,1.06297957629));
#16324=CARTESIAN_POINT('Ctrl Pts',(31.16104820091,0.8445456793518,0.6838996031158));
#16325=CARTESIAN_POINT('Ctrl Pts',(31.11229820091,1.086727031141,-1.083766177912E-7));
#16326=CARTESIAN_POINT('Ctrl Pts',(31.06354820091,0.8445461960836,-0.6838991696094));
#16327=CARTESIAN_POINT('Ctrl Pts',(31.01479820091,0.2259412078788,-1.062981093563));
#16328=CARTESIAN_POINT('Ctrl Pts',(30.96604820091,-0.4933560618227,-0.9682753741689));
#16329=CARTESIAN_POINT('Ctrl Pts',(30.91729820091,-0.9928036170159,-0.4420327897627));
#16330=CARTESIAN_POINT('Ctrl Pts',(30.86854820091,-1.049589852444,0.2813441556141));
#16331=CARTESIAN_POINT('Ctrl Pts',(30.83604820091,-0.7759734579398,0.6797066675681));
#16332=CARTESIAN_POINT('Ctrl Pts',(30.81979820091,-0.5913119638062,0.8138710963412));
#16333=CARTESIAN_POINT('Ctrl Pts',(32.29439460273,0.4091770629343,-0.9190267303885));
#16334=CARTESIAN_POINT('Ctrl Pts',(32.27814460273,0.2006565122657,-1.011866061022));
#16335=CARTESIAN_POINT('Ctrl Pts',(32.24564460273,-0.2811437402541,-1.049643553578));
#16336=CARTESIAN_POINT('Ctrl Pts',(32.19689460273,-0.8792134337482,-0.6387767584235));
#16337=CARTESIAN_POINT('Ctrl Pts',(32.14814460273,-1.0852291028,0.05687880443496));
#16338=CARTESIAN_POINT('Ctrl Pts',(32.09939460273,-0.8075980268285,0.7271613725661));
#16339=CARTESIAN_POINT('Ctrl Pts',(32.05064460273,-0.170000956467,1.073348045283));
#16340=CARTESIAN_POINT('Ctrl Pts',(32.00189460273,0.5433634217137,0.9411332701358));
#16341=CARTESIAN_POINT('Ctrl Pts',(31.95314460273,1.014547269612,0.3894482114171));
#16342=CARTESIAN_POINT('Ctrl Pts',(31.90439460273,1.033538954174,-0.3358171723489));
#16343=CARTESIAN_POINT('Ctrl Pts',(31.85564460273,0.5918740460484,-0.9114061000685));
#16344=CARTESIAN_POINT('Ctrl Pts',(31.80689460273,-0.1135939230171,-1.080773975495));
#16345=CARTESIAN_POINT('Ctrl Pts',(31.75814460273,-0.7684321582634,-0.7684321583925));
#16346=CARTESIAN_POINT('Ctrl Pts',(31.70939460273,-1.080773975171,-0.1135939221766));
#16347=CARTESIAN_POINT('Ctrl Pts',(31.66064460273,-0.9114061014946,0.5918740428154));
#16348=CARTESIAN_POINT('Ctrl Pts',(31.61189460273,-0.3358171669691,1.033538966266));
#16349=CARTESIAN_POINT('Ctrl Pts',(31.56314460273,0.3894481913237,1.014547224479));
#16350=CARTESIAN_POINT('Ctrl Pts',(31.51439460273,0.9411333451298,0.543363590154));
#16351=CARTESIAN_POINT('Ctrl Pts',(31.46564460273,1.0733477654,-0.1700015850955));
#16352=CARTESIAN_POINT('Ctrl Pts',(31.41689460273,0.7271624171027,-0.807595680755));
#16353=CARTESIAN_POINT('Ctrl Pts',(31.36814460273,0.05687490617145,-1.085237858466));
#16354=CARTESIAN_POINT('Ctrl Pts',(31.31939460273,-0.6387622099061,-0.8791807571591));
#16355=CARTESIAN_POINT('Ctrl Pts',(31.27064460273,-1.049697849384,-0.2812656909448));
#16356=CARTESIAN_POINT('Ctrl Pts',(31.22189460273,-0.9927746800367,0.4420117646994));
#16357=CARTESIAN_POINT('Ctrl Pts',(31.17314460273,-0.4933638127992,0.9682810097529));
#16358=CARTESIAN_POINT('Ctrl Pts',(31.12439460273,0.2259432748059,1.06297957629));
#16359=CARTESIAN_POINT('Ctrl Pts',(31.07564460273,0.8445456793518,0.6838996031158));
#16360=CARTESIAN_POINT('Ctrl Pts',(31.02689460273,1.086727031141,-1.083766177912E-7));
#16361=CARTESIAN_POINT('Ctrl Pts',(30.97814460273,0.8445461960836,-0.6838991696094));
#16362=CARTESIAN_POINT('Ctrl Pts',(30.92939460273,0.2259412078788,-1.062981093563));
#16363=CARTESIAN_POINT('Ctrl Pts',(30.88064460273,-0.4933560618227,-0.9682753741689));
#16364=CARTESIAN_POINT('Ctrl Pts',(30.83189460273,-0.9928036170159,-0.4420327897627));
#16365=CARTESIAN_POINT('Ctrl Pts',(30.78314460273,-1.049589852444,0.2813441556141));
#16366=CARTESIAN_POINT('Ctrl Pts',(30.75064460273,-0.7759734579398,0.6797066675681));
#16367=CARTESIAN_POINT('Ctrl Pts',(30.73439460273,-0.5913119638062,0.8138710963412));
#16368=CARTESIAN_POINT('',(30.97662653432,-0.8712215562071,0.503));
#16369=CARTESIAN_POINT('Ctrl Pts',(31.05060539727,-1.00048902674,0.1051556340473));
#16370=CARTESIAN_POINT('Ctrl Pts',(31.03435539727,-0.9766299702056,0.3321593934543));
#16371=CARTESIAN_POINT('Ctrl Pts',(31.00185539727,-0.7684461121902,0.7682993979641));
#16372=CARTESIAN_POINT('Ctrl Pts',(30.95310539727,-0.1135901832678,1.080809548186));
#16373=CARTESIAN_POINT('Ctrl Pts',(30.90435539727,0.5918730409778,0.9113965697339));
#16374=CARTESIAN_POINT('Ctrl Pts',(30.85560539727,1.033539234707,0.3358197209966));
#16375=CARTESIAN_POINT('Ctrl Pts',(30.80685539727,1.014547152551,-0.3894488756732));
#16376=CARTESIAN_POINT('Ctrl Pts',(30.75810539727,0.5433636094275,-0.9411331617592));
#16377=CARTESIAN_POINT('Ctrl Pts',(30.70935539727,-0.1700015902605,-1.073347814533));
#16378=CARTESIAN_POINT('Ctrl Pts',(30.66060539727,-0.8075956793684,-0.7271624039412));
#16379=CARTESIAN_POINT('Ctrl Pts',(30.61185539727,-1.085237858848,-0.05687490968431));
#16380=CARTESIAN_POINT('Ctrl Pts',(30.56310539727,-0.8791807570196,0.6387622107961));
#16381=CARTESIAN_POINT('Ctrl Pts',(30.51435539727,-0.2812656911211,1.049697849337));
#16382=CARTESIAN_POINT('Ctrl Pts',(30.46560539727,0.4420117652652,0.9927746793357));
#16383=CARTESIAN_POINT('Ctrl Pts',(30.41685539727,0.968281007666,0.4933638156507));
#16384=CARTESIAN_POINT('Ctrl Pts',(30.36810539727,1.062979584072,-0.2259432855107));
#16385=CARTESIAN_POINT('Ctrl Pts',(30.31935539727,0.6838995740763,-0.8445456393839));
#16386=CARTESIAN_POINT('Ctrl Pts',(30.27060539727,-1.795785742331E-14,-1.086727180308));
#16387=CARTESIAN_POINT('Ctrl Pts',(30.22185539727,-0.6838995740763,-0.8445456393839));
#16388=CARTESIAN_POINT('Ctrl Pts',(30.17310539727,-1.062979584072,-0.2259432855107));
#16389=CARTESIAN_POINT('Ctrl Pts',(30.12435539727,-0.968281007666,0.4933638156508));
#16390=CARTESIAN_POINT('Ctrl Pts',(30.07560539727,-0.4420117652651,0.9927746793357));
#16391=CARTESIAN_POINT('Ctrl Pts',(30.02685539727,0.2812656911211,1.049697849337));
#16392=CARTESIAN_POINT('Ctrl Pts',(29.97810539727,0.8791807570196,0.6387622107961));
#16393=CARTESIAN_POINT('Ctrl Pts',(29.92935539727,1.085237858848,-0.05687490968435));
#16394=CARTESIAN_POINT('Ctrl Pts',(29.88060539727,0.8075956793683,-0.7271624039412));
#16395=CARTESIAN_POINT('Ctrl Pts',(29.83185539727,0.1700015902605,-1.073347814533));
#16396=CARTESIAN_POINT('Ctrl Pts',(29.78310539727,-0.5433636094275,-0.9411331617592));
#16397=CARTESIAN_POINT('Ctrl Pts',(29.73435539727,-1.014547152551,-0.3894488756732));
#16398=CARTESIAN_POINT('Ctrl Pts',(29.68560539727,-1.033539234707,0.3358197209966));
#16399=CARTESIAN_POINT('Ctrl Pts',(29.63685539727,-0.5918730409778,0.9113965697339));
#16400=CARTESIAN_POINT('Ctrl Pts',(29.58810539727,0.1135901832678,1.080809548186));
#16401=CARTESIAN_POINT('Ctrl Pts',(29.53935539727,0.7684461121903,0.7682993979641));
#16402=CARTESIAN_POINT('Ctrl Pts',(29.50685539727,0.9766299702056,0.3321593934543));
#16403=CARTESIAN_POINT('Ctrl Pts',(29.49060539727,1.00048902674,0.1051556340472));
#16404=CARTESIAN_POINT('Ctrl Pts',(30.96520179909,-1.00048902674,0.1051556340473));
#16405=CARTESIAN_POINT('Ctrl Pts',(30.94895179909,-0.9766299702056,0.3321593934543));
#16406=CARTESIAN_POINT('Ctrl Pts',(30.91645179909,-0.7684461121902,0.7682993979641));
#16407=CARTESIAN_POINT('Ctrl Pts',(30.86770179909,-0.1135901832678,1.080809548186));
#16408=CARTESIAN_POINT('Ctrl Pts',(30.81895179909,0.5918730409778,0.9113965697339));
#16409=CARTESIAN_POINT('Ctrl Pts',(30.77020179909,1.033539234707,0.3358197209966));
#16410=CARTESIAN_POINT('Ctrl Pts',(30.72145179909,1.014547152551,-0.3894488756732));
#16411=CARTESIAN_POINT('Ctrl Pts',(30.67270179909,0.5433636094275,-0.9411331617592));
#16412=CARTESIAN_POINT('Ctrl Pts',(30.62395179909,-0.1700015902605,-1.073347814533));
#16413=CARTESIAN_POINT('Ctrl Pts',(30.57520179909,-0.8075956793684,-0.7271624039412));
#16414=CARTESIAN_POINT('Ctrl Pts',(30.52645179909,-1.085237858848,-0.05687490968431));
#16415=CARTESIAN_POINT('Ctrl Pts',(30.47770179909,-0.8791807570196,0.6387622107961));
#16416=CARTESIAN_POINT('Ctrl Pts',(30.42895179909,-0.2812656911211,1.049697849337));
#16417=CARTESIAN_POINT('Ctrl Pts',(30.38020179909,0.4420117652652,0.9927746793357));
#16418=CARTESIAN_POINT('Ctrl Pts',(30.33145179909,0.968281007666,0.4933638156507));
#16419=CARTESIAN_POINT('Ctrl Pts',(30.28270179909,1.062979584072,-0.2259432855107));
#16420=CARTESIAN_POINT('Ctrl Pts',(30.23395179909,0.6838995740763,-0.8445456393839));
#16421=CARTESIAN_POINT('Ctrl Pts',(30.18520179909,-1.795785742331E-14,-1.086727180308));
#16422=CARTESIAN_POINT('Ctrl Pts',(30.13645179909,-0.6838995740763,-0.8445456393839));
#16423=CARTESIAN_POINT('Ctrl Pts',(30.08770179909,-1.062979584072,-0.2259432855107));
#16424=CARTESIAN_POINT('Ctrl Pts',(30.03895179909,-0.968281007666,0.4933638156508));
#16425=CARTESIAN_POINT('Ctrl Pts',(29.99020179909,-0.4420117652651,0.9927746793357));
#16426=CARTESIAN_POINT('Ctrl Pts',(29.94145179909,0.2812656911211,1.049697849337));
#16427=CARTESIAN_POINT('Ctrl Pts',(29.89270179909,0.8791807570196,0.6387622107961));
#16428=CARTESIAN_POINT('Ctrl Pts',(29.84395179909,1.085237858848,-0.05687490968435));
#16429=CARTESIAN_POINT('Ctrl Pts',(29.79520179909,0.8075956793683,-0.7271624039412));
#16430=CARTESIAN_POINT('Ctrl Pts',(29.74645179909,0.1700015902605,-1.073347814533));
#16431=CARTESIAN_POINT('Ctrl Pts',(29.69770179909,-0.5433636094275,-0.9411331617592));
#16432=CARTESIAN_POINT('Ctrl Pts',(29.64895179909,-1.014547152551,-0.3894488756732));
#16433=CARTESIAN_POINT('Ctrl Pts',(29.60020179909,-1.033539234707,0.3358197209966));
#16434=CARTESIAN_POINT('Ctrl Pts',(29.55145179909,-0.5918730409778,0.9113965697339));
#16435=CARTESIAN_POINT('Ctrl Pts',(29.50270179909,0.1135901832678,1.080809548186));
#16436=CARTESIAN_POINT('Ctrl Pts',(29.45395179909,0.7684461121903,0.7682993979641));
#16437=CARTESIAN_POINT('Ctrl Pts',(29.42145179909,0.9766299702056,0.3321593934543));
#16438=CARTESIAN_POINT('Ctrl Pts',(29.40520179909,1.00048902674,0.1051556340472));
#16439=CARTESIAN_POINT('Ctrl Pts',(30.87979820091,-1.00048902674,0.1051556340473));
#16440=CARTESIAN_POINT('Ctrl Pts',(30.86354820091,-0.9766299702056,0.3321593934543));
#16441=CARTESIAN_POINT('Ctrl Pts',(30.83104820091,-0.7684461121902,0.7682993979641));
#16442=CARTESIAN_POINT('Ctrl Pts',(30.78229820091,-0.1135901832678,1.080809548186));
#16443=CARTESIAN_POINT('Ctrl Pts',(30.73354820091,0.5918730409778,0.9113965697339));
#16444=CARTESIAN_POINT('Ctrl Pts',(30.68479820091,1.033539234707,0.3358197209966));
#16445=CARTESIAN_POINT('Ctrl Pts',(30.63604820091,1.014547152551,-0.3894488756732));
#16446=CARTESIAN_POINT('Ctrl Pts',(30.58729820091,0.5433636094275,-0.9411331617592));
#16447=CARTESIAN_POINT('Ctrl Pts',(30.53854820091,-0.1700015902605,-1.073347814533));
#16448=CARTESIAN_POINT('Ctrl Pts',(30.48979820091,-0.8075956793684,-0.7271624039412));
#16449=CARTESIAN_POINT('Ctrl Pts',(30.44104820091,-1.085237858848,-0.05687490968431));
#16450=CARTESIAN_POINT('Ctrl Pts',(30.39229820091,-0.8791807570196,0.6387622107961));
#16451=CARTESIAN_POINT('Ctrl Pts',(30.34354820091,-0.2812656911211,1.049697849337));
#16452=CARTESIAN_POINT('Ctrl Pts',(30.29479820091,0.4420117652652,0.9927746793357));
#16453=CARTESIAN_POINT('Ctrl Pts',(30.24604820091,0.968281007666,0.4933638156507));
#16454=CARTESIAN_POINT('Ctrl Pts',(30.19729820091,1.062979584072,-0.2259432855107));
#16455=CARTESIAN_POINT('Ctrl Pts',(30.14854820091,0.6838995740763,-0.8445456393839));
#16456=CARTESIAN_POINT('Ctrl Pts',(30.09979820091,-1.795785742331E-14,-1.086727180308));
#16457=CARTESIAN_POINT('Ctrl Pts',(30.05104820091,-0.6838995740763,-0.8445456393839));
#16458=CARTESIAN_POINT('Ctrl Pts',(30.00229820091,-1.062979584072,-0.2259432855107));
#16459=CARTESIAN_POINT('Ctrl Pts',(29.95354820091,-0.968281007666,0.4933638156508));
#16460=CARTESIAN_POINT('Ctrl Pts',(29.90479820091,-0.4420117652651,0.9927746793357));
#16461=CARTESIAN_POINT('Ctrl Pts',(29.85604820091,0.2812656911211,1.049697849337));
#16462=CARTESIAN_POINT('Ctrl Pts',(29.80729820091,0.8791807570196,0.6387622107961));
#16463=CARTESIAN_POINT('Ctrl Pts',(29.75854820091,1.085237858848,-0.05687490968435));
#16464=CARTESIAN_POINT('Ctrl Pts',(29.70979820091,0.8075956793683,-0.7271624039412));
#16465=CARTESIAN_POINT('Ctrl Pts',(29.66104820091,0.1700015902605,-1.073347814533));
#16466=CARTESIAN_POINT('Ctrl Pts',(29.61229820091,-0.5433636094275,-0.9411331617592));
#16467=CARTESIAN_POINT('Ctrl Pts',(29.56354820091,-1.014547152551,-0.3894488756732));
#16468=CARTESIAN_POINT('Ctrl Pts',(29.51479820091,-1.033539234707,0.3358197209966));
#16469=CARTESIAN_POINT('Ctrl Pts',(29.46604820091,-0.5918730409778,0.9113965697339));
#16470=CARTESIAN_POINT('Ctrl Pts',(29.41729820091,0.1135901832678,1.080809548186));
#16471=CARTESIAN_POINT('Ctrl Pts',(29.36854820091,0.7684461121903,0.7682993979641));
#16472=CARTESIAN_POINT('Ctrl Pts',(29.33604820091,0.9766299702056,0.3321593934543));
#16473=CARTESIAN_POINT('Ctrl Pts',(29.31979820091,1.00048902674,0.1051556340472));
#16474=CARTESIAN_POINT('Ctrl Pts',(30.79439460273,-1.00048902674,0.1051556340473));
#16475=CARTESIAN_POINT('Ctrl Pts',(30.77814460273,-0.9766299702056,0.3321593934543));
#16476=CARTESIAN_POINT('Ctrl Pts',(30.74564460273,-0.7684461121902,0.7682993979641));
#16477=CARTESIAN_POINT('Ctrl Pts',(30.69689460273,-0.1135901832678,1.080809548186));
#16478=CARTESIAN_POINT('Ctrl Pts',(30.64814460273,0.5918730409778,0.9113965697339));
#16479=CARTESIAN_POINT('Ctrl Pts',(30.59939460273,1.033539234707,0.3358197209966));
#16480=CARTESIAN_POINT('Ctrl Pts',(30.55064460273,1.014547152551,-0.3894488756732));
#16481=CARTESIAN_POINT('Ctrl Pts',(30.50189460273,0.5433636094275,-0.9411331617592));
#16482=CARTESIAN_POINT('Ctrl Pts',(30.45314460273,-0.1700015902605,-1.073347814533));
#16483=CARTESIAN_POINT('Ctrl Pts',(30.40439460273,-0.8075956793684,-0.7271624039412));
#16484=CARTESIAN_POINT('Ctrl Pts',(30.35564460273,-1.085237858848,-0.05687490968431));
#16485=CARTESIAN_POINT('Ctrl Pts',(30.30689460273,-0.8791807570196,0.6387622107961));
#16486=CARTESIAN_POINT('Ctrl Pts',(30.25814460273,-0.2812656911211,1.049697849337));
#16487=CARTESIAN_POINT('Ctrl Pts',(30.20939460273,0.4420117652652,0.9927746793357));
#16488=CARTESIAN_POINT('Ctrl Pts',(30.16064460273,0.968281007666,0.4933638156507));
#16489=CARTESIAN_POINT('Ctrl Pts',(30.11189460273,1.062979584072,-0.2259432855107));
#16490=CARTESIAN_POINT('Ctrl Pts',(30.06314460273,0.6838995740763,-0.8445456393839));
#16491=CARTESIAN_POINT('Ctrl Pts',(30.01439460273,-1.795785742331E-14,-1.086727180308));
#16492=CARTESIAN_POINT('Ctrl Pts',(29.96564460273,-0.6838995740763,-0.8445456393839));
#16493=CARTESIAN_POINT('Ctrl Pts',(29.91689460273,-1.062979584072,-0.2259432855107));
#16494=CARTESIAN_POINT('Ctrl Pts',(29.86814460273,-0.968281007666,0.4933638156508));
#16495=CARTESIAN_POINT('Ctrl Pts',(29.81939460273,-0.4420117652651,0.9927746793357));
#16496=CARTESIAN_POINT('Ctrl Pts',(29.77064460273,0.2812656911211,1.049697849337));
#16497=CARTESIAN_POINT('Ctrl Pts',(29.72189460273,0.8791807570196,0.6387622107961));
#16498=CARTESIAN_POINT('Ctrl Pts',(29.67314460273,1.085237858848,-0.05687490968435));
#16499=CARTESIAN_POINT('Ctrl Pts',(29.62439460273,0.8075956793683,-0.7271624039412));
#16500=CARTESIAN_POINT('Ctrl Pts',(29.57564460273,0.1700015902605,-1.073347814533));
#16501=CARTESIAN_POINT('Ctrl Pts',(29.52689460273,-0.5433636094275,-0.9411331617592));
#16502=CARTESIAN_POINT('Ctrl Pts',(29.47814460273,-1.014547152551,-0.3894488756732));
#16503=CARTESIAN_POINT('Ctrl Pts',(29.42939460273,-1.033539234707,0.3358197209966));
#16504=CARTESIAN_POINT('Ctrl Pts',(29.38064460273,-0.5918730409778,0.9113965697339));
#16505=CARTESIAN_POINT('Ctrl Pts',(29.33189460273,0.1135901832678,1.080809548186));
#16506=CARTESIAN_POINT('Ctrl Pts',(29.28314460273,0.7684461121903,0.7682993979641));
#16507=CARTESIAN_POINT('Ctrl Pts',(29.25064460273,0.9766299702056,0.3321593934543));
#16508=CARTESIAN_POINT('Ctrl Pts',(29.23439460273,1.00048902674,0.1051556340472));
#16509=CARTESIAN_POINT('',(29.308373466651,0.871221485691904,0.502999959536925));
#16510=CARTESIAN_POINT('Ctrl Pts',(30.8083864422337,-0.870772069750912,
0.502741978477052));
#16511=CARTESIAN_POINT('Ctrl Pts',(30.8008521885261,-0.818004270752092,
0.594472186190461));
#16512=CARTESIAN_POINT('Ctrl Pts',(30.7920928354003,-0.74226233496147,0.694100380026428));
#16513=CARTESIAN_POINT('Ctrl Pts',(30.7731153143573,-0.534424048498561,
0.860636605924475));
#16514=CARTESIAN_POINT('Ctrl Pts',(30.7642892222818,-0.423170162032183,
0.920186008439541));
#16515=CARTESIAN_POINT('Ctrl Pts',(30.7460042305897,-0.178646956831074,
0.998775584332035));
#16516=CARTESIAN_POINT('Ctrl Pts',(30.7367588244469,-0.0472837866908757,
1.01362569808423));
#16517=CARTESIAN_POINT('Ctrl Pts',(30.7180479571781,0.214494381189115,0.990633906486489));
#16518=CARTESIAN_POINT('Ctrl Pts',(30.7088151157514,0.341677793262393,0.954510297187085));
#16519=CARTESIAN_POINT('Ctrl Pts',(30.6886171121704,0.594508302867244,0.826283085072341));
#16520=CARTESIAN_POINT('Ctrl Pts',(30.6792516786672,0.693921902387751,0.736013762237494));
#16521=CARTESIAN_POINT('Ctrl Pts',(30.6624059009715,0.847217927666136,0.555636629667067));
#16522=CARTESIAN_POINT('Ctrl Pts',(30.6534069464233,0.911379127217043,0.4441108841133));
#16523=CARTESIAN_POINT('Ctrl Pts',(30.6342989682698,0.998002528379833,0.190430974375329));
#16524=CARTESIAN_POINT('Ctrl Pts',(30.6247947693779,1.01157017614526,0.0548890692946352));
#16525=CARTESIAN_POINT('Ctrl Pts',(30.6082077163493,0.995521631670858,-0.17764597144364));
#16526=CARTESIAN_POINT('Ctrl Pts',(30.5990210738254,0.970098454855203,-0.306791753619249));
#16527=CARTESIAN_POINT('Ctrl Pts',(30.5788719338335,0.845240586957547,-0.560500408959282));
#16528=CARTESIAN_POINT('Ctrl Pts',(30.5694606001009,0.763151979773334,-0.667500700456631));
#16529=CARTESIAN_POINT('Ctrl Pts',(30.5505675506108,0.564358031936664,-0.843275682317893));
#16530=CARTESIAN_POINT('Ctrl Pts',(30.5413142276786,0.449835071540398,-0.909552155701698));
#16531=CARTESIAN_POINT('Ctrl Pts',(30.5226106191189,0.200891944607366,-0.993435412233473));
#16532=CARTESIAN_POINT('Ctrl Pts',(30.5133914653587,0.0701110249796663,
-1.01138590544987));
#16533=CARTESIAN_POINT('Ctrl Pts',(30.4931854475347,-0.213025964557814,
-0.995444387176705));
#16534=CARTESIAN_POINT('Ctrl Pts',(30.483806736634,-0.34046753425378,-0.952477692807911));
#16535=CARTESIAN_POINT('Ctrl Pts',(30.4670009367566,-0.552782663940084,
-0.84906487250493));
#16536=CARTESIAN_POINT('Ctrl Pts',(30.45801688248,-0.656165051344275,-0.772850244059696));
#16537=CARTESIAN_POINT('Ctrl Pts',(30.4394916971384,-0.831881844613014,
-0.581371288177416));
#16538=CARTESIAN_POINT('Ctrl Pts',(30.4299862507459,-0.901486061152791,
-0.464335182585286));
#16539=CARTESIAN_POINT('Ctrl Pts',(30.4128021772268,-0.983138694974887,
-0.237085248117362));
#16540=CARTESIAN_POINT('Ctrl Pts',(30.4036116032871,-1.01164457155601,-0.108534779049115));
#16541=CARTESIAN_POINT('Ctrl Pts',(30.3834719027531,-0.99914720466093,0.17383498727286));
#16542=CARTESIAN_POINT('Ctrl Pts',(30.3740686495797,-0.967009114614636,
0.304690319176165));
#16543=CARTESIAN_POINT('Ctrl Pts',(30.3551692839619,-0.855581407083058,
0.545608350968359));
#16544=CARTESIAN_POINT('Ctrl Pts',(30.3459048150743,-0.777163779775291,
0.652387656279846));
#16545=CARTESIAN_POINT('Ctrl Pts',(30.3272137745115,-0.582980235794567,
0.829064401206589));
#16546=CARTESIAN_POINT('Ctrl Pts',(30.3180068956466,-0.470601448908796,
0.897970498795624));
#16547=CARTESIAN_POINT('Ctrl Pts',(30.2977899305544,-0.204799025246617,
0.997222455929395));
#16548=CARTESIAN_POINT('Ctrl Pts',(30.2883977032763,-0.07061115429442,1.0089765786811));
#16549=CARTESIAN_POINT('Ctrl Pts',(30.2716308252545,0.164820890836547,0.999641820194012));
#16550=CARTESIAN_POINT('Ctrl Pts',(30.2626606378465,0.289920670515312,0.971492512618052));
#16551=CARTESIAN_POINT('Ctrl Pts',(30.2441622029206,0.527466569099338,0.867007573502011));
#16552=CARTESIAN_POINT('Ctrl Pts',(30.2346587869632,0.638304838566819,0.787948218222781));
#16553=CARTESIAN_POINT('Ctrl Pts',(30.2174342420197,0.804917354004863,0.612382577780543));
#16554=CARTESIAN_POINT('Ctrl Pts',(30.2082400320689,0.882667521494572,0.506058560714851));
#16555=CARTESIAN_POINT('Ctrl Pts',(30.1881085385381,0.984682436642582,0.242576766412211));
#16556=CARTESIAN_POINT('Ctrl Pts',(30.1787128604578,1.00788845481734,0.109958040776812));
#16557=CARTESIAN_POINT('Ctrl Pts',(30.1598090757102,1.00280273292441,-0.155484472839208));
#16558=CARTESIAN_POINT('Ctrl Pts',(30.1505332144177,0.973839811222991,-0.284930092981155));
#16559=CARTESIAN_POINT('Ctrl Pts',(30.1318547354579,0.867144006061644,-0.524617833052899));
#16560=CARTESIAN_POINT('Ctrl Pts',(30.1226591218941,0.792089695015471,-0.632780197940589));
#16561=CARTESIAN_POINT('Ctrl Pts',(30.1024311543348,0.588587875794969,-0.830697511597098));
#16562=CARTESIAN_POINT('Ctrl Pts',(30.093026368846,0.470235006290618,-0.895430023340954));
#16563=CARTESIAN_POINT('Ctrl Pts',(30.0762958650647,0.251421288995113,-0.981433054835685));
#16564=CARTESIAN_POINT('Ctrl Pts',(30.0673383109915,0.12576520800403,-1.00599999999997));
#16565=CARTESIAN_POINT('Ctrl Pts',(30.0494086203685,-0.125765208004121,
-1.00599999999996));
#16566=CARTESIAN_POINT('Ctrl Pts',(30.0404510663023,-0.251421288995195,
-0.98143305483567));
#16567=CARTESIAN_POINT('Ctrl Pts',(30.0237205625209,-0.470235006290693,
-0.895430023340922));
#16568=CARTESIAN_POINT('Ctrl Pts',(30.0143157770321,-0.588587875795033,
-0.830697511597058));
#16569=CARTESIAN_POINT('Ctrl Pts',(29.9940878094728,-0.79208969501552,-0.63278019794053));
#16570=CARTESIAN_POINT('Ctrl Pts',(29.984892195909,-0.867144006061687,-0.524617833052829));
#16571=CARTESIAN_POINT('Ctrl Pts',(29.9662137169491,-0.973839811223016,
-0.28493009298106));
#16572=CARTESIAN_POINT('Ctrl Pts',(29.9569378556566,-1.00280273292442,-0.155484472839104));
#16573=CARTESIAN_POINT('Ctrl Pts',(29.938034070909,-1.00788845481734,0.109958040776938));
#16574=CARTESIAN_POINT('Ctrl Pts',(29.9286383928286,-0.984682436642559,
0.242576766412358));
#16575=CARTESIAN_POINT('Ctrl Pts',(29.9085068992979,-0.882667521494521,
0.506058560714965));
#16576=CARTESIAN_POINT('Ctrl Pts',(29.8993126893471,-0.804917354004816,
0.61238257778062));
#16577=CARTESIAN_POINT('Ctrl Pts',(29.8820881444036,-0.638304838566773,
0.787948218222813));
#16578=CARTESIAN_POINT('Ctrl Pts',(29.8725847284462,-0.527466569099291,
0.867007573502023));
#16579=CARTESIAN_POINT('Ctrl Pts',(29.8540862935204,-0.289920670515246,
0.971492512618064));
#16580=CARTESIAN_POINT('Ctrl Pts',(29.8451161061125,-0.164820890836453,
0.999641820194026));
#16581=CARTESIAN_POINT('Ctrl Pts',(29.8283492280908,0.0706111542945384,
1.00897657868109));
#16582=CARTESIAN_POINT('Ctrl Pts',(29.8189570008127,0.204799025246714,0.997222455929378));
#16583=CARTESIAN_POINT('Ctrl Pts',(29.7987400357205,0.470601448908869,0.897970498795589));
#16584=CARTESIAN_POINT('Ctrl Pts',(29.7895331568555,0.582980235794636,0.829064401206542));
#16585=CARTESIAN_POINT('Ctrl Pts',(29.7708421162926,0.777163779775349,0.652387656279774));
#16586=CARTESIAN_POINT('Ctrl Pts',(29.7615776474049,0.855581407083106,0.545608350968274));
#16587=CARTESIAN_POINT('Ctrl Pts',(29.7426782817869,0.967009114614662,0.30469031917606));
#16588=CARTESIAN_POINT('Ctrl Pts',(29.7332750286134,0.999147204660943,0.173834987272742));
#16589=CARTESIAN_POINT('Ctrl Pts',(29.7131353280793,1.01164457155598,-0.108534779049213));
#16590=CARTESIAN_POINT('Ctrl Pts',(29.7039447541397,0.983138694974841,-0.237085248117433));
#16591=CARTESIAN_POINT('Ctrl Pts',(29.6867606806207,0.901486061152719,-0.464335182585334));
#16592=CARTESIAN_POINT('Ctrl Pts',(29.6772552342284,0.831881844612926,-0.581371288177457));
#16593=CARTESIAN_POINT('Ctrl Pts',(29.6587300488869,0.656165051344154,-0.772850244059751));
#16594=CARTESIAN_POINT('Ctrl Pts',(29.6497459946103,0.552782663939933,-0.849064872504999));
#16595=CARTESIAN_POINT('Ctrl Pts',(29.6329401947329,0.340467534253599,-0.952477692807964));
#16596=CARTESIAN_POINT('Ctrl Pts',(29.6235614838323,0.213025964557654,-0.995444387176732));
#16597=CARTESIAN_POINT('Ctrl Pts',(29.6033554660083,-0.0701110249797902,
-1.01138590544986));
#16598=CARTESIAN_POINT('Ctrl Pts',(29.594136312248,-0.20089194460748,-0.993435412233449));
#16599=CARTESIAN_POINT('Ctrl Pts',(29.5754327036883,-0.449835071540499,
-0.909552155701649));
#16600=CARTESIAN_POINT('Ctrl Pts',(29.5661793807561,-0.564358031936759,
-0.843275682317829));
#16601=CARTESIAN_POINT('Ctrl Pts',(29.5472863312659,-0.763151979773412,
-0.667500700456543));
#16602=CARTESIAN_POINT('Ctrl Pts',(29.5378749975332,-0.845240586957616,
-0.560500408959181));
#16603=CARTESIAN_POINT('Ctrl Pts',(29.5177258575413,-0.970098454855238,
-0.306791753619133));
#16604=CARTESIAN_POINT('Ctrl Pts',(29.5085392150175,-0.995521631670878,
-0.177645971443525));
#16605=CARTESIAN_POINT('Ctrl Pts',(29.491952161989,-1.01157017614525,0.0548890692947026));
#16606=CARTESIAN_POINT('Ctrl Pts',(29.4824479630973,-0.998002528379827,
0.190430974375389));
#16607=CARTESIAN_POINT('Ctrl Pts',(29.4633399849439,-0.911379127216999,
0.444110884113391));
#16608=CARTESIAN_POINT('Ctrl Pts',(29.4543410303956,-0.847217927666079,
0.555636629667153));
#16609=CARTESIAN_POINT('Ctrl Pts',(29.4374952526998,-0.693921902387677,
0.736013762237563));
#16610=CARTESIAN_POINT('Ctrl Pts',(29.4281298191965,-0.594508302867161,
0.8262830850724));
#16611=CARTESIAN_POINT('Ctrl Pts',(29.4079318156156,-0.341677793262293,
0.954510297187121));
#16612=CARTESIAN_POINT('Ctrl Pts',(29.3986989741889,-0.214494381189009,
0.990633906486512));
#16613=CARTESIAN_POINT('Ctrl Pts',(29.3799881069202,0.0472837866910012,
1.01362569808423));
#16614=CARTESIAN_POINT('Ctrl Pts',(29.3707427007773,0.178646956831211,0.998775584332013));
#16615=CARTESIAN_POINT('Ctrl Pts',(29.3524577090853,0.42317016203226,0.920186008439517));
#16616=CARTESIAN_POINT('Ctrl Pts',(29.3436316170096,0.534424048498588,0.860636605924485));
#16617=CARTESIAN_POINT('Ctrl Pts',(29.3246540986636,0.742262305424851,0.694100403693534));
#16618=CARTESIAN_POINT('Ctrl Pts',(29.3158947475415,0.818004230287513,0.59447223902697));
#16619=CARTESIAN_POINT('Ctrl Pts',(29.3083604951404,0.8707720276777,0.502742051616109));
#16620=CARTESIAN_POINT('',(29.4766265292794,0.871221485734819,0.502999959546298));
#16621=CARTESIAN_POINT('',(29.47662653432,0.8712215562072,0.503));
#16622=CARTESIAN_POINT('Ctrl Pts',(30.9766395048596,-0.870772027677664,
0.502742051616115));
#16623=CARTESIAN_POINT('Ctrl Pts',(30.9691052524585,-0.818004230287503,
0.594472239026902));
#16624=CARTESIAN_POINT('Ctrl Pts',(30.9603459013364,-0.742262305424921,
0.694100403693345));
#16625=CARTESIAN_POINT('Ctrl Pts',(30.9413683829904,-0.534424048498782,
0.860636605924357));
#16626=CARTESIAN_POINT('Ctrl Pts',(30.9325422909147,-0.423170162032304,
0.920186008439501));
#16627=CARTESIAN_POINT('Ctrl Pts',(30.9142572992227,-0.178646956831084,
0.998775584332033));
#16628=CARTESIAN_POINT('Ctrl Pts',(30.9050118930798,-0.0472837866908874,
1.01362569808423));
#16629=CARTESIAN_POINT('Ctrl Pts',(30.8863010258111,0.214494381189104,0.990633906486492));
#16630=CARTESIAN_POINT('Ctrl Pts',(30.8770681843844,0.341677793262382,0.954510297187089));
#16631=CARTESIAN_POINT('Ctrl Pts',(30.8568701808035,0.594508302867236,0.826283085072347));
#16632=CARTESIAN_POINT('Ctrl Pts',(30.8475047473002,0.693921902387745,0.7360137622375));
#16633=CARTESIAN_POINT('Ctrl Pts',(30.8306589696044,0.847217927666129,0.555636629667076));
#16634=CARTESIAN_POINT('Ctrl Pts',(30.8216600150561,0.911379127217037,0.444110884113312));
#16635=CARTESIAN_POINT('Ctrl Pts',(30.8025520369027,0.998002528379825,0.190430974375358));
#16636=CARTESIAN_POINT('Ctrl Pts',(30.793047838011,1.01157017614526,0.0548890692946727));
#16637=CARTESIAN_POINT('Ctrl Pts',(30.7764607849825,0.995521631670864,-0.17764597144361));
#16638=CARTESIAN_POINT('Ctrl Pts',(30.7672741424587,0.970098454855212,-0.306791753619219));
#16639=CARTESIAN_POINT('Ctrl Pts',(30.7471250024668,0.845240586957565,-0.560500408959257));
#16640=CARTESIAN_POINT('Ctrl Pts',(30.7377136687341,0.763151979773352,-0.667500700456611));
#16641=CARTESIAN_POINT('Ctrl Pts',(30.7188206192439,0.564358031936684,-0.84327568231788));
#16642=CARTESIAN_POINT('Ctrl Pts',(30.7095672963117,0.449835071540419,-0.909552155701688));
#16643=CARTESIAN_POINT('Ctrl Pts',(30.690863687752,0.200891944607386,-0.993435412233469));
#16644=CARTESIAN_POINT('Ctrl Pts',(30.6816445339917,0.0701110249796861,
-1.01138590544987));
#16645=CARTESIAN_POINT('Ctrl Pts',(30.6614385161677,-0.213025964557793,
-0.995444387176709));
#16646=CARTESIAN_POINT('Ctrl Pts',(30.6520598052671,-0.34046753425376,-0.952477692807918));
#16647=CARTESIAN_POINT('Ctrl Pts',(30.6352540053897,-0.552782663940063,
-0.849064872504943));
#16648=CARTESIAN_POINT('Ctrl Pts',(30.6262699511131,-0.656165051344254,
-0.772850244059713));
#16649=CARTESIAN_POINT('Ctrl Pts',(30.6077447657717,-0.831881844612995,
-0.581371288177443));
#16650=CARTESIAN_POINT('Ctrl Pts',(30.5982393193793,-0.901486061152773,
-0.46433518258532));
#16651=CARTESIAN_POINT('Ctrl Pts',(30.5810552458603,-0.983138694974879,
-0.237085248117399));
#16652=CARTESIAN_POINT('Ctrl Pts',(30.5718646719207,-1.01164457155601,-0.108534779049151));
#16653=CARTESIAN_POINT('Ctrl Pts',(30.5517249713866,-0.999147204660936,
0.173834987272831));
#16654=CARTESIAN_POINT('Ctrl Pts',(30.542321718213,-0.967009114614643,0.304690319176143));
#16655=CARTESIAN_POINT('Ctrl Pts',(30.5234223525951,-0.855581407083066,
0.545608350968346));
#16656=CARTESIAN_POINT('Ctrl Pts',(30.5141578837074,-0.777163779775299,
0.652387656279837));
#16657=CARTESIAN_POINT('Ctrl Pts',(30.4954668431445,-0.582980235794573,
0.829064401206585));
#16658=CARTESIAN_POINT('Ctrl Pts',(30.4862599642795,-0.470601448908801,
0.897970498795622));
#16659=CARTESIAN_POINT('Ctrl Pts',(30.4660429991873,-0.204799025246621,
0.997222455929394));
#16660=CARTESIAN_POINT('Ctrl Pts',(30.4566507719092,-0.0706111542944245,
1.0089765786811));
#16661=CARTESIAN_POINT('Ctrl Pts',(30.4398838938875,0.164820890836542,0.999641820194012));
#16662=CARTESIAN_POINT('Ctrl Pts',(30.4309137064796,0.289920670515305,0.971492512618054));
#16663=CARTESIAN_POINT('Ctrl Pts',(30.4124152715538,0.527466569099329,0.867007573502016));
#16664=CARTESIAN_POINT('Ctrl Pts',(30.4029118555964,0.63830483856681,0.787948218222788));
#16665=CARTESIAN_POINT('Ctrl Pts',(30.3856873106528,0.804917354004856,0.612382577780553));
#16666=CARTESIAN_POINT('Ctrl Pts',(30.3764931007021,0.882667521494565,0.506058560714863));
#16667=CARTESIAN_POINT('Ctrl Pts',(30.3563616071713,0.984682436642579,0.242576766412225));
#16668=CARTESIAN_POINT('Ctrl Pts',(30.346965929091,1.00788845481734,0.109958040776825));
#16669=CARTESIAN_POINT('Ctrl Pts',(30.3280621443434,1.00280273292441,-0.155484472839195));
#16670=CARTESIAN_POINT('Ctrl Pts',(30.3187862830509,0.973839811222994,-0.284930092981143));
#16671=CARTESIAN_POINT('Ctrl Pts',(30.300107804091,0.86714400606165,-0.524617833052891));
#16672=CARTESIAN_POINT('Ctrl Pts',(30.2909121905272,0.792089695015476,-0.632780197940582));
#16673=CARTESIAN_POINT('Ctrl Pts',(30.2706842229679,0.588587875794973,-0.830697511597097));
#16674=CARTESIAN_POINT('Ctrl Pts',(30.2612794374791,0.470235006290619,-0.895430023340954));
#16675=CARTESIAN_POINT('Ctrl Pts',(30.2445489336977,0.251421288995111,-0.981433054835686));
#16676=CARTESIAN_POINT('Ctrl Pts',(30.2355913796315,0.12576520800403,-1.00599999999997));
#16677=CARTESIAN_POINT('Ctrl Pts',(30.2176616890085,-0.12576520800412,-1.00599999999996));
#16678=CARTESIAN_POINT('Ctrl Pts',(30.2087041349353,-0.251421288995197,
-0.981433054835669));
#16679=CARTESIAN_POINT('Ctrl Pts',(30.191973631154,-0.470235006290692,-0.895430023340922));
#16680=CARTESIAN_POINT('Ctrl Pts',(30.1825688456652,-0.588587875795032,
-0.830697511597059));
#16681=CARTESIAN_POINT('Ctrl Pts',(30.1623408781059,-0.792089695015518,
-0.632780197940532));
#16682=CARTESIAN_POINT('Ctrl Pts',(30.1531452645421,-0.867144006061684,
-0.524617833052833));
#16683=CARTESIAN_POINT('Ctrl Pts',(30.1344667855823,-0.973839811223013,
-0.284930092981069));
#16684=CARTESIAN_POINT('Ctrl Pts',(30.1251909242898,-1.00280273292442,-0.155484472839113));
#16685=CARTESIAN_POINT('Ctrl Pts',(30.1062871395422,-1.00788845481734,0.109958040776927));
#16686=CARTESIAN_POINT('Ctrl Pts',(30.0968914614619,-0.984682436642562,
0.242576766412345));
#16687=CARTESIAN_POINT('Ctrl Pts',(30.0767599679312,-0.882667521494528,
0.506058560714953));
#16688=CARTESIAN_POINT('Ctrl Pts',(30.0675657579804,-0.804917354004824,
0.61238257778061));
#16689=CARTESIAN_POINT('Ctrl Pts',(30.0503412130368,-0.63830483856678,0.787948218222807));
#16690=CARTESIAN_POINT('Ctrl Pts',(30.0408377970794,-0.527466569099297,
0.867007573502019));
#16691=CARTESIAN_POINT('Ctrl Pts',(30.0223393621535,-0.289920670515251,
0.971492512618062));
#16692=CARTESIAN_POINT('Ctrl Pts',(30.0133691747455,-0.164820890836456,
0.999641820194026));
#16693=CARTESIAN_POINT('Ctrl Pts',(29.9966022967237,0.0706111542945367,
1.00897657868109));
#16694=CARTESIAN_POINT('Ctrl Pts',(29.9872100694456,0.204799025246713,0.997222455929378));
#16695=CARTESIAN_POINT('Ctrl Pts',(29.9669931043534,0.470601448908866,0.89797049879559));
#16696=CARTESIAN_POINT('Ctrl Pts',(29.9577862254885,0.582980235794632,0.829064401206544));
#16697=CARTESIAN_POINT('Ctrl Pts',(29.9390951849257,0.777163779775341,0.652387656279782));
#16698=CARTESIAN_POINT('Ctrl Pts',(29.9298307160381,0.855581407083098,0.545608350968287));
#16699=CARTESIAN_POINT('Ctrl Pts',(29.9109313504203,0.967009114614655,0.304690319176081));
#16700=CARTESIAN_POINT('Ctrl Pts',(29.9015280972469,0.999147204660938,0.173834987272769));
#16701=CARTESIAN_POINT('Ctrl Pts',(29.8813883967129,1.01164457155599,-0.10853477904918));
#16702=CARTESIAN_POINT('Ctrl Pts',(29.8721978227732,0.983138694974849,-0.2370852481174));
#16703=CARTESIAN_POINT('Ctrl Pts',(29.8550137492541,0.901486061152735,-0.464335182585305));
#16704=CARTESIAN_POINT('Ctrl Pts',(29.8455083028615,0.831881844612943,-0.581371288177433));
#16705=CARTESIAN_POINT('Ctrl Pts',(29.82698311752,0.656165051344171,-0.772850244059737));
#16706=CARTESIAN_POINT('Ctrl Pts',(29.8179990632434,0.552782663939949,-0.849064872504989));
#16707=CARTESIAN_POINT('Ctrl Pts',(29.801193263366,0.340467534253614,-0.952477692807958));
#16708=CARTESIAN_POINT('Ctrl Pts',(29.7918145524654,0.21302596455767,-0.995444387176729));
#16709=CARTESIAN_POINT('Ctrl Pts',(29.7716085346413,-0.0701110249797728,
-1.01138590544987));
#16710=CARTESIAN_POINT('Ctrl Pts',(29.7623893808811,-0.200891944607462,
-0.993435412233453));
#16711=CARTESIAN_POINT('Ctrl Pts',(29.7436857723215,-0.44983507154048,-0.909552155701658));
#16712=CARTESIAN_POINT('Ctrl Pts',(29.7344324493892,-0.56435803193674,-0.843275682317841));
#16713=CARTESIAN_POINT('Ctrl Pts',(29.7155393998991,-0.763151979773394,
-0.667500700456562));
#16714=CARTESIAN_POINT('Ctrl Pts',(29.7061280661665,-0.845240586957599,
-0.560500408959205));
#16715=CARTESIAN_POINT('Ctrl Pts',(29.6859789261746,-0.97009845485523,-0.306791753619162));
#16716=CARTESIAN_POINT('Ctrl Pts',(29.6767922836507,-0.995521631670873,
-0.177645971443554));
#16717=CARTESIAN_POINT('Ctrl Pts',(29.6602052306221,-1.01157017614525,0.0548890692946818));
#16718=CARTESIAN_POINT('Ctrl Pts',(29.6507010317302,-0.99800252837983,0.190430974375375));
#16719=CARTESIAN_POINT('Ctrl Pts',(29.6315930535767,-0.911379127217004,
0.444110884113379));
#16720=CARTESIAN_POINT('Ctrl Pts',(29.6225940990285,-0.847217927666085,
0.555636629667144));
#16721=CARTESIAN_POINT('Ctrl Pts',(29.6057483213328,-0.693921902387682,
0.73601376223756));
#16722=CARTESIAN_POINT('Ctrl Pts',(29.5963828878296,-0.594508302867167,
0.826283085072396));
#16723=CARTESIAN_POINT('Ctrl Pts',(29.5761848842486,-0.341677793262302,
0.954510297187118));
#16724=CARTESIAN_POINT('Ctrl Pts',(29.5669520428219,-0.214494381189018,
0.99063390648651));
#16725=CARTESIAN_POINT('Ctrl Pts',(29.5482411755531,0.0472837866909914,
1.01362569808423));
#16726=CARTESIAN_POINT('Ctrl Pts',(29.5389957694103,0.178646956831203,0.998775584332015));
#16727=CARTESIAN_POINT('Ctrl Pts',(29.5207107777183,0.423170162032483,0.920186008439446));
#16728=CARTESIAN_POINT('Ctrl Pts',(29.5118846856427,0.534424048499014,0.860636605924257));
#16729=CARTESIAN_POINT('Ctrl Pts',(29.4929071645997,0.742262334961756,0.694100380026134));
#16730=CARTESIAN_POINT('Ctrl Pts',(29.4841478114739,0.818004270752247,0.594472186190298));
#16731=CARTESIAN_POINT('Ctrl Pts',(29.4766135577663,0.870772069751002,0.502741978476952));
#16732=CARTESIAN_POINT('Ctrl Pts',(31.16948943148,-1.281030538212,0.1346417350707));
#16733=CARTESIAN_POINT('Ctrl Pts',(31.15323943148,-1.250481297573,0.4252983443058));
#16734=CARTESIAN_POINT('Ctrl Pts',(31.12073943148,-0.9839217726285,0.9837339190898));
#16735=CARTESIAN_POINT('Ctrl Pts',(31.07198943148,-0.1454413688885,1.383873286175));
#16736=CARTESIAN_POINT('Ctrl Pts',(31.02323943148,0.7578368377583,1.166956165481));
#16737=CARTESIAN_POINT('Ctrl Pts',(30.97448943148,1.323348169458,0.429985043746));
#16738=CARTESIAN_POINT('Ctrl Pts',(30.92573943148,1.299030624161,-0.4986520486237));
#16739=CARTESIAN_POINT('Ctrl Pts',(30.87698943148,0.6957251488278,-1.205031028341));
#16740=CARTESIAN_POINT('Ctrl Pts',(30.82823943148,-0.2176707818353,-1.374319249677));
#16741=CARTESIAN_POINT('Ctrl Pts',(30.77948943148,-1.034049050162,-0.9310619315066));
#16742=CARTESIAN_POINT('Ctrl Pts',(30.73073943148,-1.38954331457,-0.07282288382614));
#16743=CARTESIAN_POINT('Ctrl Pts',(30.68198943148,-1.125706897575,0.8178739364602));
#16744=CARTESIAN_POINT('Ctrl Pts',(30.63323943148,-0.360133824607,1.344037730506));
#16745=CARTESIAN_POINT('Ctrl Pts',(30.58448943148,0.56595380301,1.271153053958));
#16746=CARTESIAN_POINT('Ctrl Pts',(30.53573943148,1.239791249317,0.6317051935655));
#16747=CARTESIAN_POINT('Ctrl Pts',(30.48698943148,1.361043721917,-0.2892987738068));
#16748=CARTESIAN_POINT('Ctrl Pts',(30.43823943148,0.8756680143869,-1.081359941037));
#16749=CARTESIAN_POINT('Ctrl Pts',(30.38948943148,-2.281508315605E-14,-1.3914502483));
#16750=CARTESIAN_POINT('Ctrl Pts',(30.34073943148,-0.8756680143869,-1.081359941037));
#16751=CARTESIAN_POINT('Ctrl Pts',(30.29198943148,-1.361043721917,-0.2892987738067));
#16752=CARTESIAN_POINT('Ctrl Pts',(30.24323943148,-1.239791249317,0.6317051935656));
#16753=CARTESIAN_POINT('Ctrl Pts',(30.19448943148,-0.56595380301,1.271153053958));
#16754=CARTESIAN_POINT('Ctrl Pts',(30.14573943148,0.360133824607,1.344037730506));
#16755=CARTESIAN_POINT('Ctrl Pts',(30.09698943148,1.125706897575,0.8178739364602));
#16756=CARTESIAN_POINT('Ctrl Pts',(30.04823943148,1.38954331457,-0.07282288382618));
#16757=CARTESIAN_POINT('Ctrl Pts',(29.99948943148,1.034049050162,-0.9310619315066));
#16758=CARTESIAN_POINT('Ctrl Pts',(29.95073943148,0.2176707818353,-1.374319249677));
#16759=CARTESIAN_POINT('Ctrl Pts',(29.90198943148,-0.6957251488278,-1.205031028341));
#16760=CARTESIAN_POINT('Ctrl Pts',(29.85323943148,-1.299030624161,-0.4986520486236));
#16761=CARTESIAN_POINT('Ctrl Pts',(29.80448943148,-1.323348169458,0.4299850437461));
#16762=CARTESIAN_POINT('Ctrl Pts',(29.75573943148,-0.7578368377582,1.166956165481));
#16763=CARTESIAN_POINT('Ctrl Pts',(29.70698943148,0.1454413688886,1.383873286175));
#16764=CARTESIAN_POINT('Ctrl Pts',(29.65823943148,0.9839217726285,0.9837339190898));
#16765=CARTESIAN_POINT('Ctrl Pts',(29.62573943148,1.250481297573,0.4252983443058));
#16766=CARTESIAN_POINT('Ctrl Pts',(29.60948943148,1.281030538212,0.1346417350707));
#16767=CARTESIAN_POINT('Ctrl Pts',(31.1078719886,-1.174890644721,0.1234859827342));
#16768=CARTESIAN_POINT('Ctrl Pts',(31.0916219886,-1.146872563997,0.3900602140506));
#16769=CARTESIAN_POINT('Ctrl Pts',(31.0591219886,-0.9023988510157,0.9022265620979));
#16770=CARTESIAN_POINT('Ctrl Pts',(31.0103719886,-0.1333908119794,1.269212348111));
#16771=CARTESIAN_POINT('Ctrl Pts',(30.9616219886,0.6950462025284,1.070267913782));
#16772=CARTESIAN_POINT('Ctrl Pts',(30.9128719886,1.213702045055,0.3943585966126));
#16773=CARTESIAN_POINT('Ctrl Pts',(30.8641219886,1.191399332028,-0.4573361909988));
#16774=CARTESIAN_POINT('Ctrl Pts',(30.8153719886,0.6380807828327,-1.105188080663));
#16775=CARTESIAN_POINT('Ctrl Pts',(30.7666219886,-0.1996356508131,-1.260449912114));
#16776=CARTESIAN_POINT('Ctrl Pts',(30.7178719886,-0.9483728287337,-0.8539187164967));
#16777=CARTESIAN_POINT('Ctrl Pts',(30.6691219886,-1.274412585824,-0.06678913763317));
#16778=CARTESIAN_POINT('Ctrl Pts',(30.6203719886,-1.032436357454,0.7501089223443));
#16779=CARTESIAN_POINT('Ctrl Pts',(30.5716219886,-0.3302949061378,1.232677370773));
#16780=CARTESIAN_POINT('Ctrl Pts',(30.5228719886,0.5190616528384,1.165831560259));
#16781=CARTESIAN_POINT('Ctrl Pts',(30.4741219886,1.137068240592,0.5793652063734));
#16782=CARTESIAN_POINT('Ctrl Pts',(30.4253719886,1.248274329329,-0.2653288994572));
#16783=CARTESIAN_POINT('Ctrl Pts',(30.3766219886,0.8031144670607,-0.9917637717473));
#16784=CARTESIAN_POINT('Ctrl Pts',(30.3278719886,-2.057218704603E-14,-1.276161520399));
#16785=CARTESIAN_POINT('Ctrl Pts',(30.2791219886,-0.8031144670608,-0.9917637717473));
#16786=CARTESIAN_POINT('Ctrl Pts',(30.2303719886,-1.248274329329,-0.2653288994572));
#16787=CARTESIAN_POINT('Ctrl Pts',(30.1816219886,-1.137068240592,0.5793652063734));
#16788=CARTESIAN_POINT('Ctrl Pts',(30.1328719886,-0.5190616528384,1.165831560259));
#16789=CARTESIAN_POINT('Ctrl Pts',(30.0841219886,0.3302949061378,1.232677370773));
#16790=CARTESIAN_POINT('Ctrl Pts',(30.0353719886,1.032436357454,0.7501089223443));
#16791=CARTESIAN_POINT('Ctrl Pts',(29.9866219886,1.274412585824,-0.06678913763321));
#16792=CARTESIAN_POINT('Ctrl Pts',(29.9378719886,0.9483728287337,-0.8539187164967));
#16793=CARTESIAN_POINT('Ctrl Pts',(29.8891219886,0.1996356508131,-1.260449912114));
#16794=CARTESIAN_POINT('Ctrl Pts',(29.8403719886,-0.6380807828327,-1.105188080663));
#16795=CARTESIAN_POINT('Ctrl Pts',(29.7916219886,-1.191399332028,-0.4573361909987));
#16796=CARTESIAN_POINT('Ctrl Pts',(29.7428719886,-1.213702045055,0.3943585966126));
#16797=CARTESIAN_POINT('Ctrl Pts',(29.6941219886,-0.6950462025284,1.070267913782));
#16798=CARTESIAN_POINT('Ctrl Pts',(29.6453719886,0.1333908119795,1.269212348111));
#16799=CARTESIAN_POINT('Ctrl Pts',(29.5966219886,0.9023988510157,0.9022265620978));
#16800=CARTESIAN_POINT('Ctrl Pts',(29.5641219886,1.146872563997,0.3900602140505));
#16801=CARTESIAN_POINT('Ctrl Pts',(29.5478719886,1.174890644721,0.1234859827342));
#16802=CARTESIAN_POINT('Ctrl Pts',(31.04625454572,-1.06875075123,0.1123302303977));
#16803=CARTESIAN_POINT('Ctrl Pts',(31.03000454572,-1.04326383042,0.3548220837953));
#16804=CARTESIAN_POINT('Ctrl Pts',(30.99750454572,-0.820875929403,0.8207192051059));
#16805=CARTESIAN_POINT('Ctrl Pts',(30.94875454572,-0.1213402550703,1.154551410048));
#16806=CARTESIAN_POINT('Ctrl Pts',(30.90000454572,0.6322555672986,0.9735796620828));
#16807=CARTESIAN_POINT('Ctrl Pts',(30.85125454572,1.104055920651,0.3587321494792));
#16808=CARTESIAN_POINT('Ctrl Pts',(30.80250454572,1.083768039895,-0.4160203333738));
#16809=CARTESIAN_POINT('Ctrl Pts',(30.75375454572,0.5804364168376,-1.005345132984));
#16810=CARTESIAN_POINT('Ctrl Pts',(30.70500454572,-0.1816005197909,-1.146580574552));
#16811=CARTESIAN_POINT('Ctrl Pts',(30.65625454572,-0.8626966073051,-0.7767755014867));
#16812=CARTESIAN_POINT('Ctrl Pts',(30.60750454572,-1.159281857079,-0.06075539144021));
#16813=CARTESIAN_POINT('Ctrl Pts',(30.55875454572,-0.9391658173332,0.6823439082283));
#16814=CARTESIAN_POINT('Ctrl Pts',(30.51000454572,-0.3004559876685,1.121317011041));
#16815=CARTESIAN_POINT('Ctrl Pts',(30.46125454572,0.4721695026668,1.060510066561));
#16816=CARTESIAN_POINT('Ctrl Pts',(30.41250454572,1.034345231867,0.5270252191813));
#16817=CARTESIAN_POINT('Ctrl Pts',(30.36375454572,1.135504936741,-0.2413590251076));
#16818=CARTESIAN_POINT('Ctrl Pts',(30.31500454572,0.7305609197345,-0.9021676024575));
#16819=CARTESIAN_POINT('Ctrl Pts',(30.26625454572,-1.95289898311E-14,-1.160872792498));
#16820=CARTESIAN_POINT('Ctrl Pts',(30.21750454572,-0.7305609197346,-0.9021676024575));
#16821=CARTESIAN_POINT('Ctrl Pts',(30.16875454572,-1.135504936741,-0.2413590251076));
#16822=CARTESIAN_POINT('Ctrl Pts',(30.12000454572,-1.034345231867,0.5270252191813));
#16823=CARTESIAN_POINT('Ctrl Pts',(30.07125454572,-0.4721695026667,1.060510066561));
#16824=CARTESIAN_POINT('Ctrl Pts',(30.02250454572,0.3004559876686,1.121317011041));
#16825=CARTESIAN_POINT('Ctrl Pts',(29.97375454572,0.9391658173332,0.6823439082283));
#16826=CARTESIAN_POINT('Ctrl Pts',(29.92500454572,1.159281857079,-0.06075539144025));
#16827=CARTESIAN_POINT('Ctrl Pts',(29.87625454572,0.8626966073051,-0.7767755014868));
#16828=CARTESIAN_POINT('Ctrl Pts',(29.82750454572,0.1816005197909,-1.146580574552));
#16829=CARTESIAN_POINT('Ctrl Pts',(29.77875454572,-0.5804364168377,-1.005345132984));
#16830=CARTESIAN_POINT('Ctrl Pts',(29.73000454572,-1.083768039895,-0.4160203333738));
#16831=CARTESIAN_POINT('Ctrl Pts',(29.68125454572,-1.104055920651,0.3587321494792));
#16832=CARTESIAN_POINT('Ctrl Pts',(29.63250454572,-0.6322555672985,0.9735796620828));
#16833=CARTESIAN_POINT('Ctrl Pts',(29.58375454572,0.1213402550704,1.154551410048));
#16834=CARTESIAN_POINT('Ctrl Pts',(29.53500454572,0.820875929403,0.8207192051059));
#16835=CARTESIAN_POINT('Ctrl Pts',(29.50250454572,1.04326383042,0.3548220837952));
#16836=CARTESIAN_POINT('Ctrl Pts',(29.48625454572,1.06875075123,0.1123302303976));
#16837=CARTESIAN_POINT('Ctrl Pts',(30.98463710284,-0.962610857739,0.1011744780611));
#16838=CARTESIAN_POINT('Ctrl Pts',(30.96838710284,-0.939655096844,0.31958395354));
#16839=CARTESIAN_POINT('Ctrl Pts',(30.93588710284,-0.7393530077902,0.739211848114));
#16840=CARTESIAN_POINT('Ctrl Pts',(30.88713710284,-0.1092896981613,1.039890471984));
#16841=CARTESIAN_POINT('Ctrl Pts',(30.83838710284,0.5694649320687,0.8768914103838));
#16842=CARTESIAN_POINT('Ctrl Pts',(30.78963710284,0.9944097962472,0.3231057023458));
#16843=CARTESIAN_POINT('Ctrl Pts',(30.74088710284,0.9761367477614,-0.3747044757489));
#16844=CARTESIAN_POINT('Ctrl Pts',(30.69213710284,0.5227920508426,-0.9055021853055));
#16845=CARTESIAN_POINT('Ctrl Pts',(30.64338710284,-0.1635653887687,-1.03271123699));
#16846=CARTESIAN_POINT('Ctrl Pts',(30.59463710284,-0.7770203858765,-0.6996322864768));
#16847=CARTESIAN_POINT('Ctrl Pts',(30.54588710284,-1.044151128333,-0.05472164524724));
#16848=CARTESIAN_POINT('Ctrl Pts',(30.49713710284,-0.8458952772121,0.6145788941124));
#16849=CARTESIAN_POINT('Ctrl Pts',(30.44838710284,-0.2706170691993,1.009956651308));
#16850=CARTESIAN_POINT('Ctrl Pts',(30.39963710284,0.4252773524951,0.9551885728626));
#16851=CARTESIAN_POINT('Ctrl Pts',(30.35088710284,0.9316222231427,0.4746852319892));
#16852=CARTESIAN_POINT('Ctrl Pts',(30.30213710284,1.022735544153,-0.2173891507581));
#16853=CARTESIAN_POINT('Ctrl Pts',(30.25338710284,0.6580073724084,-0.8125714331677));
#16854=CARTESIAN_POINT('Ctrl Pts',(30.20463710284,-1.731947918415E-14,-1.045584064598));
#16855=CARTESIAN_POINT('Ctrl Pts',(30.15588710284,-0.6580073724084,-0.8125714331677));
#16856=CARTESIAN_POINT('Ctrl Pts',(30.10713710284,-1.022735544153,-0.217389150758));
#16857=CARTESIAN_POINT('Ctrl Pts',(30.05838710284,-0.9316222231426,0.4746852319892));
#16858=CARTESIAN_POINT('Ctrl Pts',(30.00963710284,-0.4252773524951,0.9551885728626));
#16859=CARTESIAN_POINT('Ctrl Pts',(29.96088710284,0.2706170691994,1.009956651308));
#16860=CARTESIAN_POINT('Ctrl Pts',(29.91213710284,0.8458952772121,0.6145788941123));
#16861=CARTESIAN_POINT('Ctrl Pts',(29.86338710284,1.044151128333,-0.05472164524727));
#16862=CARTESIAN_POINT('Ctrl Pts',(29.81463710284,0.7770203858765,-0.6996322864768));
#16863=CARTESIAN_POINT('Ctrl Pts',(29.76588710284,0.1635653887687,-1.03271123699));
#16864=CARTESIAN_POINT('Ctrl Pts',(29.71713710284,-0.5227920508426,-0.9055021853054));
#16865=CARTESIAN_POINT('Ctrl Pts',(29.66838710284,-0.9761367477614,-0.3747044757489));
#16866=CARTESIAN_POINT('Ctrl Pts',(29.61963710284,-0.9944097962471,0.3231057023458));
#16867=CARTESIAN_POINT('Ctrl Pts',(29.57088710284,-0.5694649320687,0.8768914103838));
#16868=CARTESIAN_POINT('Ctrl Pts',(29.52213710284,0.1092896981613,1.039890471984));
#16869=CARTESIAN_POINT('Ctrl Pts',(29.47338710284,0.7393530077902,0.739211848114));
#16870=CARTESIAN_POINT('Ctrl Pts',(29.44088710284,0.939655096844,0.31958395354));
#16871=CARTESIAN_POINT('Ctrl Pts',(29.42463710284,0.962610857739,0.1011744780611));
#16872=CARTESIAN_POINT('',(29.6173426729392,1.08229570994162,0.624863717666542));
#16873=CARTESIAN_POINT('Ctrl Pts',(29.6176143539202,1.08217404411672,0.62477577113726));
#16874=CARTESIAN_POINT('Ctrl Pts',(29.624006078429,1.02692313633376,0.72095524840202));
#16875=CARTESIAN_POINT('Ctrl Pts',(29.6300982973051,0.959567950505402,0.80866689162659));
#16876=CARTESIAN_POINT('Ctrl Pts',(29.642405213234,0.805177359442618,0.961582228722831));
#16877=CARTESIAN_POINT('Ctrl Pts',(29.6486181844899,0.719600014745411,1.02676062670149));
#16878=CARTESIAN_POINT('Ctrl Pts',(29.6603920217373,0.544736432615982,1.12829523582901));
#16879=CARTESIAN_POINT('Ctrl Pts',(29.6659562556449,0.456650520588996,1.16701073503247));
#16880=CARTESIAN_POINT('Ctrl Pts',(29.677217232469,0.26753464102805,1.22524604638644));
#16881=CARTESIAN_POINT('Ctrl Pts',(29.6828002272489,0.166994080218219,1.24292681195758));
#16882=CARTESIAN_POINT('Ctrl Pts',(29.6933799224966,-0.0180241963746623,
1.25212919749128));
#16883=CARTESIAN_POINT('Ctrl Pts',(29.6982004972975,-0.101216694303839,
1.24795972121552));
#16884=CARTESIAN_POINT('Ctrl Pts',(29.7086891642604,-0.27942575559589,1.22150982604158));
#16885=CARTESIAN_POINT('Ctrl Pts',(29.7143622631559,-0.374099964090084,
1.19618207008826));
#16886=CARTESIAN_POINT('Ctrl Pts',(29.7258599403583,-0.56156923419032,1.1215657071463));
#16887=CARTESIAN_POINT('Ctrl Pts',(29.7315605712698,-0.652719320880998,
1.07105375242234));
#16888=CARTESIAN_POINT('Ctrl Pts',(29.7422685234012,-0.80378203686466,0.960235111854163));
#16889=CARTESIAN_POINT('Ctrl Pts',(29.7470893694736,-0.865691388100042,
0.904541514672143));
#16890=CARTESIAN_POINT('Ctrl Pts',(29.7575548795348,-0.987031922779028,
0.771912092007434));
#16891=CARTESIAN_POINT('Ctrl Pts',(29.7632039529513,-1.04433572334087,0.692883434585601));
#16892=CARTESIAN_POINT('Ctrl Pts',(29.7746485393149,-1.14248867363917,0.51757590484434));
#16893=CARTESIAN_POINT('Ctrl Pts',(29.7803228612616,-1.18132573215868,0.421387032124818));
#16894=CARTESIAN_POINT('Ctrl Pts',(29.7910025371398,-1.22890273220619,0.240666505206899));
#16895=CARTESIAN_POINT('Ctrl Pts',(29.7958233857595,-1.24198371349995,0.15842366891221));
#16896=CARTESIAN_POINT('Ctrl Pts',(29.8062905593356,-1.25285449382397,-0.0210353298026874));
#16897=CARTESIAN_POINT('Ctrl Pts',(29.8119413766803,-1.24766895484646,-0.118540271041648));
#16898=CARTESIAN_POINT('Ctrl Pts',(29.8233905058994,-1.21364125427389,-0.316621766311773));
#16899=CARTESIAN_POINT('Ctrl Pts',(29.8290672187053,-1.1832866023825,-0.415860313469128));
#16900=CARTESIAN_POINT('Ctrl Pts',(29.8397493384842,-1.10651941709313,-0.586291237802933));
#16901=CARTESIAN_POINT('Ctrl Pts',(29.8445701692025,-1.06493107988469,-0.65844035127944));
#16902=CARTESIAN_POINT('Ctrl Pts',(29.8550382895607,-0.960438444020922,
-0.804765872180896));
#16903=CARTESIAN_POINT('Ctrl Pts',(29.8606900786369,-0.895037104296968,
-0.877292185999977));
#16904=CARTESIAN_POINT('Ctrl Pts',(29.8721410937214,-0.743911877053629,
-1.00983818692771));
#16905=CARTESIAN_POINT('Ctrl Pts',(29.8778186927784,-0.657854911540548,
-1.0678657110005));
#16906=CARTESIAN_POINT('Ctrl Pts',(29.8885018175822,-0.490923110762975,
-1.15200547510011));
#16907=CARTESIAN_POINT('Ctrl Pts',(29.8933226556308,-0.413197385639256,
-1.18190074127503));
#16908=CARTESIAN_POINT('Ctrl Pts',(29.9037902621361,-0.239912892682437,
-1.22984962205128));
#16909=CARTESIAN_POINT('Ctrl Pts',(29.9094415211202,-0.143452590634435,
-1.24505123570626));
#16910=CARTESIAN_POINT('Ctrl Pts',(29.9208913119615,0.0573873184303584,
-1.2529493814113));
#16911=CARTESIAN_POINT('Ctrl Pts',(29.9265682655615,0.160772387954986,-1.2438890857129));
#16912=CARTESIAN_POINT('Ctrl Pts',(29.9372506771216,0.343442956077328,-1.20422974934481));
#16913=CARTESIAN_POINT('Ctrl Pts',(29.9420715140664,0.422661457005336,-1.17854950375753));
#16914=CARTESIAN_POINT('Ctrl Pts',(29.9525393204991,0.587508268981554,-1.10676239626014));
#16915=CARTESIAN_POINT('Ctrl Pts',(29.9581907845802,0.672042139416098,-1.05787108303544));
#16916=CARTESIAN_POINT('Ctrl Pts',(29.9696327050032,0.832984309871719,-0.937700574032089));
#16917=CARTESIAN_POINT('Ctrl Pts',(29.975302140758,0.907539604845622,-0.865708448776034));
#16918=CARTESIAN_POINT('Ctrl Pts',(29.9859759790889,1.02450658945619,-0.720077726497188));
#16919=CARTESIAN_POINT('Ctrl Pts',(29.9907968641008,1.06993512467627,-0.650278802855199));
#16920=CARTESIAN_POINT('Ctrl Pts',(30.0012686163419,1.15295219073745,-0.490715127389166));
#16921=CARTESIAN_POINT('Ctrl Pts',(30.0069240412507,1.18792592563569,-0.399467717681269));
#16922=CARTESIAN_POINT('Ctrl Pts',(30.0182537292321,1.23692421017922,-0.206718632695365));
#16923=CARTESIAN_POINT('Ctrl Pts',(30.0238150291331,1.2495831573343,-0.105894062156999));
#16924=CARTESIAN_POINT('Ctrl Pts',(30.0343650719903,1.24978013102473,0.0788946968053972));
#16925=CARTESIAN_POINT('Ctrl Pts',(30.03918647532,1.24155914322836,0.161818966878246));
#16926=CARTESIAN_POINT('Ctrl Pts',(30.049716193534,1.20631400859158,0.339223774572963));
#16927=CARTESIAN_POINT('Ctrl Pts',(30.0554300523819,1.17611645123081,0.433186524248501));
#16928=CARTESIAN_POINT('Ctrl Pts',(30.0675374387705,1.08773783421796,0.626353450277986));
#16929=CARTESIAN_POINT('Ctrl Pts',(30.0737661544201,1.02629079132724,0.722514395481912));
#16930=CARTESIAN_POINT('Ctrl Pts',(30.0850677301825,0.898311720065109,0.872323797899091));
#16931=CARTESIAN_POINT('Ctrl Pts',(30.0898826047594,0.838420345371865,0.929811830416312));
#16932=CARTESIAN_POINT('Ctrl Pts',(30.1001063454557,0.700551180287231,1.03858986657383));
#16933=CARTESIAN_POINT('Ctrl Pts',(30.1055166619412,0.621156618871846,1.08824415113204));
#16934=CARTESIAN_POINT('Ctrl Pts',(30.1155732472167,0.461535574094524,1.16461119456429));
#16935=CARTESIAN_POINT('Ctrl Pts',(30.1201846224814,0.382630077285512,1.19286944412205));
#16936=CARTESIAN_POINT('Ctrl Pts',(30.1303201759706,0.209221629354947,1.23560306157392));
#16937=CARTESIAN_POINT('Ctrl Pts',(30.1358277672504,0.114600498425028,1.24765599318599));
#16938=CARTESIAN_POINT('Ctrl Pts',(30.1461423243216,-0.0625593640511048,
1.2504209271504));
#16939=CARTESIAN_POINT('Ctrl Pts',(30.1509499487298,-0.145158645335778,
1.24370209826895));
#16940=CARTESIAN_POINT('Ctrl Pts',(30.1623960154908,-0.34138856704879,1.20803039925062));
#16941=CARTESIAN_POINT('Ctrl Pts',(30.1687600206973,-0.452098250127229,
1.17119579309478));
#16942=CARTESIAN_POINT('Ctrl Pts',(30.1812232769964,-0.6475609189281,1.0734199677459));
#16943=CARTESIAN_POINT('Ctrl Pts',(30.1871507413653,-0.732808811270244,
1.01681968518547));
#16944=CARTESIAN_POINT('Ctrl Pts',(30.1978846820031,-0.873249736341285,
0.897298777762955));
#16945=CARTESIAN_POINT('Ctrl Pts',(30.2026998467177,-0.931156847168942,
0.837385858829736));
#16946=CARTESIAN_POINT('Ctrl Pts',(30.2128560269344,-1.04160926343471,0.697460755129515));
#16947=CARTESIAN_POINT('Ctrl Pts',(30.2180744566332,-1.09152962316664,0.616422806085973));
#16948=CARTESIAN_POINT('Ctrl Pts',(30.2291153833449,-1.17343776603598,0.440598243640985));
#16949=CARTESIAN_POINT('Ctrl Pts',(30.2348633917994,-1.20439161560408,0.346197958887923));
#16950=CARTESIAN_POINT('Ctrl Pts',(30.2454211962973,-1.24064756275581,0.168513870520372));
#16951=CARTESIAN_POINT('Ctrl Pts',(30.2502356404206,-1.24929616484977,0.0857996286522642));
#16952=CARTESIAN_POINT('Ctrl Pts',(30.260845968283,-1.25015559790857,-0.0998540057624514));
#16953=CARTESIAN_POINT('Ctrl Pts',(30.2664618688018,-1.23783723726391,-0.201732441524374));
#16954=CARTESIAN_POINT('Ctrl Pts',(30.2779476142182,-1.18877368950535,-0.397420656303737));
#16955=CARTESIAN_POINT('Ctrl Pts',(30.2837121233972,-1.15320964302152,-0.490475139093015));
#16956=CARTESIAN_POINT('Ctrl Pts',(30.2942863118249,-1.069186562366,-0.651500670982716));
#16957=CARTESIAN_POINT('Ctrl Pts',(30.2991009718451,-1.02373608151537,-0.721167505274727));
#16958=CARTESIAN_POINT('Ctrl Pts',(30.3096647652641,-0.907811249820588,
-0.865207026839823));
#16959=CARTESIAN_POINT('Ctrl Pts',(30.3152394739193,-0.834627259119606,
-0.936040525954595));
#16960=CARTESIAN_POINT('Ctrl Pts',(30.3266764849137,-0.674053122419932,
-1.05677212531789));
#16961=CARTESIAN_POINT('Ctrl Pts',(30.3324367366807,-0.587930416894772,
-1.10669970892292));
#16962=CARTESIAN_POINT('Ctrl Pts',(30.3430067005688,-0.421391361778247,
-1.17899951718269));
#16963=CARTESIAN_POINT('Ctrl Pts',(30.3478213072528,-0.342241259312169,
-1.20456840716749));
#16964=CARTESIAN_POINT('Ctrl Pts',(30.3583968820281,-0.161331742712564,
-1.24367026121187));
#16965=CARTESIAN_POINT('Ctrl Pts',(30.3639820052499,-0.0596875303654986,
-1.25269824867541));
#16966=CARTESIAN_POINT('Ctrl Pts',(30.3754311781681,0.141292087509596,-1.24545325484622));
#16967=CARTESIAN_POINT('Ctrl Pts',(30.3811923531843,0.239656538131442,-1.23004619913465));
#16968=CARTESIAN_POINT('Ctrl Pts',(30.3917632379838,0.414592514073174,-1.18140765243432));
#16969=CARTESIAN_POINT('Ctrl Pts',(30.3965778600333,0.492192921487782,-1.15146040435034));
#16970=CARTESIAN_POINT('Ctrl Pts',(30.4071511642511,0.657352826866551,-1.06799972437164));
#16971=CARTESIAN_POINT('Ctrl Pts',(30.4127342974649,0.741992803185985,-1.01106594613429));
#16972=CARTESIAN_POINT('Ctrl Pts',(30.4241815875351,0.893598307086217,-0.878976891974612));
#16973=CARTESIAN_POINT('Ctrl Pts',(30.4299430228036,0.960348276783893,-0.805096992503565));
#16974=CARTESIAN_POINT('Ctrl Pts',(30.4405141518347,1.06569068887403,-0.657202158667046));
#16975=CARTESIAN_POINT('Ctrl Pts',(30.4453287636464,1.10715034993008,-0.585092594502051));
#16976=CARTESIAN_POINT('Ctrl Pts',(30.4559012674437,1.18297284107288,-0.416303633918732));
#16977=CARTESIAN_POINT('Ctrl Pts',(30.4614836780058,1.21291732983988,-0.318804555305318));
#16978=CARTESIAN_POINT('Ctrl Pts',(30.4729289349782,1.24760835985574,-0.12077840292281));
#16979=CARTESIAN_POINT('Ctrl Pts',(30.4786890924477,1.25299193291298,-0.0213780096235605));
#16980=CARTESIAN_POINT('Ctrl Pts',(30.4892589680672,1.24179913974343,0.159830349400949));
#16981=CARTESIAN_POINT('Ctrl Pts',(30.4940735898383,1.22864529584052,0.241961471557666));
#16982=CARTESIAN_POINT('Ctrl Pts',(30.5046456597338,1.18136362477796,0.420845888978654));
#16983=CARTESIAN_POINT('Ctrl Pts',(30.5102275079894,1.14328812854245,0.515456134887667));
#16984=CARTESIAN_POINT('Ctrl Pts',(30.5216724857142,1.04564032875421,0.691196105002304));
#16985=CARTESIAN_POINT('Ctrl Pts',(30.5274331889503,0.987267088029638,0.771848249436175));
#16986=CARTESIAN_POINT('Ctrl Pts',(30.5380037168126,0.86452950417065,0.905646658825268));
#16987=CARTESIAN_POINT('Ctrl Pts',(30.5428183824186,0.802624260369341,0.961199870112804));
#16988=CARTESIAN_POINT('Ctrl Pts',(30.5534132806734,0.653002216612035,1.07070080173363));
#16989=CARTESIAN_POINT('Ctrl Pts',(30.5590165680466,0.563515427790726,1.12041819426113));
#16990=CARTESIAN_POINT('Ctrl Pts',(30.5705013144578,0.376386750052923,1.19561757470478));
#16991=CARTESIAN_POINT('Ctrl Pts',(30.5762777298779,0.28000269287151,1.22151736339223));
#16992=CARTESIAN_POINT('Ctrl Pts',(30.5868629719407,0.100126080921217,1.24804271905387));
#16993=CARTESIAN_POINT('Ctrl Pts',(30.5916772320891,0.0170323540855195,
1.25213893207139));
#16994=CARTESIAN_POINT('Ctrl Pts',(30.6021452020552,-0.166049167240009,
1.24290134522974));
#16995=CARTESIAN_POINT('Ctrl Pts',(30.6076315893111,-0.264813429237742,
1.22568525623814));
#16996=CARTESIAN_POINT('Ctrl Pts',(30.6188947504349,-0.454317427207725,
1.16809897304761));
#16997=CARTESIAN_POINT('Ctrl Pts',(30.6245780697958,-0.544350438350243,
1.12865296595475));
#16998=CARTESIAN_POINT('Ctrl Pts',(30.6364550006192,-0.720622542665699,
1.02601904795267));
#16999=CARTESIAN_POINT('Ctrl Pts',(30.6426517477027,-0.805926829170602,
0.96092863891174));
#17000=CARTESIAN_POINT('Ctrl Pts',(30.6549281010291,-0.959862670245003,
0.808282316275064));
#17001=CARTESIAN_POINT('Ctrl Pts',(30.661007903792,-1.02704403086579,0.720744863512174));
#17002=CARTESIAN_POINT('Ctrl Pts',(30.6673856673726,-1.08217422817382,0.6247754507349));
#17003=CARTESIAN_POINT('',(29.6175,1.082531754731,0.625));
#17004=CARTESIAN_POINT('Ctrl Pts',(30.86036289716,-0.962610857739,0.1011744780611));
#17005=CARTESIAN_POINT('Ctrl Pts',(30.84411289716,-0.939655096844,0.31958395354));
#17006=CARTESIAN_POINT('Ctrl Pts',(30.81161289716,-0.7393530077902,0.739211848114));
#17007=CARTESIAN_POINT('Ctrl Pts',(30.76286289716,-0.1092896981613,1.039890471984));
#17008=CARTESIAN_POINT('Ctrl Pts',(30.71411289716,0.5694649320687,0.8768914103838));
#17009=CARTESIAN_POINT('Ctrl Pts',(30.66536289716,0.9944097962472,0.3231057023458));
#17010=CARTESIAN_POINT('Ctrl Pts',(30.61661289716,0.9761367477614,-0.3747044757489));
#17011=CARTESIAN_POINT('Ctrl Pts',(30.56786289716,0.5227920508426,-0.9055021853055));
#17012=CARTESIAN_POINT('Ctrl Pts',(30.51911289716,-0.1635653887687,-1.03271123699));
#17013=CARTESIAN_POINT('Ctrl Pts',(30.47036289716,-0.7770203858765,-0.6996322864768));
#17014=CARTESIAN_POINT('Ctrl Pts',(30.42161289716,-1.044151128333,-0.05472164524724));
#17015=CARTESIAN_POINT('Ctrl Pts',(30.37286289716,-0.8458952772121,0.6145788941124));
#17016=CARTESIAN_POINT('Ctrl Pts',(30.32411289716,-0.2706170691993,1.009956651308));
#17017=CARTESIAN_POINT('Ctrl Pts',(30.27536289716,0.4252773524951,0.9551885728626));
#17018=CARTESIAN_POINT('Ctrl Pts',(30.22661289716,0.9316222231427,0.4746852319892));
#17019=CARTESIAN_POINT('Ctrl Pts',(30.17786289716,1.022735544153,-0.2173891507581));
#17020=CARTESIAN_POINT('Ctrl Pts',(30.12911289716,0.6580073724084,-0.8125714331677));
#17021=CARTESIAN_POINT('Ctrl Pts',(30.08036289716,-1.726396803292E-14,-1.045584064598));
#17022=CARTESIAN_POINT('Ctrl Pts',(30.03161289716,-0.6580073724084,-0.8125714331677));
#17023=CARTESIAN_POINT('Ctrl Pts',(29.98286289716,-1.022735544153,-0.217389150758));
#17024=CARTESIAN_POINT('Ctrl Pts',(29.93411289716,-0.9316222231426,0.4746852319892));
#17025=CARTESIAN_POINT('Ctrl Pts',(29.88536289716,-0.4252773524951,0.9551885728626));
#17026=CARTESIAN_POINT('Ctrl Pts',(29.83661289716,0.2706170691994,1.009956651308));
#17027=CARTESIAN_POINT('Ctrl Pts',(29.78786289716,0.8458952772121,0.6145788941123));
#17028=CARTESIAN_POINT('Ctrl Pts',(29.73911289716,1.044151128333,-0.05472164524727));
#17029=CARTESIAN_POINT('Ctrl Pts',(29.69036289716,0.7770203858765,-0.6996322864768));
#17030=CARTESIAN_POINT('Ctrl Pts',(29.64161289716,0.1635653887687,-1.03271123699));
#17031=CARTESIAN_POINT('Ctrl Pts',(29.59286289716,-0.5227920508426,-0.9055021853054));
#17032=CARTESIAN_POINT('Ctrl Pts',(29.54411289716,-0.9761367477614,-0.3747044757489));
#17033=CARTESIAN_POINT('Ctrl Pts',(29.49536289716,-0.9944097962471,0.3231057023458));
#17034=CARTESIAN_POINT('Ctrl Pts',(29.44661289716,-0.5694649320687,0.8768914103838));
#17035=CARTESIAN_POINT('Ctrl Pts',(29.39786289716,0.1092896981613,1.039890471984));
#17036=CARTESIAN_POINT('Ctrl Pts',(29.34911289716,0.7393530077902,0.739211848114));
#17037=CARTESIAN_POINT('Ctrl Pts',(29.31661289716,0.939655096844,0.31958395354));
#17038=CARTESIAN_POINT('Ctrl Pts',(29.30036289716,0.962610857739,0.1011744780611));
#17039=CARTESIAN_POINT('Ctrl Pts',(30.79874545428,-1.06875075123,0.1123302303977));
#17040=CARTESIAN_POINT('Ctrl Pts',(30.78249545428,-1.04326383042,0.3548220837953));
#17041=CARTESIAN_POINT('Ctrl Pts',(30.74999545428,-0.820875929403,0.8207192051059));
#17042=CARTESIAN_POINT('Ctrl Pts',(30.70124545428,-0.1213402550703,1.154551410048));
#17043=CARTESIAN_POINT('Ctrl Pts',(30.65249545428,0.6322555672986,0.9735796620828));
#17044=CARTESIAN_POINT('Ctrl Pts',(30.60374545428,1.104055920651,0.3587321494792));
#17045=CARTESIAN_POINT('Ctrl Pts',(30.55499545428,1.083768039895,-0.4160203333738));
#17046=CARTESIAN_POINT('Ctrl Pts',(30.50624545428,0.5804364168376,-1.005345132984));
#17047=CARTESIAN_POINT('Ctrl Pts',(30.45749545428,-0.1816005197909,-1.146580574552));
#17048=CARTESIAN_POINT('Ctrl Pts',(30.40874545428,-0.8626966073051,-0.7767755014867));
#17049=CARTESIAN_POINT('Ctrl Pts',(30.35999545428,-1.159281857079,-0.0607553914402));
#17050=CARTESIAN_POINT('Ctrl Pts',(30.31124545428,-0.9391658173332,0.6823439082283));
#17051=CARTESIAN_POINT('Ctrl Pts',(30.26249545428,-0.3004559876685,1.121317011041));
#17052=CARTESIAN_POINT('Ctrl Pts',(30.21374545428,0.4721695026668,1.060510066561));
#17053=CARTESIAN_POINT('Ctrl Pts',(30.16499545428,1.034345231867,0.5270252191813));
#17054=CARTESIAN_POINT('Ctrl Pts',(30.11624545428,1.135504936741,-0.2413590251076));
#17055=CARTESIAN_POINT('Ctrl Pts',(30.06749545428,0.7305609197345,-0.9021676024575));
#17056=CARTESIAN_POINT('Ctrl Pts',(30.01874545428,-1.947954876406E-14,-1.160872792498));
#17057=CARTESIAN_POINT('Ctrl Pts',(29.96999545428,-0.7305609197346,-0.9021676024575));
#17058=CARTESIAN_POINT('Ctrl Pts',(29.92124545428,-1.135504936741,-0.2413590251076));
#17059=CARTESIAN_POINT('Ctrl Pts',(29.87249545428,-1.034345231867,0.5270252191813));
#17060=CARTESIAN_POINT('Ctrl Pts',(29.82374545428,-0.4721695026667,1.060510066561));
#17061=CARTESIAN_POINT('Ctrl Pts',(29.77499545428,0.3004559876686,1.121317011041));
#17062=CARTESIAN_POINT('Ctrl Pts',(29.72624545428,0.9391658173332,0.6823439082283));
#17063=CARTESIAN_POINT('Ctrl Pts',(29.67749545428,1.159281857079,-0.06075539144024));
#17064=CARTESIAN_POINT('Ctrl Pts',(29.62874545428,0.8626966073051,-0.7767755014868));
#17065=CARTESIAN_POINT('Ctrl Pts',(29.57999545428,0.1816005197909,-1.146580574552));
#17066=CARTESIAN_POINT('Ctrl Pts',(29.53124545428,-0.5804364168377,-1.005345132984));
#17067=CARTESIAN_POINT('Ctrl Pts',(29.48249545428,-1.083768039895,-0.4160203333738));
#17068=CARTESIAN_POINT('Ctrl Pts',(29.43374545428,-1.104055920651,0.3587321494792));
#17069=CARTESIAN_POINT('Ctrl Pts',(29.38499545428,-0.6322555672985,0.9735796620828));
#17070=CARTESIAN_POINT('Ctrl Pts',(29.33624545428,0.1213402550704,1.154551410048));
#17071=CARTESIAN_POINT('Ctrl Pts',(29.28749545428,0.820875929403,0.8207192051059));
#17072=CARTESIAN_POINT('Ctrl Pts',(29.25499545428,1.04326383042,0.3548220837952));
#17073=CARTESIAN_POINT('Ctrl Pts',(29.23874545428,1.06875075123,0.1123302303976));
#17074=CARTESIAN_POINT('Ctrl Pts',(30.7371280114,-1.174890644721,0.1234859827342));
#17075=CARTESIAN_POINT('Ctrl Pts',(30.7208780114,-1.146872563997,0.3900602140506));
#17076=CARTESIAN_POINT('Ctrl Pts',(30.6883780114,-0.9023988510157,0.9022265620979));
#17077=CARTESIAN_POINT('Ctrl Pts',(30.6396280114,-0.1333908119794,1.269212348111));
#17078=CARTESIAN_POINT('Ctrl Pts',(30.5908780114,0.6950462025284,1.070267913782));
#17079=CARTESIAN_POINT('Ctrl Pts',(30.5421280114,1.213702045055,0.3943585966126));
#17080=CARTESIAN_POINT('Ctrl Pts',(30.4933780114,1.191399332028,-0.4573361909988));
#17081=CARTESIAN_POINT('Ctrl Pts',(30.4446280114,0.6380807828327,-1.105188080663));
#17082=CARTESIAN_POINT('Ctrl Pts',(30.3958780114,-0.1996356508131,-1.260449912114));
#17083=CARTESIAN_POINT('Ctrl Pts',(30.3471280114,-0.9483728287337,-0.8539187164967));
#17084=CARTESIAN_POINT('Ctrl Pts',(30.2983780114,-1.274412585824,-0.06678913763317));
#17085=CARTESIAN_POINT('Ctrl Pts',(30.2496280114,-1.032436357454,0.7501089223443));
#17086=CARTESIAN_POINT('Ctrl Pts',(30.2008780114,-0.3302949061378,1.232677370773));
#17087=CARTESIAN_POINT('Ctrl Pts',(30.1521280114,0.5190616528384,1.165831560259));
#17088=CARTESIAN_POINT('Ctrl Pts',(30.1033780114,1.137068240592,0.5793652063734));
#17089=CARTESIAN_POINT('Ctrl Pts',(30.0546280114,1.248274329329,-0.2653288994572));
#17090=CARTESIAN_POINT('Ctrl Pts',(30.0058780114,0.8031144670607,-0.9917637717473));
#17091=CARTESIAN_POINT('Ctrl Pts',(29.9571280114,-1.980022061951E-14,-1.276161520399));
#17092=CARTESIAN_POINT('Ctrl Pts',(29.9083780114,-0.8031144670608,-0.9917637717473));
#17093=CARTESIAN_POINT('Ctrl Pts',(29.8596280114,-1.248274329329,-0.2653288994572));
#17094=CARTESIAN_POINT('Ctrl Pts',(29.8108780114,-1.137068240592,0.5793652063734));
#17095=CARTESIAN_POINT('Ctrl Pts',(29.7621280114,-0.5190616528384,1.165831560259));
#17096=CARTESIAN_POINT('Ctrl Pts',(29.7133780114,0.3302949061378,1.232677370773));
#17097=CARTESIAN_POINT('Ctrl Pts',(29.6646280114,1.032436357454,0.7501089223443));
#17098=CARTESIAN_POINT('Ctrl Pts',(29.6158780114,1.274412585824,-0.06678913763322));
#17099=CARTESIAN_POINT('Ctrl Pts',(29.5671280114,0.9483728287337,-0.8539187164967));
#17100=CARTESIAN_POINT('Ctrl Pts',(29.5183780114,0.1996356508131,-1.260449912114));
#17101=CARTESIAN_POINT('Ctrl Pts',(29.4696280114,-0.6380807828327,-1.105188080663));
#17102=CARTESIAN_POINT('Ctrl Pts',(29.4208780114,-1.191399332028,-0.4573361909987));
#17103=CARTESIAN_POINT('Ctrl Pts',(29.3721280114,-1.213702045055,0.3943585966126));
#17104=CARTESIAN_POINT('Ctrl Pts',(29.3233780114,-0.6950462025284,1.070267913782));
#17105=CARTESIAN_POINT('Ctrl Pts',(29.2746280114,0.1333908119795,1.269212348111));
#17106=CARTESIAN_POINT('Ctrl Pts',(29.2258780114,0.9023988510157,0.9022265620978));
#17107=CARTESIAN_POINT('Ctrl Pts',(29.1933780114,1.146872563997,0.3900602140505));
#17108=CARTESIAN_POINT('Ctrl Pts',(29.1771280114,1.174890644721,0.1234859827342));
#17109=CARTESIAN_POINT('Ctrl Pts',(30.67551056852,-1.281030538212,0.1346417350707));
#17110=CARTESIAN_POINT('Ctrl Pts',(30.65926056852,-1.250481297573,0.4252983443058));
#17111=CARTESIAN_POINT('Ctrl Pts',(30.62676056852,-0.9839217726285,0.9837339190898));
#17112=CARTESIAN_POINT('Ctrl Pts',(30.57801056852,-0.1454413688885,1.383873286175));
#17113=CARTESIAN_POINT('Ctrl Pts',(30.52926056852,0.7578368377583,1.166956165481));
#17114=CARTESIAN_POINT('Ctrl Pts',(30.48051056852,1.323348169458,0.429985043746));
#17115=CARTESIAN_POINT('Ctrl Pts',(30.43176056852,1.299030624161,-0.4986520486237));
#17116=CARTESIAN_POINT('Ctrl Pts',(30.38301056852,0.6957251488278,-1.205031028341));
#17117=CARTESIAN_POINT('Ctrl Pts',(30.33426056852,-0.2176707818353,-1.374319249677));
#17118=CARTESIAN_POINT('Ctrl Pts',(30.28551056852,-1.034049050162,-0.9310619315066));
#17119=CARTESIAN_POINT('Ctrl Pts',(30.23676056852,-1.38954331457,-0.07282288382613));
#17120=CARTESIAN_POINT('Ctrl Pts',(30.18801056852,-1.125706897575,0.8178739364602));
#17121=CARTESIAN_POINT('Ctrl Pts',(30.13926056852,-0.360133824607,1.344037730506));
#17122=CARTESIAN_POINT('Ctrl Pts',(30.09051056852,0.56595380301,1.271153053958));
#17123=CARTESIAN_POINT('Ctrl Pts',(30.04176056852,1.239791249317,0.6317051935655));
#17124=CARTESIAN_POINT('Ctrl Pts',(29.99301056852,1.361043721917,-0.2892987738068));
#17125=CARTESIAN_POINT('Ctrl Pts',(29.94426056852,0.8756680143869,-1.081359941037));
#17126=CARTESIAN_POINT('Ctrl Pts',(29.89551056852,-2.198241588758E-14,-1.3914502483));
#17127=CARTESIAN_POINT('Ctrl Pts',(29.84676056852,-0.875668014387,-1.081359941037));
#17128=CARTESIAN_POINT('Ctrl Pts',(29.79801056852,-1.361043721917,-0.2892987738067));
#17129=CARTESIAN_POINT('Ctrl Pts',(29.74926056852,-1.239791249317,0.6317051935656));
#17130=CARTESIAN_POINT('Ctrl Pts',(29.70051056852,-0.56595380301,1.271153053958));
#17131=CARTESIAN_POINT('Ctrl Pts',(29.65176056852,0.360133824607,1.344037730506));
#17132=CARTESIAN_POINT('Ctrl Pts',(29.60301056852,1.125706897575,0.8178739364602));
#17133=CARTESIAN_POINT('Ctrl Pts',(29.55426056852,1.38954331457,-0.07282288382619));
#17134=CARTESIAN_POINT('Ctrl Pts',(29.50551056852,1.034049050162,-0.9310619315066));
#17135=CARTESIAN_POINT('Ctrl Pts',(29.45676056852,0.2176707818353,-1.374319249677));
#17136=CARTESIAN_POINT('Ctrl Pts',(29.40801056852,-0.6957251488278,-1.205031028341));
#17137=CARTESIAN_POINT('Ctrl Pts',(29.35926056852,-1.299030624161,-0.4986520486236));
#17138=CARTESIAN_POINT('Ctrl Pts',(29.31051056852,-1.323348169458,0.4299850437461));
#17139=CARTESIAN_POINT('Ctrl Pts',(29.26176056852,-0.7578368377582,1.166956165481));
#17140=CARTESIAN_POINT('Ctrl Pts',(29.21301056852,0.1454413688886,1.383873286175));
#17141=CARTESIAN_POINT('Ctrl Pts',(29.16426056852,0.9839217726285,0.9837339190898));
#17142=CARTESIAN_POINT('Ctrl Pts',(29.13176056852,1.250481297573,0.4252983443058));
#17143=CARTESIAN_POINT('Ctrl Pts',(29.11551056852,1.281030538212,0.1346417350707));
#17144=CARTESIAN_POINT('',(29.1676573270715,1.08229570837247,0.624863720396445));
#17145=CARTESIAN_POINT('Ctrl Pts',(29.617627341968,1.08215501597624,0.62476352113272));
#17146=CARTESIAN_POINT('Ctrl Pts',(29.61459741681,1.10800857523719,0.579922158874817));
#17147=CARTESIAN_POINT('Ctrl Pts',(29.6115421791637,1.13109114492466,0.533476323136956));
#17148=CARTESIAN_POINT('Ctrl Pts',(29.5979044654554,1.22146502968022,0.319487471057165));
#17149=CARTESIAN_POINT('Ctrl Pts',(29.5888599482143,1.24922762750675,0.153891219598247));
#17150=CARTESIAN_POINT('Ctrl Pts',(29.5737847077041,1.24989879330249,-0.113832666126114));
#17151=CARTESIAN_POINT('Ctrl Pts',(29.5669031019519,1.23354843079392,-0.230222265136776));
#17152=CARTESIAN_POINT('Ctrl Pts',(29.5560364877087,1.18303861956897,-0.407985503133046));
#17153=CARTESIAN_POINT('Ctrl Pts',(29.5520249813698,1.15886534353969,-0.472541576903855));
#17154=CARTESIAN_POINT('Ctrl Pts',(29.5426236328536,1.08803886439693,-0.622208331795665));
#17155=CARTESIAN_POINT('Ctrl Pts',(29.5373144435947,1.03646342659019,-0.704760379661174));
#17156=CARTESIAN_POINT('Ctrl Pts',(29.5252776000949,0.902890623340095,-0.871840292472444));
#17157=CARTESIAN_POINT('Ctrl Pts',(29.5183993972978,0.81711148767936,-0.952400105380579));
#17158=CARTESIAN_POINT('Ctrl Pts',(29.5072903013536,0.662900641104247,-1.06168646706383));
#17159=CARTESIAN_POINT('Ctrl Pts',(29.5030466274329,0.599916290928708,-1.09861661506134));
#17160=CARTESIAN_POINT('Ctrl Pts',(29.4935499634098,0.448370282102632,-1.17026616405347));
#17161=CARTESIAN_POINT('Ctrl Pts',(29.4883511300327,0.358178885242108,-1.20093403070587));
#17162=CARTESIAN_POINT('Ctrl Pts',(29.4764216575478,0.151089332425558,-1.2459862887354));
#17163=CARTESIAN_POINT('Ctrl Pts',(29.4695340008344,0.0336386874856851,
-1.25443381468143));
#17164=CARTESIAN_POINT('Ctrl Pts',(29.4585602097506,-0.152648874215112,
-1.24216397620102));
#17165=CARTESIAN_POINT('Ctrl Pts',(29.4544538449471,-0.222473817675357,
-1.23166981758508));
#17166=CARTESIAN_POINT('Ctrl Pts',(29.4450136136811,-0.384335500019739,
-1.19293104198071));
#17167=CARTESIAN_POINT('Ctrl Pts',(29.4397494515913,-0.474974442137163,
-1.15981399212218));
#17168=CARTESIAN_POINT('Ctrl Pts',(29.4277636106627,-0.665321913901319,
-1.06424838874914));
#17169=CARTESIAN_POINT('Ctrl Pts',(29.4208892753518,-0.761865224190842,
-0.997128445216505));
#17170=CARTESIAN_POINT('Ctrl Pts',(29.4097593639183,-0.901053681731414,
-0.868778241319131));
#17171=CARTESIAN_POINT('Ctrl Pts',(29.4054913512447,-0.950524419006847,
-0.814508791853337));
#17172=CARTESIAN_POINT('Ctrl Pts',(29.3959883691584,-1.05205634969515,-0.68094437448249));
#17173=CARTESIAN_POINT('Ctrl Pts',(29.3908045259822,-1.10059723896093,-0.599309120618603));
#17174=CARTESIAN_POINT('Ctrl Pts',(29.3801568761226,-1.17827835703337,-0.426851826779456));
#17175=CARTESIAN_POINT('Ctrl Pts',(29.3746502745195,-1.20704346491738,-0.336466924104589));
#17176=CARTESIAN_POINT('Ctrl Pts',(29.3649862290562,-1.2390999636105,-0.1754160308971));
#17177=CARTESIAN_POINT('Ctrl Pts',(29.3608584555161,-1.24704808336017,-0.105612279761285));
#17178=CARTESIAN_POINT('Ctrl Pts',(29.3527448374063,-1.25115038739277,0.0351003553259205));
#17179=CARTESIAN_POINT('Ctrl Pts',(29.3487973845041,-1.24713429538041,0.105792904140653));
#17180=CARTESIAN_POINT('Ctrl Pts',(29.3387661503307,-1.22182615116716,0.284089728846796));
#17181=CARTESIAN_POINT('Ctrl Pts',(29.3326747356135,-1.19237958602683,0.389730367717767));
#17182=CARTESIAN_POINT('Ctrl Pts',(29.3175510069523,-1.09049746262549,0.62776530071626));
#17183=CARTESIAN_POINT('Ctrl Pts',(29.3076789663981,-1.0003923014378,0.771310551286882));
#17184=CARTESIAN_POINT('Ctrl Pts',(29.2940075376696,-0.823883953792329,
0.941501666280569));
#17185=CARTESIAN_POINT('Ctrl Pts',(29.2906548112083,-0.77732146047511,0.980307422285116));
#17186=CARTESIAN_POINT('Ctrl Pts',(29.282259797587,-0.656399188471644,1.06700328117913));
#17187=CARTESIAN_POINT('Ctrl Pts',(29.2771202228619,-0.579432598450008,
1.11052953944549));
#17188=CARTESIAN_POINT('Ctrl Pts',(29.2652769550014,-0.394863984399084,
1.19087511045753));
#17189=CARTESIAN_POINT('Ctrl Pts',(29.2586205770142,-0.284696785371201,
1.22212264404173));
#17190=CARTESIAN_POINT('Ctrl Pts',(29.2476722995244,-0.0914843826785107,
1.24889940201236));
#17191=CARTESIAN_POINT('Ctrl Pts',(29.243215154838,-0.010336908285927,1.25220705415618));
#17192=CARTESIAN_POINT('Ctrl Pts',(29.2332417528454,0.16616149197302,1.24223431935585));
#17193=CARTESIAN_POINT('Ctrl Pts',(29.2276409552425,0.260829710909366,1.22568679187361));
#17194=CARTESIAN_POINT('Ctrl Pts',(29.2159304610313,0.451611747274278,1.169601699981));
#17195=CARTESIAN_POINT('Ctrl Pts',(29.2098673387471,0.547347851324356,1.12817256922947));
#17196=CARTESIAN_POINT('Ctrl Pts',(29.1953702495661,0.769260145843567,0.996707303011102));
#17197=CARTESIAN_POINT('Ctrl Pts',(29.1862505178116,0.897634598070124,0.887573424797484));
#17198=CARTESIAN_POINT('Ctrl Pts',(29.172937791388,1.03241317167635,0.705446011550095));
#17199=CARTESIAN_POINT('Ctrl Pts',(29.1701446500545,1.05843702892822,0.665787836578457));
#17200=CARTESIAN_POINT('Ctrl Pts',(29.1673726659358,1.0821385210664,0.624792090993702));
#17201=CARTESIAN_POINT('',(29.30837346568,0.8712215562072,0.503));
#17202=CARTESIAN_POINT('Ctrl Pts',(29.36036289716,0.5689250970851,0.7830582177302));
#17203=CARTESIAN_POINT('Ctrl Pts',(29.34411289716,0.7465953708295,0.6539732078924));
#17204=CARTESIAN_POINT('Ctrl Pts',(29.31161289716,1.00985274314,0.2706925630537));
#17205=CARTESIAN_POINT('Ctrl Pts',(29.26286289716,0.9552164149722,-0.4252975810125));
#17206=CARTESIAN_POINT('Ctrl Pts',(29.21411289716,0.4746777717184,-0.9316168029278));
#17207=CARTESIAN_POINT('Ctrl Pts',(29.16536289716,-0.2173871517845,-1.022736996495));
#17208=CARTESIAN_POINT('Ctrl Pts',(29.11661289716,-0.812571968791,-0.6580069832544));
#17209=CARTESIAN_POINT('Ctrl Pts',(29.06786289716,-1.045583921078,-1.042734902035E-7));
#17210=CARTESIAN_POINT('Ctrl Pts',(29.01911289716,-0.8125714716224,0.6580074003485));
#17211=CARTESIAN_POINT('Ctrl Pts',(28.97036289716,-0.2173891404584,1.022735536666));
#17212=CARTESIAN_POINT('Ctrl Pts',(28.92161289716,0.4746852292457,0.9316222251505));
#17213=CARTESIAN_POINT('Ctrl Pts',(28.87286289716,0.9551885735371,0.4252773519507));
#17214=CARTESIAN_POINT('Ctrl Pts',(28.82411289716,1.009956651354,-0.2706170690297));
#17215=CARTESIAN_POINT('Ctrl Pts',(28.77536289716,0.614578893256,-0.8458952773463));
#17216=CARTESIAN_POINT('Ctrl Pts',(28.72661289716,-0.0547216418674,-1.044151127966));
#17217=CARTESIAN_POINT('Ctrl Pts',(28.67786289716,-0.69963229914,-0.7770203872106));
#17218=CARTESIAN_POINT('Ctrl Pts',(28.62911289716,-1.032711189717,-0.1635653837992));
#17219=CARTESIAN_POINT('Ctrl Pts',(28.58036289716,-0.9055023617337,0.5227920322988));
#17220=CARTESIAN_POINT('Ctrl Pts',(28.53161289716,-0.3747038173085,0.9761368169669));
#17221=CARTESIAN_POINT('Ctrl Pts',(28.48286289716,0.3231032450129,0.9944095379687));
#17222=CARTESIAN_POINT('Ctrl Pts',(28.43411289716,0.8769005812753,0.5694658959771));
#17223=CARTESIAN_POINT('Ctrl Pts',(28.38536289716,1.039856245751,-0.1092932955163));
#17224=CARTESIAN_POINT('Ctrl Pts',(28.33661289716,0.7393395821542,-0.7393395822784));
#17225=CARTESIAN_POINT('Ctrl Pts',(28.28786289716,0.109293296325,-1.039856246063));
#17226=CARTESIAN_POINT('Ctrl Pts',(28.23911289716,-0.5694658990877,-0.8769005799032));
#17227=CARTESIAN_POINT('Ctrl Pts',(28.19036289716,-0.994409526335,-0.323103250189));
#17228=CARTESIAN_POINT('Ctrl Pts',(28.14161289716,-0.9761368603912,0.3747038366413));
#17229=CARTESIAN_POINT('Ctrl Pts',(28.09286289716,-0.5227918702355,0.905502289579));
#17230=CARTESIAN_POINT('Ctrl Pts',(28.04411289716,0.1635647789705,1.032711459003));
#17231=CARTESIAN_POINT('Ctrl Pts',(27.99536289716,0.7770226444627,0.6996312941492));
#17232=CARTESIAN_POINT('Ctrl Pts',(27.94661289716,1.044142703787,0.05472539254393));
#17233=CARTESIAN_POINT('Ctrl Pts',(27.89786289716,0.845926716811,-0.6145928909717));
#17234=CARTESIAN_POINT('Ctrl Pts',(27.84911289716,0.27049973535,-1.009904411168));
#17235=CARTESIAN_POINT('Ctrl Pts',(27.81661289716,-0.1930597260145,-0.9735571614325));
#17236=CARTESIAN_POINT('Ctrl Pts',(27.80036289716,-0.393685760654,-0.8842326957913));
#17237=CARTESIAN_POINT('Ctrl Pts',(29.29874545428,0.6316562087523,0.86940018568));
#17238=CARTESIAN_POINT('Ctrl Pts',(29.28249545428,0.8289168536007,0.7260819380959));
#17239=CARTESIAN_POINT('Ctrl Pts',(29.24999545428,1.121201645697,0.3005398056651));
#17240=CARTESIAN_POINT('Ctrl Pts',(29.20124545428,1.060540978612,-0.4721919616313));
#17241=CARTESIAN_POINT('Ctrl Pts',(29.15249545428,0.5270169363223,-1.034339214006));
#17242=CARTESIAN_POINT('Ctrl Pts',(29.10374545428,-0.2413568057223,-1.135506549222));
#17243=CARTESIAN_POINT('Ctrl Pts',(29.05499545428,-0.9021681971399,-0.7305604876715));
#17244=CARTESIAN_POINT('Ctrl Pts',(29.00624545428,-1.160872633154,-1.157709476594E-7));
#17245=CARTESIAN_POINT('Ctrl Pts',(28.95749545428,-0.9021676451524,0.7305609507555));
#17246=CARTESIAN_POINT('Ctrl Pts',(28.90874545428,-0.2413590136723,1.135504928428));
#17247=CARTESIAN_POINT('Ctrl Pts',(28.85999545428,0.5270252161353,1.034345234097));
#17248=CARTESIAN_POINT('Ctrl Pts',(28.81124545428,1.06051006731,0.4721695020623));
#17249=CARTESIAN_POINT('Ctrl Pts',(28.76249545428,1.121317011091,-0.3004559874803));
#17250=CARTESIAN_POINT('Ctrl Pts',(28.71374545428,0.6823439072775,-0.9391658174822));
#17251=CARTESIAN_POINT('Ctrl Pts',(28.66499545428,-0.0607553876877,-1.159281856671));
#17252=CARTESIAN_POINT('Ctrl Pts',(28.61624545428,-0.7767755155462,-0.8626966087863));
#17253=CARTESIAN_POINT('Ctrl Pts',(28.56749545428,-1.146580522067,-0.1816005142735));
#17254=CARTESIAN_POINT('Ctrl Pts',(28.51874545428,-1.005345328866,0.5804363962492));
#17255=CARTESIAN_POINT('Ctrl Pts',(28.46999545428,-0.4160196023322,1.083768116731));
#17256=CARTESIAN_POINT('Ctrl Pts',(28.42124545428,0.3587294211946,1.104055633894));
#17257=CARTESIAN_POINT('Ctrl Pts',(28.37249545428,0.9735898441798,0.6322566374899));
#17258=CARTESIAN_POINT('Ctrl Pts',(28.32374545428,1.154513409944,-0.1213442490789));
#17259=CARTESIAN_POINT('Ctrl Pts',(28.27499545428,0.8208610234226,-0.8208610235605));
#17260=CARTESIAN_POINT('Ctrl Pts',(28.22624545428,0.1213442499766,-1.154513410291));
#17261=CARTESIAN_POINT('Ctrl Pts',(28.17749545428,-0.6322566409435,-0.9735898426565));
#17262=CARTESIAN_POINT('Ctrl Pts',(28.12874545428,-1.104055620977,-0.3587294269414));
#17263=CARTESIAN_POINT('Ctrl Pts',(28.07999545428,-1.083768164943,0.4160196237967));
#17264=CARTESIAN_POINT('Ctrl Pts',(28.03124545428,-0.5804362163164,1.005345248755));
#17265=CARTESIAN_POINT('Ctrl Pts',(27.98249545428,0.1815998427548,1.146580821045));
#17266=CARTESIAN_POINT('Ctrl Pts',(27.93374545428,0.8626991149286,0.7767743997426));
#17267=CARTESIAN_POINT('Ctrl Pts',(27.88499545428,1.159272503621,0.06075955192325));
#17268=CARTESIAN_POINT('Ctrl Pts',(27.83624545428,0.9392007235413,-0.6823594484165));
#17269=CARTESIAN_POINT('Ctrl Pts',(27.78749545428,0.300325716294,-1.121259010771));
#17270=CARTESIAN_POINT('Ctrl Pts',(27.75499545428,-0.2143469768198,-1.080904021891));
#17271=CARTESIAN_POINT('Ctrl Pts',(27.73874545428,-0.4370945424777,-0.9817304160776));
#17272=CARTESIAN_POINT('Ctrl Pts',(29.2371280114,0.6943873204196,0.9557421536299));
#17273=CARTESIAN_POINT('Ctrl Pts',(29.2208780114,0.9112383363718,0.7981906682994));
#17274=CARTESIAN_POINT('Ctrl Pts',(29.1883780114,1.232550548254,0.3303870482765));
#17275=CARTESIAN_POINT('Ctrl Pts',(29.1396280114,1.165865542251,-0.5190863422501));
#17276=CARTESIAN_POINT('Ctrl Pts',(29.0908780114,0.5793561009262,-1.137061625084));
#17277=CARTESIAN_POINT('Ctrl Pts',(29.0421280114,-0.26532645966,-1.248276101949));
#17278=CARTESIAN_POINT('Ctrl Pts',(28.9933780114,-0.9917644254889,-0.8031139920886));
#17279=CARTESIAN_POINT('Ctrl Pts',(28.9446280114,-1.27616134523,-1.272684035096E-7));
#17280=CARTESIAN_POINT('Ctrl Pts',(28.8958780114,-0.9917638186823,0.8031145011624));
#17281=CARTESIAN_POINT('Ctrl Pts',(28.8471280114,-0.2653288868863,1.248274320191));
#17282=CARTESIAN_POINT('Ctrl Pts',(28.7983780114,0.5793652030249,1.137068243043));
#17283=CARTESIAN_POINT('Ctrl Pts',(28.7496280114,1.165831561083,0.5190616521739));
#17284=CARTESIAN_POINT('Ctrl Pts',(28.7008780114,1.232677370829,-0.3302949059308));
#17285=CARTESIAN_POINT('Ctrl Pts',(28.6521280114,0.7501089212991,-1.032436357618));
#17286=CARTESIAN_POINT('Ctrl Pts',(28.6033780114,-0.066789133508,-1.274412585376));
#17287=CARTESIAN_POINT('Ctrl Pts',(28.5546280114,-0.8539187319524,-0.948372830362));
#17288=CARTESIAN_POINT('Ctrl Pts',(28.5058780114,-1.260449854417,-0.1996356447477));
#17289=CARTESIAN_POINT('Ctrl Pts',(28.4571280114,-1.105188295998,0.6380807601996));
#17290=CARTESIAN_POINT('Ctrl Pts',(28.4083780114,-0.4573353873558,1.191399416495));
#17291=CARTESIAN_POINT('Ctrl Pts',(28.3596280114,0.3943555973763,1.213701729819));
#17292=CARTESIAN_POINT('Ctrl Pts',(28.3108780114,1.070279107084,0.6950473790027));
#17293=CARTESIAN_POINT('Ctrl Pts',(28.2621280114,1.269170574137,-0.1333952026414));
#17294=CARTESIAN_POINT('Ctrl Pts',(28.2133780114,0.9023824646909,-0.9023824648426));
#17295=CARTESIAN_POINT('Ctrl Pts',(28.1646280114,0.1333952036283,-1.269170574518));
#17296=CARTESIAN_POINT('Ctrl Pts',(28.1158780114,-0.6950473827993,-1.07027910541));
#17297=CARTESIAN_POINT('Ctrl Pts',(28.0671280114,-1.21370171562,-0.3943556036939));
#17298=CARTESIAN_POINT('Ctrl Pts',(28.0183780114,-1.191399469495,0.457335410952));
#17299=CARTESIAN_POINT('Ctrl Pts',(27.9696280114,-0.6380805623973,1.105188207931));
#17300=CARTESIAN_POINT('Ctrl Pts',(27.9208780114,0.1996349065391,1.260450183087));
#17301=CARTESIAN_POINT('Ctrl Pts',(27.8721280114,0.9483755853946,0.853917505336));
#17302=CARTESIAN_POINT('Ctrl Pts',(27.8233780114,1.274402303455,0.06679371130257));
#17303=CARTESIAN_POINT('Ctrl Pts',(27.7746280114,1.032474730272,-0.7501260058614));
#17304=CARTESIAN_POINT('Ctrl Pts',(27.7258780114,0.3301516972379,-1.232613610374));
#17305=CARTESIAN_POINT('Ctrl Pts',(27.6933780114,-0.2356342276251,-1.18825088235));
#17306=CARTESIAN_POINT('Ctrl Pts',(27.6771280114,-0.4805033243014,-1.079228136364));
#17307=CARTESIAN_POINT('Ctrl Pts',(29.17551056852,0.7571184320868,1.04208412158));
#17308=CARTESIAN_POINT('Ctrl Pts',(29.15926056852,0.9935598191429,0.8702993985028));
#17309=CARTESIAN_POINT('Ctrl Pts',(29.12676056852,1.34389945081,0.3602342908879));
#17310=CARTESIAN_POINT('Ctrl Pts',(29.07801056852,1.271190105891,-0.5659807228689));
#17311=CARTESIAN_POINT('Ctrl Pts',(29.02926056852,0.6316952655301,-1.239784036163));
#17312=CARTESIAN_POINT('Ctrl Pts',(28.98051056852,-0.2892961135977,-1.361045654676));
#17313=CARTESIAN_POINT('Ctrl Pts',(28.93176056852,-1.081360653838,-0.8756674965057));
#17314=CARTESIAN_POINT('Ctrl Pts',(28.88301056852,-1.391450057306,-1.387658609686E-7));
#17315=CARTESIAN_POINT('Ctrl Pts',(28.83426056852,-1.081359992212,0.8756680515693));
#17316=CARTESIAN_POINT('Ctrl Pts',(28.78551056852,-0.2892987601002,1.361043711953));
#17317=CARTESIAN_POINT('Ctrl Pts',(28.73676056852,0.6317051899145,1.239791251989));
#17318=CARTESIAN_POINT('Ctrl Pts',(28.68801056852,1.271153054855,0.5659538022855));
#17319=CARTESIAN_POINT('Ctrl Pts',(28.63926056852,1.344037730566,-0.3601338243813));
#17320=CARTESIAN_POINT('Ctrl Pts',(28.59051056852,0.8178739353206,-1.125706897754));
#17321=CARTESIAN_POINT('Ctrl Pts',(28.54176056852,-0.07282287932829,-1.389543314081));
#17322=CARTESIAN_POINT('Ctrl Pts',(28.49301056852,-0.9310619483587,-1.034049051938));
#17323=CARTESIAN_POINT('Ctrl Pts',(28.44426056852,-1.374319186766,-0.217670775222));
#17324=CARTESIAN_POINT('Ctrl Pts',(28.39551056852,-1.20503126313,0.69572512415));
#17325=CARTESIAN_POINT('Ctrl Pts',(28.34676056852,-0.4986511723795,1.299030716259));
#17326=CARTESIAN_POINT('Ctrl Pts',(28.29801056852,0.429981773558,1.323347825744));
#17327=CARTESIAN_POINT('Ctrl Pts',(28.24926056852,1.166968369989,0.7578381205155));
#17328=CARTESIAN_POINT('Ctrl Pts',(28.20051056852,1.383827738331,-0.1454461562039));
#17329=CARTESIAN_POINT('Ctrl Pts',(28.15176056852,0.9839039059593,-0.9839039061246));
#17330=CARTESIAN_POINT('Ctrl Pts',(28.10301056852,0.14544615728,-1.383827738746));
#17331=CARTESIAN_POINT('Ctrl Pts',(28.05426056852,-0.7578381246551,-1.166968368163));
#17332=CARTESIAN_POINT('Ctrl Pts',(28.00551056852,-1.323347810262,-0.4299817804463));
#17333=CARTESIAN_POINT('Ctrl Pts',(27.95676056852,-1.299030774048,0.4986511981073));
#17334=CARTESIAN_POINT('Ctrl Pts',(27.90801056852,-0.6957249084782,1.205031167107));
#17335=CARTESIAN_POINT('Ctrl Pts',(27.85926056852,0.2176699703234,1.374319545129));
#17336=CARTESIAN_POINT('Ctrl Pts',(27.81051056852,1.034052055861,0.9310606109294));
#17337=CARTESIAN_POINT('Ctrl Pts',(27.76176056852,1.389532103288,0.07282787068189));
#17338=CARTESIAN_POINT('Ctrl Pts',(27.71301056852,1.125748737002,-0.8178925633062));
#17339=CARTESIAN_POINT('Ctrl Pts',(27.66426056852,0.3599776781819,-1.343968209978));
#17340=CARTESIAN_POINT('Ctrl Pts',(27.63176056852,-0.2569214784304,-1.295597742809));
#17341=CARTESIAN_POINT('Ctrl Pts',(27.61551056852,-0.5239121061251,-1.17672585665));
#17342=CARTESIAN_POINT('',(28.1173426729269,-1.58041447686304E-9,-1.24972743805679));
#17343=CARTESIAN_POINT('Ctrl Pts',(29.1673856727373,1.08215847935993,0.62480272807601));
#17344=CARTESIAN_POINT('Ctrl Pts',(29.1609968231379,1.13780188993381,0.528907476598624));
#17345=CARTESIAN_POINT('Ctrl Pts',(29.1549070070917,1.18007293410309,0.426766710488715));
#17346=CARTESIAN_POINT('Ctrl Pts',(29.1426003915839,1.23533098518457,0.216609270813267));
#17347=CARTESIAN_POINT('Ctrl Pts',(29.1363846186847,1.24900067471773,0.10985972163656));
#17348=CARTESIAN_POINT('Ctrl Pts',(29.1246079782619,1.24950055350375,-0.0923920289181761));
#17349=CARTESIAN_POINT('Ctrl Pts',(29.1190437443542,1.23898620331935,-0.188034416051438));
#17350=CARTESIAN_POINT('Ctrl Pts',(29.1077827675308,1.19486152256845,-0.380931227675969));
#17351=CARTESIAN_POINT('Ctrl Pts',(29.1021997727515,1.15990323431047,-0.476842290222699));
#17352=CARTESIAN_POINT('Ctrl Pts',(29.0916200775045,1.07536359566911,-0.641674010674401));
#17353=CARTESIAN_POINT('Ctrl Pts',(29.0867995027036,1.03015647433006,-0.711636089148229));
#17354=CARTESIAN_POINT('Ctrl Pts',(29.0763108357406,0.918145662537286,-0.852744715826819));
#17355=CARTESIAN_POINT('Ctrl Pts',(29.0706377368451,0.84887407821414,-0.92207110749063));
#17356=CARTESIAN_POINT('Ctrl Pts',(29.0591400596422,0.690519777313731,-1.04711607636201));
#17357=CARTESIAN_POINT('Ctrl Pts',(29.0534394287303,0.601200097976828,-1.10079838963519));
#17358=CARTESIAN_POINT('Ctrl Pts',(29.0427314765985,0.42969698203359,-1.17621321895953));
#17359=CARTESIAN_POINT('Ctrl Pts',(29.0379106305261,0.350510236428156,-1.2019814912698));
#17360=CARTESIAN_POINT('Ctrl Pts',(29.027445120465,0.174979519771536,-1.2407507654775));
#17361=CARTESIAN_POINT('Ctrl Pts',(29.0217960470484,0.0778867945362808,
-1.2508629837861));
#17362=CARTESIAN_POINT('Ctrl Pts',(29.0103514606849,-0.123010454843654,
-1.24821216732928));
#17363=CARTESIAN_POINT('Ctrl Pts',(29.0046771387381,-0.225730991439992,
-1.23375161025516));
#17364=CARTESIAN_POINT('Ctrl Pts',(28.9939974628599,-0.406028058759957,
-1.18459423747219));
#17365=CARTESIAN_POINT('Ctrl Pts',(28.9891766142402,-0.483792934917113,
-1.15480128143127));
#17366=CARTESIAN_POINT('Ctrl Pts',(28.9787094406642,-0.644644376902829,
-1.07448615399293));
#17367=CARTESIAN_POINT('Ctrl Pts',(28.9730586233196,-0.726493363520805,
-1.02124287488659));
#17368=CARTESIAN_POINT('Ctrl Pts',(28.9616094940918,-0.881023120274798,
-0.892733274025263));
#17369=CARTESIAN_POINT('Ctrl Pts',(28.9559327812777,-0.951788897290975,
-0.816826100660987));
#17370=CARTESIAN_POINT('Ctrl Pts',(28.9452506614896,-1.06100281474115,-0.665128305694781));
#17371=CARTESIAN_POINT('Ctrl Pts',(28.9404298307713,-1.10269161124056,-0.593037192421202));
#17372=CARTESIAN_POINT('Ctrl Pts',(28.9299617104173,-1.17716691154411,-0.429381154843096));
#17373=CARTESIAN_POINT('Ctrl Pts',(28.9243099213453,-1.20727587184561,-0.336478776348865));
#17374=CARTESIAN_POINT('Ctrl Pts',(28.9128589053545,-1.24650146526412,-0.139327474322873));
#17375=CARTESIAN_POINT('Ctrl Pts',(28.9071813054504,-1.25372629152159,-0.0357861780207992));
#17376=CARTESIAN_POINT('Ctrl Pts',(28.8964981796817,-1.24312755625725,0.150850899382122));
#17377=CARTESIAN_POINT('Ctrl Pts',(28.8916773416385,-1.23015475067021,0.233110984081));
#17378=CARTESIAN_POINT('Ctrl Pts',(28.8812097355702,-1.18503744856303,0.407154188490358));
#17379=CARTESIAN_POINT('Ctrl Pts',(28.8755584770246,-1.14997228120041,0.498292059529182));
#17380=CARTESIAN_POINT('Ctrl Pts',(28.8641085952306,-1.05639157416792,0.676175007538576));
#17381=CARTESIAN_POINT('Ctrl Pts',(28.8584315565826,-0.99685151062749,0.761180141227436));
#17382=CARTESIAN_POINT('Ctrl Pts',(28.8477490481642,-0.871168646274408,
0.899548501056932));
#17383=CARTESIAN_POINT('Ctrl Pts',(28.8429282117568,-0.809319472973177,
0.955313355727054));
#17384=CARTESIAN_POINT('Ctrl Pts',(28.8324604491855,-0.664726825936106,
1.0621803476943));
#17385=CARTESIAN_POINT('Ctrl Pts',(28.8268090291305,-0.580119269771693,
1.11094256397802));
#17386=CARTESIAN_POINT('Ctrl Pts',(28.8153608141088,-0.39547571549497,1.19028059577321));
#17387=CARTESIAN_POINT('Ctrl Pts',(28.8096854796079,-0.295740972270812,
1.21886789376563));
#17388=CARTESIAN_POINT('Ctrl Pts',(28.799004920911,-0.111022478533813,1.24731595871076));
#17389=CARTESIAN_POINT('Ctrl Pts',(28.7941840725387,-0.0278621866324802,
1.25173710673691));
#17390=CARTESIAN_POINT('Ctrl Pts',(28.783715371199,0.151777824311083,1.24380664271366));
#17391=CARTESIAN_POINT('Ctrl Pts',(28.7780630096127,0.248233768235987,1.22846011416248));
#17392=CARTESIAN_POINT('Ctrl Pts',(28.7666688661819,0.440745046189595,1.17418381083944));
#17393=CARTESIAN_POINT('Ctrl Pts',(28.761044729133,0.535411455001453,1.13412624208424));
#17394=CARTESIAN_POINT('Ctrl Pts',(28.7504226043197,0.696271670037493,1.0408417898367));
#17395=CARTESIAN_POINT('Ctrl Pts',(28.745601465636,0.763811970201196,0.99208242969822));
#17396=CARTESIAN_POINT('Ctrl Pts',(28.7351059230236,0.89904284123568,0.872862932852518));
#17397=CARTESIAN_POINT('Ctrl Pts',(28.7294265690749,0.964772407202923,0.800013145469062));
#17398=CARTESIAN_POINT('Ctrl Pts',(28.7175549018527,1.08524523589081,0.630024828488589));
#17399=CARTESIAN_POINT('Ctrl Pts',(28.7115121987401,1.13646338425354,0.531967497284216));
#17400=CARTESIAN_POINT('Ctrl Pts',(28.7004178235523,1.20231572056898,0.349876761132139));
#17401=CARTESIAN_POINT('Ctrl Pts',(28.6956005072857,1.22270420461145,0.269312521838998));
#17402=CARTESIAN_POINT('Ctrl Pts',(28.6853025041299,1.24928400747707,0.0944403346743677));
#17403=CARTESIAN_POINT('Ctrl Pts',(28.6798196179985,1.25311307280083,-0.000329806078066004));
#17404=CARTESIAN_POINT('Ctrl Pts',(28.6698538536718,1.24023256691938,-0.175075399992849));
#17405=CARTESIAN_POINT('Ctrl Pts',(28.6654023964275,1.22637185852316,-0.254673920123353));
#17406=CARTESIAN_POINT('Ctrl Pts',(28.656120254182,1.18250126169467,-0.412630540184733));
#17407=CARTESIAN_POINT('Ctrl Pts',(28.651308721134,1.15211009650188,-0.490484077956556));
#17408=CARTESIAN_POINT('Ctrl Pts',(28.6402791571121,1.06621272285659,-0.659611041467915));
#17409=CARTESIAN_POINT('Ctrl Pts',(28.6340423593765,1.0059787604408,-0.748625224630084));
#17410=CARTESIAN_POINT('Ctrl Pts',(28.6235704314111,0.88491755396491,-0.885925058168001));
#17411=CARTESIAN_POINT('Ctrl Pts',(28.619341299677,0.829489182644027,-0.938117904947043));
#17412=CARTESIAN_POINT('Ctrl Pts',(28.6056416940033,0.637217189292378,-1.0880523872875));
#17413=CARTESIAN_POINT('Ctrl Pts',(28.5964663934893,0.493873124613629,-1.1564816575457));
#17414=CARTESIAN_POINT('Ctrl Pts',(28.5832571271695,0.275857378970494,-1.22144536570823));
#17415=CARTESIAN_POINT('Ctrl Pts',(28.5784836206256,0.194162861610605,-1.23735031895491));
#17416=CARTESIAN_POINT('Ctrl Pts',(28.5681687583255,0.0118748310926331,
-1.25389771722638));
#17417=CARTESIAN_POINT('Ctrl Pts',(28.5626389226762,-0.0880714154939871,
-1.25071016360653));
#17418=CARTESIAN_POINT('Ctrl Pts',(28.5495790029823,-0.312377603319782,
-1.21620261797431));
#17419=CARTESIAN_POINT('Ctrl Pts',(28.5421259172881,-0.434727227617343,
-1.17797308587252));
#17420=CARTESIAN_POINT('Ctrl Pts',(28.5259541327221,-0.686696704182463,
-1.05550036517512));
#17421=CARTESIAN_POINT('Ctrl Pts',(28.5176743220364,-0.809974980446674,
-0.964339063317631));
#17422=CARTESIAN_POINT('Ctrl Pts',(28.5018915255945,-0.996684232313097,
-0.762897639913671));
#17423=CARTESIAN_POINT('Ctrl Pts',(28.4947884408799,-1.06605194740329,-0.662310901274681));
#17424=CARTESIAN_POINT('Ctrl Pts',(28.478242069081,-1.19332547341186,-0.406321486463468));
#17425=CARTESIAN_POINT('Ctrl Pts',(28.4693392709946,-1.23647935954279,-0.246852651704806));
#17426=CARTESIAN_POINT('Ctrl Pts',(28.4527491629305,-1.25466077156035,0.0411246745072808));
#17427=CARTESIAN_POINT('Ctrl Pts',(28.445519723942,-1.24435020038222,0.165043891084873));
#17428=CARTESIAN_POINT('Ctrl Pts',(28.4289027367094,-1.17940926325769,0.444977178094289));
#17429=CARTESIAN_POINT('Ctrl Pts',(28.4200489075221,-1.11165294241514,0.594751104676615));
#17430=CARTESIAN_POINT('Ctrl Pts',(28.4032467279876,-0.940922001055101,
0.831567809637354));
#17431=CARTESIAN_POINT('Ctrl Pts',(28.3957655905894,-0.850859018249042,
0.923455894554462));
#17432=CARTESIAN_POINT('Ctrl Pts',(28.379695000864,-0.628378280453494,1.09092775812837));
#17433=CARTESIAN_POINT('Ctrl Pts',(28.3715266034993,-0.493160971631295,
1.15851365987721));
#17434=CARTESIAN_POINT('Ctrl Pts',(28.3559740940566,-0.23287888310737,1.23319870860315));
#17435=CARTESIAN_POINT('Ctrl Pts',(28.3489751243855,-0.113607696680456,
1.24971763753644));
#17436=CARTESIAN_POINT('Ctrl Pts',(28.3324939596632,0.170943447329841,1.24898130791147));
#17437=CARTESIAN_POINT('Ctrl Pts',(28.3235539903221,0.333427313594694,1.21608692054995));
#17438=CARTESIAN_POINT('Ctrl Pts',(28.3071454749248,0.596307822609007,1.10431561727585));
#17439=CARTESIAN_POINT('Ctrl Pts',(28.3001230430521,0.699661147036682,1.04176253692698));
#17440=CARTESIAN_POINT('Ctrl Pts',(28.283626841901,0.920268908395139,0.861552091487536));
#17441=CARTESIAN_POINT('Ctrl Pts',(28.2746953841206,1.02554613396491,0.733653396596494));
#17442=CARTESIAN_POINT('Ctrl Pts',(28.2582441863208,1.15945745744885,0.480551291001781));
#17443=CARTESIAN_POINT('Ctrl Pts',(28.2511735069117,1.20042346896607,0.366020576549046));
#17444=CARTESIAN_POINT('Ctrl Pts',(28.2346450095893,1.25765576767662,0.08631348627535));
#17445=CARTESIAN_POINT('Ctrl Pts',(28.2257275433854,1.25842963526239,-0.079101086624162));
#17446=CARTESIAN_POINT('Ctrl Pts',(28.2091729460902,1.20209026283813,-0.361504893424582));
#17447=CARTESIAN_POINT('Ctrl Pts',(28.2019899388488,1.16064213771058,-0.477888717818062));
#17448=CARTESIAN_POINT('Ctrl Pts',(28.1854044491616,1.02666889684467,-0.731427854742207));
#17449=CARTESIAN_POINT('Ctrl Pts',(28.1765426400489,0.922762085626656,-0.859122704134831));
#17450=CARTESIAN_POINT('Ctrl Pts',(28.1599441436812,0.699673347662511,-1.04230381455487));
#17451=CARTESIAN_POINT('Ctrl Pts',(28.1526754229846,0.592495098195602,-1.10666724822368));
#17452=CARTESIAN_POINT('Ctrl Pts',(28.1360033505331,0.3264006252068,-1.21762615967261));
#17453=CARTESIAN_POINT('Ctrl Pts',(28.1271255168001,0.165037419574197,-1.2499368389208));
#17454=CARTESIAN_POINT('Ctrl Pts',(28.1176143326274,-1.57020897636201E-5,
-1.249578098287));
#17455=CARTESIAN_POINT('',(27.6676389699633,5.88637870807089E-8,-1.24975677572573));
#17456=CARTESIAN_POINT('Ctrl Pts',(28.1176273340642,-1.65623511105583E-5,
-1.24955549515429));
#17457=CARTESIAN_POINT('Ctrl Pts',(28.114597434561,-0.0517766618297808,
-1.24952464781677));
#17458=CARTESIAN_POINT('Ctrl Pts',(28.111542222149,-0.103540795931321,-1.24629187069692));
#17459=CARTESIAN_POINT('Ctrl Pts',(28.0979036849824,-0.33406144677909,-1.21756200064025));
#17460=CARTESIAN_POINT('Ctrl Pts',(28.088858522933,-0.491365261329243,-1.15879939649692));
#17461=CARTESIAN_POINT('Ctrl Pts',(28.0737796659526,-0.723606544051522,
-1.02548045909452));
#17462=CARTESIAN_POINT('Ctrl Pts',(28.0668948495712,-0.816261884977432,
-0.953085469185867));
#17463=CARTESIAN_POINT('Ctrl Pts',(28.0494181450597,-1.02320760685829,-0.73975314249526));
#17464=CARTESIAN_POINT('Ctrl Pts',(28.0403027353165,-1.10952736406557,-0.594731371774655));
#17465=CARTESIAN_POINT('Ctrl Pts',(28.0251273885272,-1.20721997126105,-0.343480859683428));
#17466=CARTESIAN_POINT('Ctrl Pts',(28.0182320724213,-1.23389522300968,-0.228649129135059));
#17467=CARTESIAN_POINT('Ctrl Pts',(28.0007833825742,-1.26074007501739,0.0670551869020103));
#17468=CARTESIAN_POINT('Ctrl Pts',(27.9916773707338,-1.2369704103679,0.233902809861688));
#17469=CARTESIAN_POINT('Ctrl Pts',(27.9765170782386,-1.15523094543665,0.490596117452913));
#17470=CARTESIAN_POINT('Ctrl Pts',(27.9696504679827,-1.10410954293391,0.596333410766813));
#17471=CARTESIAN_POINT('Ctrl Pts',(27.9584962475405,-0.998929190634868,
0.754248903470159));
#17472=CARTESIAN_POINT('Ctrl Pts',(27.9541973498062,-0.952707784063023,
0.812003758880748));
#17473=CARTESIAN_POINT('Ctrl Pts',(27.9446828069813,-0.836372557148644,
0.933237617417355));
#17474=CARTESIAN_POINT('Ctrl Pts',(27.9395147789793,-0.76352459211252,0.99371067926825));
#17475=CARTESIAN_POINT('Ctrl Pts',(27.9276110431682,-0.586654373116962,
1.10958073156092));
#17476=CARTESIAN_POINT('Ctrl Pts',(27.9207162695047,-0.479901383405464,
1.1595048481225));
#17477=CARTESIAN_POINT('Ctrl Pts',(27.9102433336147,-0.309658999011491,
1.2121249866436));
#17478=CARTESIAN_POINT('Ctrl Pts',(27.9066355286707,-0.249344448199697,
1.22602349690604));
#17479=CARTESIAN_POINT('Ctrl Pts',(27.8996144255548,-0.127684267857531,
1.24460926497425));
#17480=CARTESIAN_POINT('Ctrl Pts',(27.8961978838974,-0.0664023934340222,
1.24936472140608));
#17481=CARTESIAN_POINT('Ctrl Pts',(27.8868889978988,0.100755768653574,1.25004530085504));
#17482=CARTESIAN_POINT('Ctrl Pts',(27.8809844783008,0.205835675470576,1.23711210933622));
#17483=CARTESIAN_POINT('Ctrl Pts',(27.866063896433,0.453204407927191,1.1738612253448));
#17484=CARTESIAN_POINT('Ctrl Pts',(27.856213080806,0.608698407592886,1.10681429561789));
#17485=CARTESIAN_POINT('Ctrl Pts',(27.8395800869788,0.846351136838392,0.926418544103274));
#17486=CARTESIAN_POINT('Ctrl Pts',(27.8332688401072,0.927130493094757,0.845659476794221));
#17487=CARTESIAN_POINT('Ctrl Pts',(27.8186212718494,1.07846991579612,0.645463686210442));
#17488=CARTESIAN_POINT('Ctrl Pts',(27.8092257227739,1.15640644586381,0.505721482317762));
#17489=CARTESIAN_POINT('Ctrl Pts',(27.7954118410962,1.22259629351538,0.26771901643447));
#17490=CARTESIAN_POINT('Ctrl Pts',(27.7915580466048,1.23564912429041,0.199007734412521));
#17491=CARTESIAN_POINT('Ctrl Pts',(27.7821086507589,1.25304459091087,0.0322260207484144));
#17492=CARTESIAN_POINT('Ctrl Pts',(27.7763945867012,1.25156055595434,-0.0659228708369851));
#17493=CARTESIAN_POINT('Ctrl Pts',(27.7642947702092,1.22482575759592,-0.269777035042931));
#17494=CARTESIAN_POINT('Ctrl Pts',(27.7579805476016,1.19694742303447,-0.375180422268098));
#17495=CARTESIAN_POINT('Ctrl Pts',(27.7473290248235,1.12462059282187,-0.550801416131723));
#17496=CARTESIAN_POINT('Ctrl Pts',(27.7428588117817,1.08644298546842,-0.622744909367946));
#17497=CARTESIAN_POINT('Ctrl Pts',(27.7330032437985,0.99004410923169,-0.76816749366027));
#17498=CARTESIAN_POINT('Ctrl Pts',(27.7275452739627,0.929840142731238,-0.83980225227136));
#17499=CARTESIAN_POINT('Ctrl Pts',(27.7159670225675,0.787597811969291,-0.975531989088523));
#17500=CARTESIAN_POINT('Ctrl Pts',(27.7098877499555,0.703663058459404,-1.03791885621826));
#17501=CARTESIAN_POINT('Ctrl Pts',(27.6953515319807,0.478261841137807,-1.16472539300529));
#17502=CARTESIAN_POINT('Ctrl Pts',(27.6862138350629,0.319229236952419,-1.22135269437979));
#17503=CARTESIAN_POINT('Ctrl Pts',(27.6729043749472,0.0941610011493839,
-1.24685136243848));
#17504=CARTESIAN_POINT('Ctrl Pts',(27.6701280384454,0.0470868928079041,
-1.24952748149934));
#17505=CARTESIAN_POINT('Ctrl Pts',(27.6673726054814,1.55296021863114E-5,
-1.24955549576934));
#17506=CARTESIAN_POINT('',(27.8084092102543,1.84542703834228E-6,-1.0059988235311));
#17507=CARTESIAN_POINT('',(27.80837346568,-3.363943902264E-14,-1.006));
#17508=CARTESIAN_POINT('Ctrl Pts',(29.3083864422337,0.870773359785393,0.50273974407169));
#17509=CARTESIAN_POINT('Ctrl Pts',(29.3008521885262,0.923830150460179,0.411176385780162));
#17510=CARTESIAN_POINT('Ctrl Pts',(29.2920928354003,0.972239729359923,0.295767848335686));
#17511=CARTESIAN_POINT('Ctrl Pts',(29.2731153143574,1.01254518840658,0.032506499430731));
#17512=CARTESIAN_POINT('Ctrl Pts',(29.2642892222818,1.00848954053166,-0.0936168937764817));
#17513=CARTESIAN_POINT('Ctrl Pts',(29.2460042305897,0.954288507126743,-0.344674989241621));
#17514=CARTESIAN_POINT('Ctrl Pts',(29.2367588244469,0.901467497815239,-0.465863888580671));
#17515=CARTESIAN_POINT('Ctrl Pts',(29.2180479571781,0.750666938273129,-0.68107453632207));
#17516=CARTESIAN_POINT('Ctrl Pts',(29.2088151157514,0.655791268906725,-0.773156797467887));
#17517=CARTESIAN_POINT('Ctrl Pts',(29.1886171121703,0.4183279909562,-0.928000835580233));
#17518=CARTESIAN_POINT('Ctrl Pts',(29.1792516786671,0.290445664438387,-0.968960876829268));
#17519=CARTESIAN_POINT('Ctrl Pts',(29.1624059009713,0.0575864727316603,
-1.01153056273425));
#17520=CARTESIAN_POINT('Ctrl Pts',(29.1534069464231,-0.0710782558689916,
-1.01133291870579));
#17521=CARTESIAN_POINT('Ctrl Pts',(29.1342989682696,-0.33408320271348,-0.95951102980604));
#17522=CARTESIAN_POINT('Ctrl Pts',(29.1247947693779,-0.458249759673372,
-0.903490004899863));
#17523=CARTESIAN_POINT('Ctrl Pts',(29.1082077163494,-0.651606739985276,
-0.773324037322213));
#17524=CARTESIAN_POINT('Ctrl Pts',(29.0990210738255,-0.750738679733316,
-0.686734029266899));
#17525=CARTESIAN_POINT('Ctrl Pts',(29.0788719338336,-0.908027886469017,
-0.45174961613479));
#17526=CARTESIAN_POINT('Ctrl Pts',(29.069460600101,-0.959648553525928,-0.327158651203322));
#17527=CARTESIAN_POINT('Ctrl Pts',(29.0505675506108,-1.01247717924914,-0.0671105513275628));
#17528=CARTESIAN_POINT('Ctrl Pts',(29.0413142276786,-1.01261280867459,0.0652074783840518));
#17529=CARTESIAN_POINT('Ctrl Pts',(29.0226106191189,-0.960786276316734,
0.322740178671338));
#17530=CARTESIAN_POINT('Ctrl Pts',(29.0133914653586,-0.910941399638767,
0.44497502400733));
#17531=CARTESIAN_POINT('Ctrl Pts',(28.9931854475346,-0.755567145070642,
0.682208090561088));
#17532=CARTESIAN_POINT('Ctrl Pts',(28.9838067366341,-0.654636111382683,
0.771092380231502));
#17533=CARTESIAN_POINT('Ctrl Pts',(28.9670009367567,-0.4589204170802,0.903256265996078));
#17534=CARTESIAN_POINT('Ctrl Pts',(28.9580168824801,-0.34122541900454,0.954680725569356));
#17535=CARTESIAN_POINT('Ctrl Pts',(28.9394916971386,-0.0875413822859824,
1.01111645447045));
#17536=CARTESIAN_POINT('Ctrl Pts',(28.9299862507462,0.0486169665867024,
1.01287742140832));
#17537=CARTESIAN_POINT('Ctrl Pts',(28.9128021772271,0.286247499755411,0.969965709350142));
#17538=CARTESIAN_POINT('Ctrl Pts',(28.9036116032874,0.411828409927549,0.930377288092358));
#17539=CARTESIAN_POINT('Ctrl Pts',(28.8834719027533,0.650119117375473,0.778369367719755));
#17540=CARTESIAN_POINT('Ctrl Pts',(28.8740686495798,0.747374114001158,0.685109299358981));
#17541=CARTESIAN_POINT('Ctrl Pts',(28.855169283962,0.900301395997063,0.46815105805523));
#17542=CARTESIAN_POINT('Ctrl Pts',(28.8459048150744,0.953566173341328,0.346849748046555));
#17543=CARTESIAN_POINT('Ctrl Pts',(28.8272137745117,1.00948095071544,0.0903434934989256));
#17544=CARTESIAN_POINT('Ctrl Pts',(28.8180068956468,1.01296598826026,-0.0414324395852837));
#17545=CARTESIAN_POINT('Ctrl Pts',(28.7977899305546,0.96601949268219,-0.321250069431297));
#17546=CARTESIAN_POINT('Ctrl Pts',(28.7883977032764,0.909104926108196,-0.443337235931546));
#17547=CARTESIAN_POINT('Ctrl Pts',(28.7716308252545,0.783304765554663,-0.642559988636238));
#17548=CARTESIAN_POINT('Ctrl Pts',(28.7626606378465,0.696376860255621,-0.736824922057778));
#17549=CARTESIAN_POINT('Ctrl Pts',(28.7441622029206,0.48711729937632,-0.890303235238164));
#17550=CARTESIAN_POINT('Ctrl Pts',(28.7346587869632,0.363230754563944,-0.946762314668834));
#17551=CARTESIAN_POINT('Ctrl Pts',(28.7174342420197,0.127880192190257,-1.00327016540539));
#17552=CARTESIAN_POINT('Ctrl Pts',(28.7082400320689,-0.00307419136589923,
-1.01744177706707));
#17553=CARTESIAN_POINT('Ctrl Pts',(28.6881085385381,-0.28226357624072,-0.974048387998716));
#17554=CARTESIAN_POINT('Ctrl Pts',(28.6787128604578,-0.408717770745895,
-0.927836026440964));
#17555=CARTESIAN_POINT('Ctrl Pts',(28.6598090757102,-0.636054869835315,
-0.790710405276924));
#17556=CARTESIAN_POINT('Ctrl Pts',(28.6505332144177,-0.733676604436167,
-0.700904969244602));
#17557=CARTESIAN_POINT('Ctrl Pts',(28.6318547354579,-0.887904373733202,
-0.488659821461708));
#17558=CARTESIAN_POINT('Ctrl Pts',(28.6226591218941,-0.944048573936195,
-0.369579698988372));
#17559=CARTESIAN_POINT('Ctrl Pts',(28.6024311543348,-1.01369908580114,-0.0943832969988881));
#17560=CARTESIAN_POINT('Ctrl Pts',(28.593026368846,-1.01058265066987,0.0404795504745563));
#17561=CARTESIAN_POINT('Ctrl Pts',(28.5762958650646,-0.975656602098983,
0.272979304096125));
#17562=CARTESIAN_POINT('Ctrl Pts',(28.5673383109915,-0.934104160209119,
0.394084134956389));
#17563=CARTESIAN_POINT('Ctrl Pts',(28.5494086203685,-0.808338952205143,
0.611915865043621));
#17564=CARTESIAN_POINT('Ctrl Pts',(28.5404510663023,-0.724235313104038,
0.708453750739589));
#17565=CARTESIAN_POINT('Ctrl Pts',(28.523720562521,-0.540347644379399,0.854950472866602));
#17566=CARTESIAN_POINT('Ctrl Pts',(28.5143157770323,-0.425111210006109,
0.925080808596303));
#17567=CARTESIAN_POINT('Ctrl Pts',(28.4940878094729,-0.151958878920122,
1.00235989692945));
#17568=CARTESIAN_POINT('Ctrl Pts',(28.4848921959089,-0.0207603676706828,
1.01327765451514));
#17569=CARTESIAN_POINT('Ctrl Pts',(28.466213716949,0.240163206787955,0.985835062226093));
#17570=CARTESIAN_POINT('Ctrl Pts',(28.4569378556565,0.366747863090104,0.946194878116318));
#17571=CARTESIAN_POINT('Ctrl Pts',(28.4380340709089,0.599170684072258,0.817877985664096));
#17572=CARTESIAN_POINT('Ctrl Pts',(28.4286383928286,0.702418860402568,0.731471621586338));
#17573=CARTESIAN_POINT('Ctrl Pts',(28.408506899298,0.879593330129104,0.511383216351959));
#17574=CARTESIAN_POINT('Ctrl Pts',(28.3993126893472,0.932797546195434,0.390887587624588));
#17575=CARTESIAN_POINT('Ctrl Pts',(28.3820881444036,1.00153559313095,0.158814096445713));
#17576=CARTESIAN_POINT('Ctrl Pts',(28.3725847284462,1.01458386847578,0.0232956617357079));
#17577=CARTESIAN_POINT('Ctrl Pts',(28.3540862935203,0.986297530771062,-0.234667590561133));
#17578=CARTESIAN_POINT('Ctrl Pts',(28.3451161061124,0.94812565639132,-0.357081831558977));
#17579=CARTESIAN_POINT('Ctrl Pts',(28.3283492280907,0.838493771813711,-0.565639342750808));
#17580=CARTESIAN_POINT('Ctrl Pts',(28.3189570008126,0.761220467435563,-0.675972386498997));
#17581=CARTESIAN_POINT('Ctrl Pts',(28.2987400357204,0.542364539351688,-0.856538059210497));
#17582=CARTESIAN_POINT('Ctrl Pts',(28.2895331568556,0.426500714921247,-0.919407894705333));
#17583=CARTESIAN_POINT('Ctrl Pts',(28.2708421162929,0.17640239356655,-0.999237404326076));
#17584=CARTESIAN_POINT('Ctrl Pts',(28.2615776474052,0.0447199889143341,
-1.01375940902338));
#17585=CARTESIAN_POINT('Ctrl Pts',(28.2426782817872,-0.219635000613443,
-0.989799618535093));
#17586=CARTESIAN_POINT('Ctrl Pts',(28.2332750286137,-0.349028087285606,
-0.952204354992624));
#17587=CARTESIAN_POINT('Ctrl Pts',(28.2131353280796,-0.599816161628714,
-0.821842509043127));
#17588=CARTESIAN_POINT('Ctrl Pts',(28.2039447541399,-0.696891195219628,
-0.73288046123261));
#17589=CARTESIAN_POINT('Ctrl Pts',(28.1867606806209,-0.852869094566055,
-0.548542238822853));
#17590=CARTESIAN_POINT('Ctrl Pts',(28.1772552342284,-0.919423226898889,
-0.429745166292887));
#17591=CARTESIAN_POINT('Ctrl Pts',(28.158730048887,-0.997390470348596,-0.181830481509589));
#17592=CARTESIAN_POINT('Ctrl Pts',(28.1497459946104,-1.01170308102003,-0.0541913934911194));
#17593=CARTESIAN_POINT('Ctrl Pts',(28.132940194733,-0.995103645636232,0.181385312576464));
#17594=CARTESIAN_POINT('Ctrl Pts',(28.1235614838324,-0.968593109628244,
0.313236296615785));
#17595=CARTESIAN_POINT('Ctrl Pts',(28.1033554660083,-0.840830374658895,
0.566410881442946));
#17596=CARTESIAN_POINT('Ctrl Pts',(28.094136312248,-0.759894331709154,0.670695233562644));
#17597=CARTESIAN_POINT('Ctrl Pts',(28.0754327036883,-0.562777737133924,
0.844344677318257));
#17598=CARTESIAN_POINT('Ctrl Pts',(28.066179380756,-0.448119147312189,0.910386233646077));
#17599=CARTESIAN_POINT('Ctrl Pts',(28.0472863312657,-0.196496573752323,
0.994659351660517));
#17600=CARTESIAN_POINT('Ctrl Pts',(28.037874997533,-0.0627872995112181,
1.01225002509461));
#17601=CARTESIAN_POINT('Ctrl Pts',(28.017725857541,0.219359775122049,0.993525782886262));
#17602=CARTESIAN_POINT('Ctrl Pts',(28.0085392150173,0.343914891685593,0.950970008765679));
#17603=CARTESIAN_POINT('Ctrl Pts',(27.9919521619889,0.553320416471902,0.848600935605234));
#17604=CARTESIAN_POINT('Ctrl Pts',(27.9824479630972,0.663919325666461,0.769080055430507));
#17605=CARTESIAN_POINT('Ctrl Pts',(27.9633399849438,0.840300871347782,0.56722203459224));
#17606=CARTESIAN_POINT('Ctrl Pts',(27.9543410303957,0.904804400397691,0.455893933067184));
#17607=CARTESIAN_POINT('Ctrl Pts',(27.9374952527,0.984367566826246,0.23294711459173));
#17608=CARTESIAN_POINT('Ctrl Pts',(27.9281298191968,1.01283629382342,0.101717750507591));
#17609=CARTESIAN_POINT('Ctrl Pts',(27.9079318156157,0.997469062168756,-0.181353499719985));
#17610=CARTESIAN_POINT('Ctrl Pts',(27.8986989741889,0.965161319461705,-0.309559370165414));
#17611=CARTESIAN_POINT('Ctrl Pts',(27.8799881069201,0.85418371112365,-0.547761809504526));
#17612=CARTESIAN_POINT('Ctrl Pts',(27.8707427007773,0.775641550295086,-0.654100595091252));
#17613=CARTESIAN_POINT('Ctrl Pts',(27.8524577057846,0.5853193441443,-0.826569145795593));
#17614=CARTESIAN_POINT('Ctrl Pts',(27.8436316104026,0.478121059661468,-0.893143155202069));
#17615=CARTESIAN_POINT('Ctrl Pts',(27.8246541289103,0.229977818093696,-0.989868041870531));
#17616=CARTESIAN_POINT('Ctrl Pts',(27.8158948070511,0.105826781086848,-1.0056484510065));
#17617=CARTESIAN_POINT('Ctrl Pts',(27.8083605733564,2.47301423003647E-6,
-1.00548172441298));
#17618=CARTESIAN_POINT('Ctrl Pts',(29.66948943148,0.7571184320868,1.04208412158));
#17619=CARTESIAN_POINT('Ctrl Pts',(29.65323943148,0.9935598191429,0.8702993985028));
#17620=CARTESIAN_POINT('Ctrl Pts',(29.62073943148,1.34389945081,0.360234290888));
#17621=CARTESIAN_POINT('Ctrl Pts',(29.57198943148,1.271190105891,-0.5659807228689));
#17622=CARTESIAN_POINT('Ctrl Pts',(29.52323943148,0.6316952655301,-1.239784036163));
#17623=CARTESIAN_POINT('Ctrl Pts',(29.47448943148,-0.2892961135977,-1.361045654676));
#17624=CARTESIAN_POINT('Ctrl Pts',(29.42573943148,-1.081360653838,-0.8756674965057));
#17625=CARTESIAN_POINT('Ctrl Pts',(29.37698943148,-1.391450057306,-1.387658549734E-7));
#17626=CARTESIAN_POINT('Ctrl Pts',(29.32823943148,-1.081359992212,0.8756680515693));
#17627=CARTESIAN_POINT('Ctrl Pts',(29.27948943148,-0.2892987601002,1.361043711953));
#17628=CARTESIAN_POINT('Ctrl Pts',(29.23073943148,0.6317051899145,1.239791251989));
#17629=CARTESIAN_POINT('Ctrl Pts',(29.18198943148,1.271153054855,0.5659538022855));
#17630=CARTESIAN_POINT('Ctrl Pts',(29.13323943148,1.344037730566,-0.3601338243813));
#17631=CARTESIAN_POINT('Ctrl Pts',(29.08448943148,0.8178739353206,-1.125706897754));
#17632=CARTESIAN_POINT('Ctrl Pts',(29.03573943148,-0.07282287932829,-1.389543314081));
#17633=CARTESIAN_POINT('Ctrl Pts',(28.98698943148,-0.9310619483587,-1.034049051938));
#17634=CARTESIAN_POINT('Ctrl Pts',(28.93823943148,-1.374319186766,-0.217670775222));
#17635=CARTESIAN_POINT('Ctrl Pts',(28.88948943148,-1.20503126313,0.69572512415));
#17636=CARTESIAN_POINT('Ctrl Pts',(28.84073943148,-0.4986511723795,1.299030716259));
#17637=CARTESIAN_POINT('Ctrl Pts',(28.79198943148,0.429981773558,1.323347825744));
#17638=CARTESIAN_POINT('Ctrl Pts',(28.74323943148,1.166968369989,0.7578381205155));
#17639=CARTESIAN_POINT('Ctrl Pts',(28.69448943148,1.383827738331,-0.1454461562039));
#17640=CARTESIAN_POINT('Ctrl Pts',(28.64573943148,0.9839039059593,-0.9839039061246));
#17641=CARTESIAN_POINT('Ctrl Pts',(28.59698943148,0.14544615728,-1.383827738746));
#17642=CARTESIAN_POINT('Ctrl Pts',(28.54823943148,-0.7578381246551,-1.166968368163));
#17643=CARTESIAN_POINT('Ctrl Pts',(28.49948943148,-1.323347810262,-0.4299817804463));
#17644=CARTESIAN_POINT('Ctrl Pts',(28.45073943148,-1.299030774048,0.4986511981073));
#17645=CARTESIAN_POINT('Ctrl Pts',(28.40198943148,-0.6957249084782,1.205031167107));
#17646=CARTESIAN_POINT('Ctrl Pts',(28.35323943148,0.2176699703234,1.374319545129));
#17647=CARTESIAN_POINT('Ctrl Pts',(28.30448943148,1.034052055861,0.9310606109294));
#17648=CARTESIAN_POINT('Ctrl Pts',(28.25573943148,1.389532103288,0.0728278706819));
#17649=CARTESIAN_POINT('Ctrl Pts',(28.20698943148,1.125748737002,-0.8178925633062));
#17650=CARTESIAN_POINT('Ctrl Pts',(28.15823943148,0.3599776781819,-1.343968209978));
#17651=CARTESIAN_POINT('Ctrl Pts',(28.12573943148,-0.2569214784304,-1.295597742809));
#17652=CARTESIAN_POINT('Ctrl Pts',(28.10948943148,-0.5239121061251,-1.17672585665));
#17653=CARTESIAN_POINT('Ctrl Pts',(29.6078719886,0.6943873204196,0.9557421536299));
#17654=CARTESIAN_POINT('Ctrl Pts',(29.5916219886,0.9112383363718,0.7981906682994));
#17655=CARTESIAN_POINT('Ctrl Pts',(29.5591219886,1.232550548254,0.3303870482766));
#17656=CARTESIAN_POINT('Ctrl Pts',(29.5103719886,1.165865542251,-0.5190863422501));
#17657=CARTESIAN_POINT('Ctrl Pts',(29.4616219886,0.5793561009262,-1.137061625084));
#17658=CARTESIAN_POINT('Ctrl Pts',(29.4128719886,-0.26532645966,-1.248276101949));
#17659=CARTESIAN_POINT('Ctrl Pts',(29.3641219886,-0.9917644254889,-0.8031139920886));
#17660=CARTESIAN_POINT('Ctrl Pts',(29.3153719886,-1.27616134523,-1.272683984522E-7));
#17661=CARTESIAN_POINT('Ctrl Pts',(29.2666219886,-0.9917638186823,0.8031145011624));
#17662=CARTESIAN_POINT('Ctrl Pts',(29.2178719886,-0.2653288868863,1.248274320191));
#17663=CARTESIAN_POINT('Ctrl Pts',(29.1691219886,0.5793652030249,1.137068243043));
#17664=CARTESIAN_POINT('Ctrl Pts',(29.1203719886,1.165831561083,0.5190616521739));
#17665=CARTESIAN_POINT('Ctrl Pts',(29.0716219886,1.232677370829,-0.3302949059308));
#17666=CARTESIAN_POINT('Ctrl Pts',(29.0228719886,0.7501089212991,-1.032436357618));
#17667=CARTESIAN_POINT('Ctrl Pts',(28.9741219886,-0.066789133508,-1.274412585376));
#17668=CARTESIAN_POINT('Ctrl Pts',(28.9253719886,-0.8539187319524,-0.948372830362));
#17669=CARTESIAN_POINT('Ctrl Pts',(28.8766219886,-1.260449854417,-0.1996356447477));
#17670=CARTESIAN_POINT('Ctrl Pts',(28.8278719886,-1.105188295998,0.6380807601996));
#17671=CARTESIAN_POINT('Ctrl Pts',(28.7791219886,-0.4573353873558,1.191399416495));
#17672=CARTESIAN_POINT('Ctrl Pts',(28.7303719886,0.3943555973763,1.213701729819));
#17673=CARTESIAN_POINT('Ctrl Pts',(28.6816219886,1.070279107084,0.6950473790027));
#17674=CARTESIAN_POINT('Ctrl Pts',(28.6328719886,1.269170574137,-0.1333952026414));
#17675=CARTESIAN_POINT('Ctrl Pts',(28.5841219886,0.9023824646909,-0.9023824648426));
#17676=CARTESIAN_POINT('Ctrl Pts',(28.5353719886,0.1333952036283,-1.269170574518));
#17677=CARTESIAN_POINT('Ctrl Pts',(28.4866219886,-0.6950473827993,-1.07027910541));
#17678=CARTESIAN_POINT('Ctrl Pts',(28.4378719886,-1.21370171562,-0.3943556036939));
#17679=CARTESIAN_POINT('Ctrl Pts',(28.3891219886,-1.191399469495,0.457335410952));
#17680=CARTESIAN_POINT('Ctrl Pts',(28.3403719886,-0.6380805623973,1.105188207931));
#17681=CARTESIAN_POINT('Ctrl Pts',(28.2916219886,0.1996349065391,1.260450183087));
#17682=CARTESIAN_POINT('Ctrl Pts',(28.2428719886,0.9483755853946,0.853917505336));
#17683=CARTESIAN_POINT('Ctrl Pts',(28.1941219886,1.274402303455,0.06679371130257));
#17684=CARTESIAN_POINT('Ctrl Pts',(28.1453719886,1.032474730272,-0.7501260058614));
#17685=CARTESIAN_POINT('Ctrl Pts',(28.0966219886,0.3301516972379,-1.232613610374));
#17686=CARTESIAN_POINT('Ctrl Pts',(28.0641219886,-0.2356342276251,-1.18825088235));
#17687=CARTESIAN_POINT('Ctrl Pts',(28.0478719886,-0.4805033243014,-1.079228136364));
#17688=CARTESIAN_POINT('Ctrl Pts',(29.54625454572,0.6316562087523,0.86940018568));
#17689=CARTESIAN_POINT('Ctrl Pts',(29.53000454572,0.8289168536007,0.7260819380959));
#17690=CARTESIAN_POINT('Ctrl Pts',(29.49750454572,1.121201645697,0.3005398056651));
#17691=CARTESIAN_POINT('Ctrl Pts',(29.44875454572,1.060540978612,-0.4721919616313));
#17692=CARTESIAN_POINT('Ctrl Pts',(29.40000454572,0.5270169363223,-1.034339214006));
#17693=CARTESIAN_POINT('Ctrl Pts',(29.35125454572,-0.2413568057223,-1.135506549222));
#17694=CARTESIAN_POINT('Ctrl Pts',(29.30250454572,-0.9021681971399,-0.7305604876715));
#17695=CARTESIAN_POINT('Ctrl Pts',(29.25375454572,-1.160872633154,-1.157709407763E-7));
#17696=CARTESIAN_POINT('Ctrl Pts',(29.20500454572,-0.9021676451524,0.7305609507555));
#17697=CARTESIAN_POINT('Ctrl Pts',(29.15625454572,-0.2413590136723,1.135504928428));
#17698=CARTESIAN_POINT('Ctrl Pts',(29.10750454572,0.5270252161353,1.034345234097));
#17699=CARTESIAN_POINT('Ctrl Pts',(29.05875454572,1.06051006731,0.4721695020623));
#17700=CARTESIAN_POINT('Ctrl Pts',(29.01000454572,1.121317011091,-0.3004559874803));
#17701=CARTESIAN_POINT('Ctrl Pts',(28.96125454572,0.6823439072775,-0.9391658174822));
#17702=CARTESIAN_POINT('Ctrl Pts',(28.91250454572,-0.0607553876877,-1.159281856671));
#17703=CARTESIAN_POINT('Ctrl Pts',(28.86375454572,-0.7767755155462,-0.8626966087863));
#17704=CARTESIAN_POINT('Ctrl Pts',(28.81500454572,-1.146580522067,-0.1816005142735));
#17705=CARTESIAN_POINT('Ctrl Pts',(28.76625454572,-1.005345328866,0.5804363962492));
#17706=CARTESIAN_POINT('Ctrl Pts',(28.71750454572,-0.4160196023322,1.083768116731));
#17707=CARTESIAN_POINT('Ctrl Pts',(28.66875454572,0.3587294211946,1.104055633894));
#17708=CARTESIAN_POINT('Ctrl Pts',(28.62000454572,0.9735898441798,0.6322566374899));
#17709=CARTESIAN_POINT('Ctrl Pts',(28.57125454572,1.154513409944,-0.1213442490789));
#17710=CARTESIAN_POINT('Ctrl Pts',(28.52250454572,0.8208610234226,-0.8208610235605));
#17711=CARTESIAN_POINT('Ctrl Pts',(28.47375454572,0.1213442499766,-1.154513410291));
#17712=CARTESIAN_POINT('Ctrl Pts',(28.42500454572,-0.6322566409435,-0.9735898426565));
#17713=CARTESIAN_POINT('Ctrl Pts',(28.37625454572,-1.104055620977,-0.3587294269414));
#17714=CARTESIAN_POINT('Ctrl Pts',(28.32750454572,-1.083768164943,0.4160196237967));
#17715=CARTESIAN_POINT('Ctrl Pts',(28.27875454572,-0.5804362163164,1.005345248755));
#17716=CARTESIAN_POINT('Ctrl Pts',(28.23000454572,0.1815998427548,1.146580821045));
#17717=CARTESIAN_POINT('Ctrl Pts',(28.18125454572,0.8626991149286,0.7767743997426));
#17718=CARTESIAN_POINT('Ctrl Pts',(28.13250454572,1.159272503621,0.06075955192325));
#17719=CARTESIAN_POINT('Ctrl Pts',(28.08375454572,0.9392007235413,-0.6823594484165));
#17720=CARTESIAN_POINT('Ctrl Pts',(28.03500454572,0.300325716294,-1.121259010771));
#17721=CARTESIAN_POINT('Ctrl Pts',(28.00250454572,-0.2143469768198,-1.080904021891));
#17722=CARTESIAN_POINT('Ctrl Pts',(27.98625454572,-0.4370945424777,-0.9817304160776));
#17723=CARTESIAN_POINT('Ctrl Pts',(29.48463710284,0.5689250970851,0.7830582177302));
#17724=CARTESIAN_POINT('Ctrl Pts',(29.46838710284,0.7465953708295,0.6539732078924));
#17725=CARTESIAN_POINT('Ctrl Pts',(29.43588710284,1.00985274314,0.2706925630537));
#17726=CARTESIAN_POINT('Ctrl Pts',(29.38713710284,0.9552164149722,-0.4252975810125));
#17727=CARTESIAN_POINT('Ctrl Pts',(29.33838710284,0.4746777717184,-0.9316168029278));
#17728=CARTESIAN_POINT('Ctrl Pts',(29.28963710284,-0.2173871517845,-1.022736996495));
#17729=CARTESIAN_POINT('Ctrl Pts',(29.24088710284,-0.812571968791,-0.6580069832544));
#17730=CARTESIAN_POINT('Ctrl Pts',(29.19213710284,-1.045583921078,-1.042734842915E-7));
#17731=CARTESIAN_POINT('Ctrl Pts',(29.14338710284,-0.8125714716224,0.6580074003485));
#17732=CARTESIAN_POINT('Ctrl Pts',(29.09463710284,-0.2173891404584,1.022735536666));
#17733=CARTESIAN_POINT('Ctrl Pts',(29.04588710284,0.4746852292457,0.9316222251505));
#17734=CARTESIAN_POINT('Ctrl Pts',(28.99713710284,0.9551885735371,0.4252773519507));
#17735=CARTESIAN_POINT('Ctrl Pts',(28.94838710284,1.009956651354,-0.2706170690297));
#17736=CARTESIAN_POINT('Ctrl Pts',(28.89963710284,0.614578893256,-0.8458952773463));
#17737=CARTESIAN_POINT('Ctrl Pts',(28.85088710284,-0.0547216418674,-1.044151127966));
#17738=CARTESIAN_POINT('Ctrl Pts',(28.80213710284,-0.69963229914,-0.7770203872106));
#17739=CARTESIAN_POINT('Ctrl Pts',(28.75338710284,-1.032711189717,-0.1635653837992));
#17740=CARTESIAN_POINT('Ctrl Pts',(28.70463710284,-0.9055023617337,0.5227920322988));
#17741=CARTESIAN_POINT('Ctrl Pts',(28.65588710284,-0.3747038173085,0.9761368169669));
#17742=CARTESIAN_POINT('Ctrl Pts',(28.60713710284,0.3231032450129,0.9944095379687));
#17743=CARTESIAN_POINT('Ctrl Pts',(28.55838710284,0.8769005812753,0.569465895977));
#17744=CARTESIAN_POINT('Ctrl Pts',(28.50963710284,1.039856245751,-0.1092932955163));
#17745=CARTESIAN_POINT('Ctrl Pts',(28.46088710284,0.7393395821542,-0.7393395822784));
#17746=CARTESIAN_POINT('Ctrl Pts',(28.41213710284,0.109293296325,-1.039856246063));
#17747=CARTESIAN_POINT('Ctrl Pts',(28.36338710284,-0.5694658990877,-0.8769005799032));
#17748=CARTESIAN_POINT('Ctrl Pts',(28.31463710284,-0.994409526335,-0.323103250189));
#17749=CARTESIAN_POINT('Ctrl Pts',(28.26588710284,-0.9761368603912,0.3747038366413));
#17750=CARTESIAN_POINT('Ctrl Pts',(28.21713710284,-0.5227918702355,0.905502289579));
#17751=CARTESIAN_POINT('Ctrl Pts',(28.16838710284,0.1635647789705,1.032711459003));
#17752=CARTESIAN_POINT('Ctrl Pts',(28.11963710284,0.7770226444627,0.6996312941492));
#17753=CARTESIAN_POINT('Ctrl Pts',(28.07088710284,1.044142703787,0.05472539254393));
#17754=CARTESIAN_POINT('Ctrl Pts',(28.02213710284,0.845926716811,-0.6145928909717));
#17755=CARTESIAN_POINT('Ctrl Pts',(27.97338710284,0.27049973535,-1.009904411168));
#17756=CARTESIAN_POINT('Ctrl Pts',(27.94088710284,-0.1930597260145,-0.9735571614325));
#17757=CARTESIAN_POINT('Ctrl Pts',(27.92463710284,-0.393685760654,-0.8842326957913));
#17758=CARTESIAN_POINT('',(27.9766265322859,2.05983980323309E-10,-1.00599991871459));
#17759=CARTESIAN_POINT('Ctrl Pts',(29.4766395048596,0.870773402089107,0.502739671065568));
#17760=CARTESIAN_POINT('Ctrl Pts',(29.4691052524585,0.923830175985616,0.411176324318506));
#17761=CARTESIAN_POINT('Ctrl Pts',(29.4603459013364,0.972239735087807,0.295767810922782));
#17762=CARTESIAN_POINT('Ctrl Pts',(29.4413683829903,1.01254518840659,0.0325064994309846));
#17763=CARTESIAN_POINT('Ctrl Pts',(29.4325422909147,1.00848954053169,-0.0936168937763489));
#17764=CARTESIAN_POINT('Ctrl Pts',(29.4142572992227,0.954288507126751,-0.344674989241598));
#17765=CARTESIAN_POINT('Ctrl Pts',(29.4050118930799,0.901467497815252,-0.465863888580647));
#17766=CARTESIAN_POINT('Ctrl Pts',(29.3863010258111,0.750666938273149,-0.681074536322047));
#17767=CARTESIAN_POINT('Ctrl Pts',(29.3770681843844,0.655791268906749,-0.773156797467866));
#17768=CARTESIAN_POINT('Ctrl Pts',(29.3568701808035,0.418327990956232,-0.928000835580218));
#17769=CARTESIAN_POINT('Ctrl Pts',(29.3475047473003,0.290445664438423,-0.968960876829257));
#17770=CARTESIAN_POINT('Ctrl Pts',(29.3306589696046,0.0575864727316964,
-1.01153056273425));
#17771=CARTESIAN_POINT('Ctrl Pts',(29.3216600150564,-0.0710782558689575,
-1.01133291870579));
#17772=CARTESIAN_POINT('Ctrl Pts',(29.3025520369029,-0.33408320271347,-0.959511029806047));
#17773=CARTESIAN_POINT('Ctrl Pts',(29.2930478380111,-0.458249759673364,
-0.903490004899866));
#17774=CARTESIAN_POINT('Ctrl Pts',(29.2764607849825,-0.651606739985256,
-0.773324037322229));
#17775=CARTESIAN_POINT('Ctrl Pts',(29.2672741424586,-0.750738679733299,
-0.686734029266918));
#17776=CARTESIAN_POINT('Ctrl Pts',(29.2471250024667,-0.908027886469006,
-0.451749616134813));
#17777=CARTESIAN_POINT('Ctrl Pts',(29.237713668734,-0.95964855352592,-0.327158651203346));
#17778=CARTESIAN_POINT('Ctrl Pts',(29.2188206192439,-1.01247717924914,-0.0671105513275875));
#17779=CARTESIAN_POINT('Ctrl Pts',(29.2095672963116,-1.01261280867459,0.0652074783840267));
#17780=CARTESIAN_POINT('Ctrl Pts',(29.190863687752,-0.960786276316742,0.322740178671316));
#17781=CARTESIAN_POINT('Ctrl Pts',(29.1816445339917,-0.910941399638776,
0.444975024007311));
#17782=CARTESIAN_POINT('Ctrl Pts',(29.1614385161677,-0.755567145070654,
0.682208090561074));
#17783=CARTESIAN_POINT('Ctrl Pts',(29.1520598052671,-0.654636111382696,
0.771092380231491));
#17784=CARTESIAN_POINT('Ctrl Pts',(29.1352540053897,-0.458920417080214,
0.903256265996071));
#17785=CARTESIAN_POINT('Ctrl Pts',(29.126269951113,-0.341225419004554,0.954680725569352));
#17786=CARTESIAN_POINT('Ctrl Pts',(29.1077447657715,-0.0875413822859973,
1.01111645447045));
#17787=CARTESIAN_POINT('Ctrl Pts',(29.0982393193791,0.0486169665866859,
1.01287742140832));
#17788=CARTESIAN_POINT('Ctrl Pts',(29.08105524586,0.286247499755392,0.969965709350147));
#17789=CARTESIAN_POINT('Ctrl Pts',(29.0718646719204,0.411828409927529,0.930377288092367));
#17790=CARTESIAN_POINT('Ctrl Pts',(29.0517249713864,0.650119117375458,0.778369367719768));
#17791=CARTESIAN_POINT('Ctrl Pts',(29.0423217182129,0.747374114001147,0.685109299358994));
#17792=CARTESIAN_POINT('Ctrl Pts',(29.023422352595,0.900301395997063,0.468151058055233));
#17793=CARTESIAN_POINT('Ctrl Pts',(29.0141578837073,0.95356617334133,0.346849748046551));
#17794=CARTESIAN_POINT('Ctrl Pts',(28.9954668431443,1.00948095071544,0.0903434934989169));
#17795=CARTESIAN_POINT('Ctrl Pts',(28.9862599642793,1.01296598826026,-0.0414324395852936));
#17796=CARTESIAN_POINT('Ctrl Pts',(28.966042999187,0.966019492682187,-0.321250069431303));
#17797=CARTESIAN_POINT('Ctrl Pts',(28.956650771909,0.909104926108195,-0.443337235931549));
#17798=CARTESIAN_POINT('Ctrl Pts',(28.9398838938874,0.783304765554662,-0.642559988636239));
#17799=CARTESIAN_POINT('Ctrl Pts',(28.9309137064795,0.696376860255623,-0.736824922057775));
#17800=CARTESIAN_POINT('Ctrl Pts',(28.9124152715538,0.487117299376328,-0.890303235238159));
#17801=CARTESIAN_POINT('Ctrl Pts',(28.9029118555964,0.363230754563954,-0.94676231466883));
#17802=CARTESIAN_POINT('Ctrl Pts',(28.8856873106528,0.127880192190271,-1.00327016540539));
#17803=CARTESIAN_POINT('Ctrl Pts',(28.876493100702,-0.00307419136588492,
-1.01744177706707));
#17804=CARTESIAN_POINT('Ctrl Pts',(28.8563616071713,-0.282263576240707,
-0.97404838799872));
#17805=CARTESIAN_POINT('Ctrl Pts',(28.846965929091,-0.408717770745884,-0.927836026440969));
#17806=CARTESIAN_POINT('Ctrl Pts',(28.8280621443433,-0.636054869835307,
-0.79071040527693));
#17807=CARTESIAN_POINT('Ctrl Pts',(28.8187862830508,-0.733676604436161,
-0.700904969244608));
#17808=CARTESIAN_POINT('Ctrl Pts',(28.800107804091,-0.887904373733199,-0.488659821461714));
#17809=CARTESIAN_POINT('Ctrl Pts',(28.7909121905271,-0.944048573936193,
-0.369579698988377));
#17810=CARTESIAN_POINT('Ctrl Pts',(28.7706842229678,-1.01369908580114,-0.0943832969988919));
#17811=CARTESIAN_POINT('Ctrl Pts',(28.761279437479,-1.01058265066987,0.0404795504745535));
#17812=CARTESIAN_POINT('Ctrl Pts',(28.7445489336977,-0.975656602098983,
0.272979304096127));
#17813=CARTESIAN_POINT('Ctrl Pts',(28.7355913796315,-0.934104160209119,
0.394084134956389));
#17814=CARTESIAN_POINT('Ctrl Pts',(28.7176616890085,-0.808338952205141,
0.611915865043623));
#17815=CARTESIAN_POINT('Ctrl Pts',(28.7087041349353,-0.724235313104034,
0.708453750739594));
#17816=CARTESIAN_POINT('Ctrl Pts',(28.6919736311539,-0.540347644379399,
0.854950472866602));
#17817=CARTESIAN_POINT('Ctrl Pts',(28.6825688456651,-0.425111210006108,
0.925080808596303));
#17818=CARTESIAN_POINT('Ctrl Pts',(28.6623408781058,-0.151958878920123,
1.00235989692945));
#17819=CARTESIAN_POINT('Ctrl Pts',(28.653145264542,-0.0207603676706871,
1.01327765451514));
#17820=CARTESIAN_POINT('Ctrl Pts',(28.6344667855823,0.240163206787947,0.985835062226095));
#17821=CARTESIAN_POINT('Ctrl Pts',(28.6251909242898,0.366747863090091,0.946194878116322));
#17822=CARTESIAN_POINT('Ctrl Pts',(28.6062871395422,0.599170684072242,0.817877985664108));
#17823=CARTESIAN_POINT('Ctrl Pts',(28.5968914614618,0.702418860402553,0.731471621586352));
#17824=CARTESIAN_POINT('Ctrl Pts',(28.5767599679311,0.879593330129096,0.511383216351974));
#17825=CARTESIAN_POINT('Ctrl Pts',(28.5675657579803,0.93279754619543,0.3908875876246));
#17826=CARTESIAN_POINT('Ctrl Pts',(28.5503412130367,1.00153559313095,0.158814096445722));
#17827=CARTESIAN_POINT('Ctrl Pts',(28.5408377970793,1.01458386847578,0.023295661735716));
#17828=CARTESIAN_POINT('Ctrl Pts',(28.5223393621534,0.986297530771063,-0.234667590561126));
#17829=CARTESIAN_POINT('Ctrl Pts',(28.5133691747455,0.948125656391323,-0.35708183155897));
#17830=CARTESIAN_POINT('Ctrl Pts',(28.4966022967238,0.838493771813713,-0.565639342750806));
#17831=CARTESIAN_POINT('Ctrl Pts',(28.4872100694457,0.761220467435563,-0.675972386498998));
#17832=CARTESIAN_POINT('Ctrl Pts',(28.4669931043534,0.542364539351682,-0.856538059210502));
#17833=CARTESIAN_POINT('Ctrl Pts',(28.4577862254884,0.426500714921235,-0.919407894705339));
#17834=CARTESIAN_POINT('Ctrl Pts',(28.4390951849256,0.176402393566531,-0.99923740432608));
#17835=CARTESIAN_POINT('Ctrl Pts',(28.4298307160378,0.0447199889143125,
-1.01375940902338));
#17836=CARTESIAN_POINT('Ctrl Pts',(28.41093135042,-0.219635000613468,-0.989799618535087));
#17837=CARTESIAN_POINT('Ctrl Pts',(28.4015280972466,-0.349028087285628,
-0.952204354992616));
#17838=CARTESIAN_POINT('Ctrl Pts',(28.3813883967126,-0.599816161628727,
-0.821842509043117));
#17839=CARTESIAN_POINT('Ctrl Pts',(28.3721978227729,-0.696891195219636,
-0.732880461232601));
#17840=CARTESIAN_POINT('Ctrl Pts',(28.3550137492539,-0.85286909456606,-0.548542238822846));
#17841=CARTESIAN_POINT('Ctrl Pts',(28.3455083028614,-0.919423226898893,
-0.429745166292879));
#17842=CARTESIAN_POINT('Ctrl Pts',(28.3269831175199,-0.997390470348598,
-0.181830481509578));
#17843=CARTESIAN_POINT('Ctrl Pts',(28.3179990632432,-1.01170308102003,-0.0541913934911062));
#17844=CARTESIAN_POINT('Ctrl Pts',(28.3011932633659,-0.995103645636229,
0.181385312576479));
#17845=CARTESIAN_POINT('Ctrl Pts',(28.2918145524652,-0.968593109628239,
0.313236296615798));
#17846=CARTESIAN_POINT('Ctrl Pts',(28.2716085346412,-0.840830374658889,
0.566410881442955));
#17847=CARTESIAN_POINT('Ctrl Pts',(28.262389380881,-0.759894331709147,0.670695233562651));
#17848=CARTESIAN_POINT('Ctrl Pts',(28.2436857723214,-0.562777737133921,
0.844344677318258));
#17849=CARTESIAN_POINT('Ctrl Pts',(28.2344324493892,-0.448119147312191,
0.910386233646076));
#17850=CARTESIAN_POINT('Ctrl Pts',(28.2155393998992,-0.196496573752333,
0.994659351660514));
#17851=CARTESIAN_POINT('Ctrl Pts',(28.2061280661666,-0.0627872995112383,
1.01225002509461));
#17852=CARTESIAN_POINT('Ctrl Pts',(28.1859789261748,0.21935977512202,0.993525782886269));
#17853=CARTESIAN_POINT('Ctrl Pts',(28.1767922836509,0.343914891685563,0.95097000876569));
#17854=CARTESIAN_POINT('Ctrl Pts',(28.1602052306222,0.553320416471885,0.848600935605246));
#17855=CARTESIAN_POINT('Ctrl Pts',(28.1507010317303,0.663919325666453,0.769080055430514));
#17856=CARTESIAN_POINT('Ctrl Pts',(28.1315930535768,0.840300871347782,0.567222034592242));
#17857=CARTESIAN_POINT('Ctrl Pts',(28.1225940990285,0.904804400397695,0.455893933067178));
#17858=CARTESIAN_POINT('Ctrl Pts',(28.1057483213327,0.98436756682625,0.232947114591715));
#17859=CARTESIAN_POINT('Ctrl Pts',(28.0963828878294,1.01283629382343,0.101717750507575));
#17860=CARTESIAN_POINT('Ctrl Pts',(28.0761848842484,0.997469062168753,-0.181353499720004));
#17861=CARTESIAN_POINT('Ctrl Pts',(28.0669520428217,0.965161319461699,-0.309559370165432));
#17862=CARTESIAN_POINT('Ctrl Pts',(28.048241175553,0.854183711123641,-0.54776180950454));
#17863=CARTESIAN_POINT('Ctrl Pts',(28.0389957694103,0.775641550295079,-0.65410059509126));
#17864=CARTESIAN_POINT('Ctrl Pts',(28.0207108054875,0.585319667539776,-0.826568852737046));
#17865=CARTESIAN_POINT('Ctrl Pts',(28.0118847412308,0.4781218150517,-0.893142685975639));
#17866=CARTESIAN_POINT('Ctrl Pts',(27.9929072063119,0.229977999238873,-0.989868172118325));
#17867=CARTESIAN_POINT('Ctrl Pts',(27.9841478270495,0.105826098472935,-1.00564856987941));
#17868=CARTESIAN_POINT('Ctrl Pts',(27.9766135594424,1.31358039184295E-6,
-1.00548172258563));
#17869=CARTESIAN_POINT('',(28.1175,-3.956254470204E-14,-1.25));
#17870=CARTESIAN_POINT('Ctrl Pts',(28.16948943148,0.523912106125,-1.17672585665));
#17871=CARTESIAN_POINT('Ctrl Pts',(28.15323943148,0.2569214784303,-1.295597742809));
#17872=CARTESIAN_POINT('Ctrl Pts',(28.12073943148,-0.359977678182,-1.343968209978));
#17873=CARTESIAN_POINT('Ctrl Pts',(28.07198943148,-1.125748737002,-0.8178925633062));
#17874=CARTESIAN_POINT('Ctrl Pts',(28.02323943148,-1.389532103288,0.07282787068199));
#17875=CARTESIAN_POINT('Ctrl Pts',(27.97448943148,-1.034052055861,0.9310606109295));
#17876=CARTESIAN_POINT('Ctrl Pts',(27.92573943148,-0.2176699703233,1.374319545129));
#17877=CARTESIAN_POINT('Ctrl Pts',(27.87698943148,0.6957249084783,1.205031167107));
#17878=CARTESIAN_POINT('Ctrl Pts',(27.82823943148,1.299030774048,0.4986511981072));
#17879=CARTESIAN_POINT('Ctrl Pts',(27.77948943148,1.323347810262,-0.4299817804464));
#17880=CARTESIAN_POINT('Ctrl Pts',(27.73073943148,0.757838124655,-1.166968368163));
#17881=CARTESIAN_POINT('Ctrl Pts',(27.68198943148,-0.1454461572801,-1.383827738746));
#17882=CARTESIAN_POINT('Ctrl Pts',(27.63323943148,-0.9839039059594,-0.9839039061246));
#17883=CARTESIAN_POINT('Ctrl Pts',(27.58448943148,-1.383827738331,-0.1454461562038));
#17884=CARTESIAN_POINT('Ctrl Pts',(27.53573943148,-1.166968369989,0.7578381205156));
#17885=CARTESIAN_POINT('Ctrl Pts',(27.48698943148,-0.4299817735579,1.323347825744));
#17886=CARTESIAN_POINT('Ctrl Pts',(27.43823943148,0.4986511723796,1.299030716259));
#17887=CARTESIAN_POINT('Ctrl Pts',(27.38948943148,1.20503126313,0.6957251241499));
#17888=CARTESIAN_POINT('Ctrl Pts',(27.34073943148,1.374319186766,-0.2176707752221));
#17889=CARTESIAN_POINT('Ctrl Pts',(27.29198943148,0.9310619483586,-1.034049051938));
#17890=CARTESIAN_POINT('Ctrl Pts',(27.24323943148,0.0728228793282,-1.389543314081));
#17891=CARTESIAN_POINT('Ctrl Pts',(27.19448943148,-0.8178739353207,-1.125706897754));
#17892=CARTESIAN_POINT('Ctrl Pts',(27.14573943148,-1.344037730566,-0.3601338243812));
#17893=CARTESIAN_POINT('Ctrl Pts',(27.09698943148,-1.271153054855,0.5659538022856));
#17894=CARTESIAN_POINT('Ctrl Pts',(27.04823943148,-0.6317051899144,1.239791251989));
#17895=CARTESIAN_POINT('Ctrl Pts',(26.99948943148,0.2892987601003,1.361043711953));
#17896=CARTESIAN_POINT('Ctrl Pts',(26.95073943148,1.081359992212,0.8756680515693));
#17897=CARTESIAN_POINT('Ctrl Pts',(26.90198943148,1.391450057306,-1.387659428753E-7));
#17898=CARTESIAN_POINT('Ctrl Pts',(26.85323943148,1.081360653838,-0.8756674965058));
#17899=CARTESIAN_POINT('Ctrl Pts',(26.80448943148,0.2892961135976,-1.361045654676));
#17900=CARTESIAN_POINT('Ctrl Pts',(26.75573943148,-0.6316952655301,-1.239784036163));
#17901=CARTESIAN_POINT('Ctrl Pts',(26.70698943148,-1.271190105891,-0.5659807228688));
#17902=CARTESIAN_POINT('Ctrl Pts',(26.65823943148,-1.34389945081,0.360234290888));
#17903=CARTESIAN_POINT('Ctrl Pts',(26.62573943148,-0.9935598191429,0.8702993985029));
#17904=CARTESIAN_POINT('Ctrl Pts',(26.60948943148,-0.7571184320867,1.04208412158));
#17905=CARTESIAN_POINT('Ctrl Pts',(28.1078719886,0.4805033243013,-1.079228136364));
#17906=CARTESIAN_POINT('Ctrl Pts',(28.0916219886,0.235634227625,-1.18825088235));
#17907=CARTESIAN_POINT('Ctrl Pts',(28.0591219886,-0.330151697238,-1.232613610374));
#17908=CARTESIAN_POINT('Ctrl Pts',(28.0103719886,-1.032474730272,-0.7501260058613));
#17909=CARTESIAN_POINT('Ctrl Pts',(27.9616219886,-1.274402303455,0.06679371130266));
#17910=CARTESIAN_POINT('Ctrl Pts',(27.9128719886,-0.9483755853946,0.8539175053361));
#17911=CARTESIAN_POINT('Ctrl Pts',(27.8641219886,-0.199634906539,1.260450183087));
#17912=CARTESIAN_POINT('Ctrl Pts',(27.8153719886,0.6380805623974,1.105188207931));
#17913=CARTESIAN_POINT('Ctrl Pts',(27.7666219886,1.191399469495,0.4573354109519));
#17914=CARTESIAN_POINT('Ctrl Pts',(27.7178719886,1.21370171562,-0.394355603694));
#17915=CARTESIAN_POINT('Ctrl Pts',(27.6691219886,0.6950473827992,-1.07027910541));
#17916=CARTESIAN_POINT('Ctrl Pts',(27.6203719886,-0.1333952036284,-1.269170574518));
#17917=CARTESIAN_POINT('Ctrl Pts',(27.5716219886,-0.902382464691,-0.9023824648425));
#17918=CARTESIAN_POINT('Ctrl Pts',(27.5228719886,-1.269170574137,-0.1333952026413));
#17919=CARTESIAN_POINT('Ctrl Pts',(27.4741219886,-1.070279107084,0.6950473790028));
#17920=CARTESIAN_POINT('Ctrl Pts',(27.4253719886,-0.3943555973762,1.213701729819));
#17921=CARTESIAN_POINT('Ctrl Pts',(27.3766219886,0.4573353873559,1.191399416495));
#17922=CARTESIAN_POINT('Ctrl Pts',(27.3278719886,1.105188295998,0.6380807601996));
#17923=CARTESIAN_POINT('Ctrl Pts',(27.2791219886,1.260449854417,-0.1996356447478));
#17924=CARTESIAN_POINT('Ctrl Pts',(27.2303719886,0.8539187319524,-0.9483728303621));
#17925=CARTESIAN_POINT('Ctrl Pts',(27.1816219886,0.06678913350791,-1.274412585376));
#17926=CARTESIAN_POINT('Ctrl Pts',(27.1328719886,-0.7501089212991,-1.032436357618));
#17927=CARTESIAN_POINT('Ctrl Pts',(27.0841219886,-1.232677370829,-0.3302949059307));
#17928=CARTESIAN_POINT('Ctrl Pts',(27.0353719886,-1.165831561083,0.519061652174));
#17929=CARTESIAN_POINT('Ctrl Pts',(26.9866219886,-0.5793652030248,1.137068243043));
#17930=CARTESIAN_POINT('Ctrl Pts',(26.9378719886,0.2653288868863,1.248274320191));
#17931=CARTESIAN_POINT('Ctrl Pts',(26.8891219886,0.9917638186823,0.8031145011623));
#17932=CARTESIAN_POINT('Ctrl Pts',(26.8403719886,1.27616134523,-1.272684787665E-7));
#17933=CARTESIAN_POINT('Ctrl Pts',(26.7916219886,0.9917644254889,-0.8031139920887));
#17934=CARTESIAN_POINT('Ctrl Pts',(26.7428719886,0.2653264596599,-1.248276101949));
#17935=CARTESIAN_POINT('Ctrl Pts',(26.6941219886,-0.5793561009262,-1.137061625084));
#17936=CARTESIAN_POINT('Ctrl Pts',(26.6453719886,-1.165865542251,-0.51908634225));
#17937=CARTESIAN_POINT('Ctrl Pts',(26.5966219886,-1.232550548254,0.3303870482766));
#17938=CARTESIAN_POINT('Ctrl Pts',(26.5641219886,-0.9112383363717,0.7981906682994));
#17939=CARTESIAN_POINT('Ctrl Pts',(26.5478719886,-0.6943873204195,0.9557421536299));
#17940=CARTESIAN_POINT('Ctrl Pts',(28.04625454572,0.4370945424776,-0.9817304160777));
#17941=CARTESIAN_POINT('Ctrl Pts',(28.03000454572,0.2143469768197,-1.080904021891));
#17942=CARTESIAN_POINT('Ctrl Pts',(27.99750454572,-0.3003257162941,-1.121259010771));
#17943=CARTESIAN_POINT('Ctrl Pts',(27.94875454572,-0.9392007235413,-0.6823594484165));
#17944=CARTESIAN_POINT('Ctrl Pts',(27.90000454572,-1.159272503621,0.06075955192333));
#17945=CARTESIAN_POINT('Ctrl Pts',(27.85125454572,-0.8626991149286,0.7767743997427));
#17946=CARTESIAN_POINT('Ctrl Pts',(27.80250454572,-0.1815998427547,1.146580821045));
#17947=CARTESIAN_POINT('Ctrl Pts',(27.75375454572,0.5804362163165,1.005345248755));
#17948=CARTESIAN_POINT('Ctrl Pts',(27.70500454572,1.083768164943,0.4160196237966));
#17949=CARTESIAN_POINT('Ctrl Pts',(27.65625454572,1.104055620977,-0.3587294269415));
#17950=CARTESIAN_POINT('Ctrl Pts',(27.60750454572,0.6322566409434,-0.9735898426565));
#17951=CARTESIAN_POINT('Ctrl Pts',(27.55875454572,-0.1213442499767,-1.154513410291));
#17952=CARTESIAN_POINT('Ctrl Pts',(27.51000454572,-0.8208610234226,-0.8208610235604));
#17953=CARTESIAN_POINT('Ctrl Pts',(27.46125454572,-1.154513409944,-0.1213442490788));
#17954=CARTESIAN_POINT('Ctrl Pts',(27.41250454572,-0.9735898441798,0.6322566374899));
#17955=CARTESIAN_POINT('Ctrl Pts',(27.36375454572,-0.3587294211945,1.104055633894));
#17956=CARTESIAN_POINT('Ctrl Pts',(27.31500454572,0.4160196023323,1.083768116731));
#17957=CARTESIAN_POINT('Ctrl Pts',(27.26625454572,1.005345328866,0.5804363962492));
#17958=CARTESIAN_POINT('Ctrl Pts',(27.21750454572,1.146580522067,-0.1816005142735));
#17959=CARTESIAN_POINT('Ctrl Pts',(27.16875454572,0.7767755155462,-0.8626966087864));
#17960=CARTESIAN_POINT('Ctrl Pts',(27.12000454572,0.06075538768762,-1.159281856671));
#17961=CARTESIAN_POINT('Ctrl Pts',(27.07125454572,-0.6823439072776,-0.9391658174821));
#17962=CARTESIAN_POINT('Ctrl Pts',(27.02250454572,-1.121317011091,-0.3004559874802));
#17963=CARTESIAN_POINT('Ctrl Pts',(26.97375454572,-1.06051006731,0.4721695020624));
#17964=CARTESIAN_POINT('Ctrl Pts',(26.92500454572,-0.5270252161352,1.034345234097));
#17965=CARTESIAN_POINT('Ctrl Pts',(26.87625454572,0.2413590136724,1.135504928428));
#17966=CARTESIAN_POINT('Ctrl Pts',(26.82750454572,0.9021676451524,0.7305609507554));
#17967=CARTESIAN_POINT('Ctrl Pts',(26.77875454572,1.160872633154,-1.157710151699E-7));
#17968=CARTESIAN_POINT('Ctrl Pts',(26.73000454572,0.9021681971399,-0.7305604876716));
#17969=CARTESIAN_POINT('Ctrl Pts',(26.68125454572,0.2413568057222,-1.135506549222));
#17970=CARTESIAN_POINT('Ctrl Pts',(26.63250454572,-0.5270169363223,-1.034339214006));
#17971=CARTESIAN_POINT('Ctrl Pts',(26.58375454572,-1.060540978612,-0.4721919616312));
#17972=CARTESIAN_POINT('Ctrl Pts',(26.53500454572,-1.121201645697,0.3005398056652));
#17973=CARTESIAN_POINT('Ctrl Pts',(26.50250454572,-0.8289168536006,0.726081938096));
#17974=CARTESIAN_POINT('Ctrl Pts',(26.48625454572,-0.6316562087523,0.86940018568));
#17975=CARTESIAN_POINT('Ctrl Pts',(27.98463710284,0.3936857606539,-0.8842326957913));
#17976=CARTESIAN_POINT('Ctrl Pts',(27.96838710284,0.1930597260145,-0.9735571614325));
#17977=CARTESIAN_POINT('Ctrl Pts',(27.93588710284,-0.2704997353501,-1.009904411168));
#17978=CARTESIAN_POINT('Ctrl Pts',(27.88713710284,-0.845926716811,-0.6145928909716));
#17979=CARTESIAN_POINT('Ctrl Pts',(27.83838710284,-1.044142703787,0.054725392544));
#17980=CARTESIAN_POINT('Ctrl Pts',(27.78963710284,-0.7770226444626,0.6996312941493));
#17981=CARTESIAN_POINT('Ctrl Pts',(27.74088710284,-0.1635647789704,1.032711459003));
#17982=CARTESIAN_POINT('Ctrl Pts',(27.69213710284,0.5227918702356,0.9055022895789));
#17983=CARTESIAN_POINT('Ctrl Pts',(27.64338710284,0.9761368603912,0.3747038366413));
#17984=CARTESIAN_POINT('Ctrl Pts',(27.59463710284,0.9944095263349,-0.3231032501891));
#17985=CARTESIAN_POINT('Ctrl Pts',(27.54588710284,0.5694658990876,-0.8769005799033));
#17986=CARTESIAN_POINT('Ctrl Pts',(27.49713710284,-0.109293296325,-1.039856246063));
#17987=CARTESIAN_POINT('Ctrl Pts',(27.44838710284,-0.7393395821542,-0.7393395822784));
#17988=CARTESIAN_POINT('Ctrl Pts',(27.39963710284,-1.039856245751,-0.1092932955163));
#17989=CARTESIAN_POINT('Ctrl Pts',(27.35088710284,-0.8769005812753,0.5694658959771));
#17990=CARTESIAN_POINT('Ctrl Pts',(27.30213710284,-0.3231032450128,0.9944095379687));
#17991=CARTESIAN_POINT('Ctrl Pts',(27.25338710284,0.3747038173086,0.9761368169669));
#17992=CARTESIAN_POINT('Ctrl Pts',(27.20463710284,0.9055023617338,0.5227920322988));
#17993=CARTESIAN_POINT('Ctrl Pts',(27.15588710284,1.032711189717,-0.1635653837993));
#17994=CARTESIAN_POINT('Ctrl Pts',(27.10713710284,0.69963229914,-0.7770203872107));
#17995=CARTESIAN_POINT('Ctrl Pts',(27.05838710284,0.05472164186733,-1.044151127966));
#17996=CARTESIAN_POINT('Ctrl Pts',(27.00963710284,-0.6145788932561,-0.8458952773462));
#17997=CARTESIAN_POINT('Ctrl Pts',(26.96088710284,-1.009956651354,-0.2706170690297));
#17998=CARTESIAN_POINT('Ctrl Pts',(26.91213710284,-0.9551885735371,0.4252773519508));
#17999=CARTESIAN_POINT('Ctrl Pts',(26.86338710284,-0.4746852292456,0.9316222251505));
#18000=CARTESIAN_POINT('Ctrl Pts',(26.81463710284,0.2173891404585,1.022735536666));
#18001=CARTESIAN_POINT('Ctrl Pts',(26.76588710284,0.8125714716225,0.6580074003485));
#18002=CARTESIAN_POINT('Ctrl Pts',(26.71713710284,1.045583921078,-1.042735511825E-7));
#18003=CARTESIAN_POINT('Ctrl Pts',(26.66838710284,0.8125719687909,-0.6580069832545));
#18004=CARTESIAN_POINT('Ctrl Pts',(26.61963710284,0.2173871517845,-1.022736996495));
#18005=CARTESIAN_POINT('Ctrl Pts',(26.57088710284,-0.4746777717184,-0.9316168029278));
#18006=CARTESIAN_POINT('Ctrl Pts',(26.52213710284,-0.9552164149723,-0.4252975810124));
#18007=CARTESIAN_POINT('Ctrl Pts',(26.47338710284,-1.00985274314,0.2706925630538));
#18008=CARTESIAN_POINT('Ctrl Pts',(26.44088710284,-0.7465953708295,0.6539732078925));
#18009=CARTESIAN_POINT('Ctrl Pts',(26.42463710284,-0.568925097085,0.7830582177302));
#18010=CARTESIAN_POINT('',(26.4799708243305,-0.893567698107012,0.46113007932394));
#18011=CARTESIAN_POINT('Ctrl Pts',(27.9766422174339,-1.5373237190809E-6,
-1.00548643891288));
#18012=CARTESIAN_POINT('Ctrl Pts',(27.9705255346309,-0.0859077806927734,
-1.00562089711478));
#18013=CARTESIAN_POINT('Ctrl Pts',(27.9644038376714,-0.171834166064752,
-0.994932640726613));
#18014=CARTESIAN_POINT('Ctrl Pts',(27.9521313122326,-0.338307248628255,
-0.951321255208717));
#18015=CARTESIAN_POINT('Ctrl Pts',(27.9459996491108,-0.41859324830683,-0.918352377669841));
#18016=CARTESIAN_POINT('Ctrl Pts',(27.9308010923912,-0.604507474757968,
-0.813185183941887));
#18017=CARTESIAN_POINT('Ctrl Pts',(27.9217162790432,-0.70401704675962,-0.729489940877468));
#18018=CARTESIAN_POINT('Ctrl Pts',(27.9004547199262,-0.891186104950947,
-0.497397527776343));
#18019=CARTESIAN_POINT('Ctrl Pts',(27.8906214013537,-0.941335991090675,
-0.364860551214267));
#18020=CARTESIAN_POINT('Ctrl Pts',(27.8766754648128,-0.995276073891188,
-0.176341402154162));
#18021=CARTESIAN_POINT('Ctrl Pts',(27.867508386247,-1.01642369245459,-0.0467042547600237));
#18022=CARTESIAN_POINT('Ctrl Pts',(27.8472694827219,-0.986706480683557,
0.235516124889919));
#18023=CARTESIAN_POINT('Ctrl Pts',(27.8378314007197,-0.946071719962327,
0.364715479070765));
#18024=CARTESIAN_POINT('Ctrl Pts',(27.8214313439974,-0.836161765852973,
0.567325413516962));
#18025=CARTESIAN_POINT('Ctrl Pts',(27.8119819791548,-0.760098085984591,
0.679268787558479));
#18026=CARTESIAN_POINT('Ctrl Pts',(27.7910321513064,-0.530789606151427,
0.863653013790982));
#18027=CARTESIAN_POINT('Ctrl Pts',(27.7817681502791,-0.413223717409633,
0.925788399292649));
#18028=CARTESIAN_POINT('Ctrl Pts',(27.7679188615263,-0.227184383092205,
0.982048937828046));
#18029=CARTESIAN_POINT('Ctrl Pts',(27.7633615602744,-0.164380263775081,
0.994628768871488));
#18030=CARTESIAN_POINT('Ctrl Pts',(27.7493060807227,0.0316682215204115,
1.01386448246957));
#18031=CARTESIAN_POINT('Ctrl Pts',(27.7398895019711,0.166239806421696,1.00019965980914));
#18032=CARTESIAN_POINT('Ctrl Pts',(27.722948630156,0.39422446910652,0.931294753093088));
#18033=CARTESIAN_POINT('Ctrl Pts',(27.7135806633062,0.516769776937294,0.87757223757841));
#18034=CARTESIAN_POINT('Ctrl Pts',(27.6930688620494,0.738867116514401,0.693970728769147));
#18035=CARTESIAN_POINT('Ctrl Pts',(27.6838346853022,0.823293763365346,0.5916217309268));
#18036=CARTESIAN_POINT('Ctrl Pts',(27.6699847101733,0.91597535503147,0.420829660664151));
#18037=CARTESIAN_POINT('Ctrl Pts',(27.6654152401922,0.940974162891107,0.361768629684782));
#18038=CARTESIAN_POINT('Ctrl Pts',(27.6513591638085,0.999311500696718,0.173674766097076));
#18039=CARTESIAN_POINT('Ctrl Pts',(27.6419654083536,1.01314003710848,0.039311455778221));
#18040=CARTESIAN_POINT('Ctrl Pts',(27.6231252836627,0.989400550382701,-0.22455377395045));
#18041=CARTESIAN_POINT('Ctrl Pts',(27.6138328999225,0.951988050045546,-0.351293863160414));
#18042=CARTESIAN_POINT('Ctrl Pts',(27.595128759979,0.828821871769212,-0.583495916260747));
#18043=CARTESIAN_POINT('Ctrl Pts',(27.5859242982163,0.745869543467991,-0.6866586081706));
#18044=CARTESIAN_POINT('Ctrl Pts',(27.5720731185926,0.597410474983936,-0.811959898152375));
#18045=CARTESIAN_POINT('Ctrl Pts',(27.5674917366428,0.544541205515937,-0.84839663720727));
#18046=CARTESIAN_POINT('Ctrl Pts',(27.5534388142855,0.372180503743955,-0.943469506501608));
#18047=CARTESIAN_POINT('Ctrl Pts',(27.5440688767006,0.243602562677523,-0.984185395931866));
#18048=CARTESIAN_POINT('Ctrl Pts',(27.5252181077583,-0.019790956493,-1.01445554834801));
#18049=CARTESIAN_POINT('Ctrl Pts',(27.5159060230867,-0.151558042053847,
-1.00333391119788));
#18050=CARTESIAN_POINT('Ctrl Pts',(27.4972207684037,-0.403699692496189,
-0.929699387128286));
#18051=CARTESIAN_POINT('Ctrl Pts',(27.4880454718056,-0.521279955364169,
-0.869530077180673));
#18052=CARTESIAN_POINT('Ctrl Pts',(27.4741927612439,-0.674040239658134,
-0.74960673165156));
#18053=CARTESIAN_POINT('Ctrl Pts',(27.4695997466732,-0.720459910529298,
-0.705142509973364));
#18054=CARTESIAN_POINT('Ctrl Pts',(27.4555529346347,-0.848377502645995,
-0.555681059924086));
#18055=CARTESIAN_POINT('Ctrl Pts',(27.4462074184943,-0.914262872089956,
-0.438238959868308));
#18056=CARTESIAN_POINT('Ctrl Pts',(27.4273501142183,-0.997461472283246,
-0.186370890415201));
#18057=CARTESIAN_POINT('Ctrl Pts',(27.418014468959,-1.01320279607384,-0.0549322312585341));
#18058=CARTESIAN_POINT('Ctrl Pts',(27.3993516905516,-0.992221655655208,
0.206690030888449));
#18059=CARTESIAN_POINT('Ctrl Pts',(27.3902046226188,-0.957291168985145,
0.333772807407334));
#18060=CARTESIAN_POINT('Ctrl Pts',(27.3763512181046,-0.870967954992039,
0.50764905831));
#18061=CARTESIAN_POINT('Ctrl Pts',(27.3717448653341,-0.836781532034192,
0.562196601259316));
#18062=CARTESIAN_POINT('Ctrl Pts',(27.3577073802788,-0.716486421177458,
0.71767212754246));
#18063=CARTESIAN_POINT('Ctrl Pts',(27.3483865423645,-0.615086538827653,
0.805957361969493));
#18064=CARTESIAN_POINT('Ctrl Pts',(27.3295286233357,-0.38542249522935,0.93874078967969));
#18065=CARTESIAN_POINT('Ctrl Pts',(27.3201620212027,-0.259667379149739,
0.980868466998606));
#18066=CARTESIAN_POINT('Ctrl Pts',(27.301526323939,0.000490033357717634,
1.01348106517059));
#18067=CARTESIAN_POINT('Ctrl Pts',(27.2924062511612,0.131755232397248,1.00521032755393));
#18068=CARTESIAN_POINT('Ctrl Pts',(27.2785538277661,0.319464250831635,0.95617772108636));
#18069=CARTESIAN_POINT('Ctrl Pts',(27.2739310443358,0.379954363604974,0.933743418142628));
#18070=CARTESIAN_POINT('Ctrl Pts',(27.2645824710877,0.497634642074296,0.876392064260345));
#18071=CARTESIAN_POINT('Ctrl Pts',(27.2598914483125,0.55413873606994,0.841549933535181));
#18072=CARTESIAN_POINT('Ctrl Pts',(27.2462803892375,0.707134147413743,0.725557967358108));
#18073=CARTESIAN_POINT('Ctrl Pts',(27.237362246922,0.793622219861324,0.630917404931592));
#18074=CARTESIAN_POINT('Ctrl Pts',(27.2238373535096,0.891630461095201,0.470034499211284));
#18075=CARTESIAN_POINT('Ctrl Pts',(27.2193698487091,0.918935033135005,0.41356732956778));
#18076=CARTESIAN_POINT('Ctrl Pts',(27.2055606395873,0.987004581363573,0.231746318671411));
#18077=CARTESIAN_POINT('Ctrl Pts',(27.1962633766506,1.00922718171059,0.0992152525598969));
#18078=CARTESIAN_POINT('Ctrl Pts',(27.1822401043235,1.00340136620523,-0.0972176553217059));
#18079=CARTESIAN_POINT('Ctrl Pts',(27.1776216056682,0.9951638680146,-0.161078166755552));
#18080=CARTESIAN_POINT('Ctrl Pts',(27.1637406949851,0.951401802556867,-0.350214922113325));
#18081=CARTESIAN_POINT('Ctrl Pts',(27.1546119632471,0.897664854294904,-0.470552356748959));
#18082=CARTESIAN_POINT('Ctrl Pts',(27.1359749150596,0.747685981774503,-0.68597793018104));
#18083=CARTESIAN_POINT('Ctrl Pts',(27.1265959280299,0.652004951410655,-0.777543331604733));
#18084=CARTESIAN_POINT('Ctrl Pts',(27.1077449073936,0.427849061677098,-0.919147495175399));
#18085=CARTESIAN_POINT('Ctrl Pts',(27.0984509493297,0.302542158836555,-0.967956149819254));
#18086=CARTESIAN_POINT('Ctrl Pts',(27.0844210573905,0.1090489926338,-1.00219031322694));
#18087=CARTESIAN_POINT('Ctrl Pts',(27.0798076083915,0.0450129822140624,
-1.00708214754234));
#18088=CARTESIAN_POINT('Ctrl Pts',(27.0659280179578,-0.149048344906606,
-1.00279330227197));
#18089=CARTESIAN_POINT('Ctrl Pts',(27.0567949468168,-0.278033405463916,
-0.974675255245754));
#18090=CARTESIAN_POINT('Ctrl Pts',(27.0381489605883,-0.519590955197979,
-0.871589515518927));
#18091=CARTESIAN_POINT('Ctrl Pts',(27.028767681825,-0.628508797564383,-0.796566723643565));
#18092=CARTESIAN_POINT('Ctrl Pts',(27.00994229388,-0.812678040764659,-0.606170204142176));
#18093=CARTESIAN_POINT('Ctrl Pts',(27.0006529512941,-0.886066522647178,
-0.493396421490482));
#18094=CARTESIAN_POINT('Ctrl Pts',(26.9866194370948,-0.958938614597588,
-0.310992833312596));
#18095=CARTESIAN_POINT('Ctrl Pts',(26.9820091985959,-0.97671250646186,-0.249421384271684));
#18096=CARTESIAN_POINT('Ctrl Pts',(26.9681351506143,-1.0121086090019,-0.0586423619505615));
#18097=CARTESIAN_POINT('Ctrl Pts',(26.9589993728496,-1.01091662374079,0.0735675041066844));
#18098=CARTESIAN_POINT('Ctrl Pts',(26.9403491684073,-0.959179498422769,
0.331121220497063));
#18099=CARTESIAN_POINT('Ctrl Pts',(26.9309611376611,-0.907891952129337,
0.452903835131262));
#18100=CARTESIAN_POINT('Ctrl Pts',(26.9121666250875,-0.759302137912035,
0.671823573379696));
#18101=CARTESIAN_POINT('Ctrl Pts',(26.9028834236569,-0.663875135361441,
0.766745789531095));
#18102=CARTESIAN_POINT('Ctrl Pts',(26.8888483303339,-0.500262661165281,
0.875221855367422));
#18103=CARTESIAN_POINT('Ctrl Pts',(26.8842421532104,-0.443733473377021,
0.905105546364918));
#18104=CARTESIAN_POINT('Ctrl Pts',(26.8703760201451,-0.264322102188032,
0.978738236522294));
#18105=CARTESIAN_POINT('Ctrl Pts',(26.8612394304227,-0.134496425536785,
1.00465935483348));
#18106=CARTESIAN_POINT('Ctrl Pts',(26.8425874128787,0.12821796553708,1.00659844603438));
#18107=CARTESIAN_POINT('Ctrl Pts',(26.8331935286416,0.257776737069651,0.98122067919966));
#18108=CARTESIAN_POINT('Ctrl Pts',(26.8144314676225,0.502179497876163,0.880737299645244));
#18109=CARTESIAN_POINT('Ctrl Pts',(26.8051560975335,0.614658956622138,0.806776652592242));
#18110=CARTESIAN_POINT('Ctrl Pts',(26.7911216829485,0.754198706932562,0.668917525005024));
#18111=CARTESIAN_POINT('Ctrl Pts',(26.7865203133558,0.794916339912257,0.619808451467912));
#18112=CARTESIAN_POINT('Ctrl Pts',(26.7726637815399,0.903723053949885,0.459423824527641));
#18113=CARTESIAN_POINT('Ctrl Pts',(26.7635284434174,0.955795481190457,0.337553314734785));
#18114=CARTESIAN_POINT('Ctrl Pts',(26.7430671285445,1.01691671680807,0.0559092551204978));
#18115=CARTESIAN_POINT('Ctrl Pts',(26.7335726504057,1.00827361012557,-0.0774627611606082));
#18116=CARTESIAN_POINT('Ctrl Pts',(26.7167489140092,0.96510418020808,-0.310561847663239));
#18117=CARTESIAN_POINT('Ctrl Pts',(26.7074831618654,0.915855808452785,-0.43583755702115));
#18118=CARTESIAN_POINT('Ctrl Pts',(26.6934517331005,0.809682273584885,-0.600555290111322));
#18119=CARTESIAN_POINT('Ctrl Pts',(26.6888556296663,0.770074228022994,-0.650371937404803));
#18120=CARTESIAN_POINT('Ctrl Pts',(26.675009634705,0.63563363352959,-0.789775672636881));
#18121=CARTESIAN_POINT('Ctrl Pts',(26.6658776811606,0.527018763233726,-0.865902447959457));
#18122=CARTESIAN_POINT('Ctrl Pts',(26.6451332237827,0.260335337877291,-0.985279478959959));
#18123=CARTESIAN_POINT('Ctrl Pts',(26.6356306855464,0.12774312417312,-1.00266395438481));
#18124=CARTESIAN_POINT('Ctrl Pts',(26.6191285504318,-0.10481767593479,-1.00840079955666));
#18125=CARTESIAN_POINT('Ctrl Pts',(26.6098742312728,-0.237527656582644,
-0.986082378766112));
#18126=CARTESIAN_POINT('Ctrl Pts',(26.5958478040773,-0.420419005484187,
-0.916233293702868));
#18127=CARTESIAN_POINT('Ctrl Pts',(26.5912565838117,-0.477212390052805,
-0.887817863142468));
#18128=CARTESIAN_POINT('Ctrl Pts',(26.5774207798424,-0.64129015998728,-0.785193009416701));
#18129=CARTESIAN_POINT('Ctrl Pts',(26.5682937239647,-0.738299711072096,
-0.694631109053306));
#18130=CARTESIAN_POINT('Ctrl Pts',(26.5474252312128,-0.911213333992815,
-0.456976015197982));
#18131=CARTESIAN_POINT('Ctrl Pts',(26.5378160228461,-0.955228839604515,
-0.329238910539293));
#18132=CARTESIAN_POINT('Ctrl Pts',(26.5225016105883,-1.0051919273077,-0.119087333308766));
#18133=CARTESIAN_POINT('Ctrl Pts',(26.5141604723334,-1.01252416824994,0.00158815197311223));
#18134=CARTESIAN_POINT('Ctrl Pts',(26.5013873245562,-0.991708199632223,
0.179309126855524));
#18135=CARTESIAN_POINT('Ctrl Pts',(26.4970734565504,-0.979393895210917,
0.237713999577028));
#18136=CARTESIAN_POINT('Ctrl Pts',(26.4884634191094,-0.944019929726152,
0.352096395825399));
#18137=CARTESIAN_POINT('Ctrl Pts',(26.4842212099352,-0.921272789443298,
0.407435861295654));
#18138=CARTESIAN_POINT('Ctrl Pts',(26.48,-0.8939005627167,0.460377710173328));
#18139=CARTESIAN_POINT('',(26.4800266000133,-0.875887823837977,0.505699775546759));
#18140=CARTESIAN_POINT('Ctrl Pts',(26.48,-0.893613512752342,0.4611507504989));
#18141=CARTESIAN_POINT('Ctrl Pts',(26.48,-0.89081917574886,0.468666621828444));
#18142=CARTESIAN_POINT('Ctrl Pts',(26.48,-0.887935158142909,0.476149169831144));
#18143=CARTESIAN_POINT('Ctrl Pts',(26.48,-0.882010577760306,0.490993452370655));
#18144=CARTESIAN_POINT('Ctrl Pts',(26.48,-0.878971184435156,0.498355708662359));
#18145=CARTESIAN_POINT('Ctrl Pts',(26.48,-0.875845991678543,0.505681328412502));
#18146=CARTESIAN_POINT('',(26.6175803212394,-1.08239526302019,0.624914431681246));
#18147=CARTESIAN_POINT('Ctrl Pts',(26.6177473887885,-1.08236453146925,0.624903453604815));
#18148=CARTESIAN_POINT('Ctrl Pts',(26.5948291214948,-1.04800484136653,0.605065877274762));
#18149=CARTESIAN_POINT('Ctrl Pts',(26.5719108542008,-1.01364515126075,0.58522830095031));
#18150=CARTESIAN_POINT('Ctrl Pts',(26.5260127912802,-0.944833526103479,
0.545499890642383));
#18151=CARTESIAN_POINT('Ctrl Pts',(26.5030329956536,-0.910381591051974,
0.525609056658872));
#18152=CARTESIAN_POINT('Ctrl Pts',(26.4800532000267,-0.87592965599741,0.505718222681016));
#18153=CARTESIAN_POINT('Ctrl Pts',(26.6176729436514,-1.08225296268473,0.62483892430428));
#18154=CARTESIAN_POINT('Ctrl Pts',(26.6233229277769,-1.13222243988375,0.538356821464131));
#18155=CARTESIAN_POINT('Ctrl Pts',(26.628840140606,-1.17178227932954,0.445892888274432));
#18156=CARTESIAN_POINT('Ctrl Pts',(26.6398126160615,-1.22565723371071,0.261226310700327));
#18157=CARTESIAN_POINT('Ctrl Pts',(26.6452637354378,-1.24149712443581,0.169751315722489));
#18158=CARTESIAN_POINT('Ctrl Pts',(26.6602924600519,-1.25737930305406,-0.0862086344073024));
#18159=CARTESIAN_POINT('Ctrl Pts',(26.6685515184089,-1.23440178668179,-0.235205427087828));
#18160=CARTESIAN_POINT('Ctrl Pts',(26.6850772214207,-1.14935312334068,-0.516442894477973));
#18161=CARTESIAN_POINT('Ctrl Pts',(26.693633133589,-1.07866597598953,-0.644497028069737));
#18162=CARTESIAN_POINT('Ctrl Pts',(26.705952000928,-0.951273837925217,-0.814528408486582));
#18163=CARTESIAN_POINT('Ctrl Pts',(26.7106361966476,-0.895018277429958,
-0.87577575106266));
#18164=CARTESIAN_POINT('Ctrl Pts',(26.7206751402919,-0.762322350473856,
-0.994581826367339));
#18165=CARTESIAN_POINT('Ctrl Pts',(26.7260298582995,-0.684068404833238,
-1.05018828899575));
#18166=CARTESIAN_POINT('Ctrl Pts',(26.7355561252237,-0.53891920407384,-1.12995717925848));
#18167=CARTESIAN_POINT('Ctrl Pts',(26.7396608009472,-0.474911111502257,
-1.15829422468238));
#18168=CARTESIAN_POINT('Ctrl Pts',(26.7530210523164,-0.25800087723676,-1.23305883785933));
#18169=CARTESIAN_POINT('Ctrl Pts',(26.7619861989868,-0.0972512468538276,
-1.25562451060708));
#18170=CARTESIAN_POINT('Ctrl Pts',(26.7803410435921,0.225443202719235,-1.24029034488642));
#18171=CARTESIAN_POINT('Ctrl Pts',(26.7896883750463,0.383702507178638,-1.2007301368539));
#18172=CARTESIAN_POINT('Ctrl Pts',(26.80382706628,0.606433346984284,-1.0954489537623));
#18173=CARTESIAN_POINT('Ctrl Pts',(26.8085441969838,0.677671505270773,-1.05281147333592));
#18174=CARTESIAN_POINT('Ctrl Pts',(26.8199336274881,0.838263677832852,-0.934102162227965));
#18175=CARTESIAN_POINT('Ctrl Pts',(26.829328142703,0.964516250915906,-0.821620611431171));
#18176=CARTESIAN_POINT('Ctrl Pts',(26.8504869605049,1.15343023316433,-0.506482220582575));
#18177=CARTESIAN_POINT('Ctrl Pts',(26.8598366313787,1.20978204209892,-0.351570030074152));
#18178=CARTESIAN_POINT('Ctrl Pts',(26.8737389494541,1.2478031354602,-0.110426880252088));
#18179=CARTESIAN_POINT('Ctrl Pts',(26.8783363175325,1.2524274771249,-0.0283093125836477));
#18180=CARTESIAN_POINT('Ctrl Pts',(26.8918898714561,1.24172752266081,0.208333288214192));
#18181=CARTESIAN_POINT('Ctrl Pts',(26.9009488769085,1.2058442502652,0.361223885151522));
#18182=CARTESIAN_POINT('Ctrl Pts',(26.9190682007871,1.07937320915612,0.650515496858714));
#18183=CARTESIAN_POINT('Ctrl Pts',(26.9277929791483,0.987506469895415,0.783029094899924));
#18184=CARTESIAN_POINT('Ctrl Pts',(26.9454649798215,0.768868859633136,0.995161173191032));
#18185=CARTESIAN_POINT('Ctrl Pts',(26.9547722464512,0.638107577335029,1.08803878674962));
#18186=CARTESIAN_POINT('Ctrl Pts',(26.9684941446703,0.412490985363296,1.18199876591539));
#18187=CARTESIAN_POINT('Ctrl Pts',(26.9725362315898,0.342875121890448,1.20407214480854));
#18188=CARTESIAN_POINT('Ctrl Pts',(26.9813229028305,0.192126306293707,1.23759666842505));
#18189=CARTESIAN_POINT('Ctrl Pts',(26.9861010085444,0.110744116420164,1.24736969716722));
#18190=CARTESIAN_POINT('Ctrl Pts',(26.9957932142666,-0.0546765437387625,
1.2511707678145));
#18191=CARTESIAN_POINT('Ctrl Pts',(27.0007125467791,-0.138968930008962,
1.24471180503867));
#18192=CARTESIAN_POINT('Ctrl Pts',(27.0138122303823,-0.366001853172527,
1.20378429434567));
#18193=CARTESIAN_POINT('Ctrl Pts',(27.0227913010392,-0.523855189025296,
1.14928485542831));
#18194=CARTESIAN_POINT('Ctrl Pts',(27.0378215228918,-0.739530067688057,
1.01012100713631));
#18195=CARTESIAN_POINT('Ctrl Pts',(27.0422130830678,-0.798426271672689,
0.964216832556656));
#18196=CARTESIAN_POINT('Ctrl Pts',(27.0512360042357,-0.912670203933948,
0.857452222520315));
#18197=CARTESIAN_POINT('Ctrl Pts',(27.05584015108,-0.967015893635766,0.795547574443293));
#18198=CARTESIAN_POINT('Ctrl Pts',(27.0659525686896,-1.07220736914641,0.649253735520837));
#18199=CARTESIAN_POINT('Ctrl Pts',(27.0714835605872,-1.12033323576103,0.562678461508257));
#18200=CARTESIAN_POINT('Ctrl Pts',(27.0819455506405,-1.18817465505177,0.396139701307846));
#18201=CARTESIAN_POINT('Ctrl Pts',(27.0867385530711,-1.21134478405695,0.318194492985015));
#18202=CARTESIAN_POINT('Ctrl Pts',(27.0962163230492,-1.2424108923148,0.15708382713042));
#18203=CARTESIAN_POINT('Ctrl Pts',(27.1008945859079,-1.24996681522301,0.0743209691452767));
#18204=CARTESIAN_POINT('Ctrl Pts',(27.111106975172,-1.24880222921897,-0.106693673917988));
#18205=CARTESIAN_POINT('Ctrl Pts',(27.1166420030754,-1.23673577746144,-0.204964063443941));
#18206=CARTESIAN_POINT('Ctrl Pts',(27.1266813126859,-1.1951055545968,-0.373989150302864));
#18207=CARTESIAN_POINT('Ctrl Pts',(27.1311183617704,-1.17029860772482,-0.445467179592022));
#18208=CARTESIAN_POINT('Ctrl Pts',(27.1447673082394,-1.07278792151908,-0.660273870989051));
#18209=CARTESIAN_POINT('Ctrl Pts',(27.1537912956173,-0.97829819161165,-0.793339356174457));
#18210=CARTESIAN_POINT('Ctrl Pts',(27.1673751717089,-0.806192065988158,
-0.958291527069703));
#18211=CARTESIAN_POINT('Ctrl Pts',(27.1718772242941,-0.744634653422319,
-1.00713043498214));
#18212=CARTESIAN_POINT('Ctrl Pts',(27.185600276084,-0.545160500110301,-1.13577857803707));
#18213=CARTESIAN_POINT('Ctrl Pts',(27.194708148134,-0.394986518730001,-1.19570312093531));
#18214=CARTESIAN_POINT('Ctrl Pts',(27.210896999223,-0.116849507298023,-1.25044185698086));
#18215=CARTESIAN_POINT('Ctrl Pts',(27.2202104785418,0.0506293948963337,
-1.26554583438168));
#18216=CARTESIAN_POINT('Ctrl Pts',(27.2412324844468,0.407852860075084,-1.19180544801608));
#18217=CARTESIAN_POINT('Ctrl Pts',(27.2505976074347,0.559836704426273,-1.12866736293217));
#18218=CARTESIAN_POINT('Ctrl Pts',(27.26421794799,0.759501734458928,-0.995862606038345));
#18219=CARTESIAN_POINT('Ctrl Pts',(27.2685769038316,0.820173225627903,-0.946539669293757));
#18220=CARTESIAN_POINT('Ctrl Pts',(27.2800270563151,0.962634433699707,-0.806046356647483));
#18221=CARTESIAN_POINT('Ctrl Pts',(27.287149432565,1.03664674878547,-0.707833652042005));
#18222=CARTESIAN_POINT('Ctrl Pts',(27.3037659770571,1.17511828860313,-0.456149209535922));
#18223=CARTESIAN_POINT('Ctrl Pts',(27.3127655717947,1.22549966150738,-0.297199147241388));
#18224=CARTESIAN_POINT('Ctrl Pts',(27.3278203043008,1.25270772564518,-0.0368720188271256));
#18225=CARTESIAN_POINT('Ctrl Pts',(27.3334311918074,1.25171066149632,0.0591489682065003));
#18226=CARTESIAN_POINT('Ctrl Pts',(27.3493594591518,1.21813364413176,0.330701470812096));
#18227=CARTESIAN_POINT('Ctrl Pts',(27.3583824392094,1.16064739395832,0.488307261101328));
#18228=CARTESIAN_POINT('Ctrl Pts',(27.3710195528419,1.05054076564694,0.680361565920234));
#18229=CARTESIAN_POINT('Ctrl Pts',(27.3750061791313,1.01172907400335,0.736682885072757));
#18230=CARTESIAN_POINT('Ctrl Pts',(27.3837173999563,0.917762226612901,0.851842029224438));
#18231=CARTESIAN_POINT('Ctrl Pts',(27.3884507068375,0.860813114976424,0.909412367610113));
#18232=CARTESIAN_POINT('Ctrl Pts',(27.3973428772326,0.741055000375852,1.00895802344042));
#18233=CARTESIAN_POINT('Ctrl Pts',(27.4015275583348,0.679029369463859,1.05170053647916));
#18234=CARTESIAN_POINT('Ctrl Pts',(27.4156137715033,0.46012589084204,1.17528367642436));
#18235=CARTESIAN_POINT('Ctrl Pts',(27.4251567813477,0.302460240456135,1.22161543060849));
#18236=CARTESIAN_POINT('Ctrl Pts',(27.4392158463335,0.0621563960705467,
1.25159362700516));
#18237=CARTESIAN_POINT('Ctrl Pts',(27.444496878216,-0.0322708771125176,
1.2525822727184));
#18238=CARTESIAN_POINT('Ctrl Pts',(27.4543480803958,-0.206727963977358,
1.23505225854882));
#18239=CARTESIAN_POINT('Ctrl Pts',(27.4589334593879,-0.287152557177882,
1.21902395681331));
#18240=CARTESIAN_POINT('Ctrl Pts',(27.4682321073975,-0.4416970928263,1.1719697789001));
#18241=CARTESIAN_POINT('Ctrl Pts',(27.4729516116456,-0.515727287380908,
1.14127995022307));
#18242=CARTESIAN_POINT('Ctrl Pts',(27.4843874363185,-0.689129958916375,
1.04895667382227));
#18243=CARTESIAN_POINT('Ctrl Pts',(27.4909756978049,-0.784294679972773,
0.979488370451264));
#18244=CARTESIAN_POINT('Ctrl Pts',(27.5022112586547,-0.927437896374184,
0.841419073632032));
#18245=CARTESIAN_POINT('Ctrl Pts',(27.5068694100356,-0.981136459626848,
0.778485227271648));
#18246=CARTESIAN_POINT('Ctrl Pts',(27.5163578130054,-1.07504666274919,0.643084026884325));
#18247=CARTESIAN_POINT('Ctrl Pts',(27.5211626001225,-1.1148376357819,0.571161446600757));
#18248=CARTESIAN_POINT('Ctrl Pts',(27.5352457956388,-1.21111916930948,0.346914450665397));
#18249=CARTESIAN_POINT('Ctrl Pts',(27.5443859627255,-1.24599797633614,0.185793411298435));
#18250=CARTESIAN_POINT('Ctrl Pts',(27.5653868720338,-1.25396608250648,-0.182192741678661));
#18251=CARTESIAN_POINT('Ctrl Pts',(27.5749869004016,-1.206632677805,-0.344777573954174));
#18252=CARTESIAN_POINT('Ctrl Pts',(27.5863792440645,-1.13455557543746,-0.529557994741678));
#18253=CARTESIAN_POINT('Ctrl Pts',(27.5911157086978,-1.09700019906553,-0.603652685816796));
#18254=CARTESIAN_POINT('Ctrl Pts',(27.6052193646264,-0.96440654221833,-0.81188213774616));
#18255=CARTESIAN_POINT('Ctrl Pts',(27.614292162518,-0.851307653605388,-0.929748658073967));
#18256=CARTESIAN_POINT('Ctrl Pts',(27.6310557749972,-0.613091677158633,
-1.09581581684141));
#18257=CARTESIAN_POINT('Ctrl Pts',(27.638388107942,-0.498563383005862,-1.15256212981081));
#18258=CARTESIAN_POINT('Ctrl Pts',(27.6529532597672,-0.255556338240585,
-1.23032546824917));
#18259=CARTESIAN_POINT('Ctrl Pts',(27.6600166118184,-0.128743288277099,
-1.24994404136352));
#18260=CARTESIAN_POINT('Ctrl Pts',(27.6674547598791,1.13833429835281E-5,
-1.24969819048317));
#18261=CARTESIAN_POINT('Ctrl Pts',(27.85693036647,0.3508711481781,-0.9020783645694));
#18262=CARTESIAN_POINT('Ctrl Pts',(27.84253965393,0.1696145104598,-0.9725796947077));
#18263=CARTESIAN_POINT('Ctrl Pts',(27.81375822884,-0.2362176485044,-1.000787437649));
#18264=CARTESIAN_POINT('Ctrl Pts',(27.7705860912,-0.7620645579118,-0.6904694580177));
#18265=CARTESIAN_POINT('Ctrl Pts',(27.72741395357,-1.019191121247,-0.136727519574));
#18266=CARTESIAN_POINT('Ctrl Pts',(27.68424181593,-0.9170855048544,0.4651998272662));
#18267=CARTESIAN_POINT('Ctrl Pts',(27.6410696783,-0.491706155922,0.9031499546372));
#18268=CARTESIAN_POINT('Ctrl Pts',(27.59789754066,0.1069945696502,1.022744811683));
#18269=CARTESIAN_POINT('Ctrl Pts',(27.55472540303,0.6679809012817,0.7818289067868));
#18270=CARTESIAN_POINT('Ctrl Pts',(27.51155326539,0.9935081337884,0.2653232965403));
#18271=CARTESIAN_POINT('Ctrl Pts',(27.46838112776,0.9688301855632,-0.3447070524446));
#18272=CARTESIAN_POINT('Ctrl Pts',(27.42520899013,0.6026458286235,-0.8332303898637));
#18273=CARTESIAN_POINT('Ctrl Pts',(27.38203685249,0.0240327020293,-1.028045381657));
#18274=CARTESIAN_POINT('Ctrl Pts',(27.33886471486,-0.5630517979017,-0.8604809995253));
#18275=CARTESIAN_POINT('Ctrl Pts',(27.29569257722,-0.9516641661597,-0.3896026083503));
#18276=CARTESIAN_POINT('Ctrl Pts',(27.25252043959,-1.004821046675,0.2186081923639));
#18277=CARTESIAN_POINT('Ctrl Pts',(27.20934830195,-0.7037849814483,0.7497610135854));
#18278=CARTESIAN_POINT('Ctrl Pts',(27.16617616432,-0.1546692441643,1.016627907602));
#18279=CARTESIAN_POINT('Ctrl Pts',(27.12300402668,0.4489664052826,0.9251400134749));
#18280=CARTESIAN_POINT('Ctrl Pts',(27.07983188905,0.8943442891871,0.5075462245036));
#18281=CARTESIAN_POINT('Ctrl Pts',(27.03665975141,1.024471572654,-0.08895433890703));
#18282=CARTESIAN_POINT('Ctrl Pts',(26.99348761378,0.7934792266292,-0.6540990709153));
#18283=CARTESIAN_POINT('Ctrl Pts',(26.95031547614,0.282790564744,-0.9886780942271));
#18284=CARTESIAN_POINT('Ctrl Pts',(26.90714333851,-0.3275799486865,-0.9747544586039));
#18285=CARTESIAN_POINT('Ctrl Pts',(26.86397120087,-0.8224806433027,-0.6172361556615));
#18286=CARTESIAN_POINT('Ctrl Pts',(26.82079906324,-1.027462199362,-0.04214608490148));
#18287=CARTESIAN_POINT('Ctrl Pts',(26.7776269256,-0.8702699878541,0.5478002119432));
#18288=CARTESIAN_POINT('Ctrl Pts',(26.73445478797,-0.4063130678999,0.9446504531373));
#18289=CARTESIAN_POINT('Ctrl Pts',(26.69128265034,0.200866052972,1.008517532369));
#18290=CARTESIAN_POINT('Ctrl Pts',(26.6481105127,0.7372431919551,0.7168885397455));
#18291=CARTESIAN_POINT('Ctrl Pts',(26.60493837507,1.013739362113,0.172561472936));
#18292=CARTESIAN_POINT('Ctrl Pts',(26.56176623743,0.9329269024502,-0.4325943337183));
#18293=CARTESIAN_POINT('Ctrl Pts',(26.5185940998,0.5231593542597,-0.8852562131224));
#18294=CARTESIAN_POINT('Ctrl Pts',(26.48981267471,0.1273004522624,-0.9790173336412));
#18295=CARTESIAN_POINT('Ctrl Pts',(26.47542196216,-0.06672189150808,-0.9656107536899));
#18296=CARTESIAN_POINT('Ctrl Pts',(27.79531292359,0.3895590831803,-1.001543793165));
#18297=CARTESIAN_POINT('Ctrl Pts',(27.78092221105,0.1883166328491,-1.079818777228));
#18298=CARTESIAN_POINT('Ctrl Pts',(27.75214078596,-0.2622636003565,-1.111136776829));
#18299=CARTESIAN_POINT('Ctrl Pts',(27.70896864832,-0.8460917121451,-0.7666023565235));
#18300=CARTESIAN_POINT('Ctrl Pts',(27.66579651069,-1.131569696854,-0.1518034396597));
#18301=CARTESIAN_POINT('Ctrl Pts',(27.62262437306,-1.018205658471,0.5164939298841));
#18302=CARTESIAN_POINT('Ctrl Pts',(27.57945223542,-0.545922912983,1.002733539448));
#18303=CARTESIAN_POINT('Ctrl Pts',(27.53628009779,0.1187920599189,1.135515226132));
#18304=CARTESIAN_POINT('Ctrl Pts',(27.49310796015,0.7416341549781,0.8680353278211));
#18305=CARTESIAN_POINT('Ctrl Pts',(27.44993582252,1.103054838622,0.2945785103259));
#18306=CARTESIAN_POINT('Ctrl Pts',(27.40676368488,1.075655837777,-0.3827153187527));
#18307=CARTESIAN_POINT('Ctrl Pts',(27.36359154725,0.669095072935,-0.9251044676621));
#18308=CARTESIAN_POINT('Ctrl Pts',(27.32041940961,0.02668260818108,-1.141400250279));
#18309=CARTESIAN_POINT('Ctrl Pts',(27.27724727198,-0.6251353048336,-0.9553597980619));
#18310=CARTESIAN_POINT('Ctrl Pts',(27.23407513434,-1.056597049914,-0.4325611715347));
#18311=CARTESIAN_POINT('Ctrl Pts',(27.19090299671,-1.115615141728,0.242712481306));
#18312=CARTESIAN_POINT('Ctrl Pts',(27.14773085907,-0.781386083047,0.8324315480863));
#18313=CARTESIAN_POINT('Ctrl Pts',(27.10455872144,-0.1717234639146,1.128723856827));
#18314=CARTESIAN_POINT('Ctrl Pts',(27.0613865838,0.4984705699766,1.027148277463));
#18315=CARTESIAN_POINT('Ctrl Pts',(27.01821444617,0.9929569391852,0.5635095473536));
#18316=CARTESIAN_POINT('Ctrl Pts',(26.97504230853,1.137432384109,-0.09876266797504));
#18317=CARTESIAN_POINT('Ctrl Pts',(26.9318701709,0.8809702412221,-0.7262216790921));
#18318=CARTESIAN_POINT('Ctrl Pts',(26.88869803327,0.3139717634401,-1.097692226755));
#18319=CARTESIAN_POINT('Ctrl Pts',(26.84552589563,-0.3636997374712,-1.082233336059));
#18320=CARTESIAN_POINT('Ctrl Pts',(26.802353758,-0.913169427017,-0.6852941661171));
#18321=CARTESIAN_POINT('Ctrl Pts',(26.75918162036,-1.140752764838,-0.04679321819168));
#18322=CARTESIAN_POINT('Ctrl Pts',(26.71600948273,-0.9662281448565,0.6082020406598));
#18323=CARTESIAN_POINT('Ctrl Pts',(26.67283734509,-0.4511141683696,1.048809987259));
#18324=CARTESIAN_POINT('Ctrl Pts',(26.62966520746,0.2230140490152,1.119719211229));
#18325=CARTESIAN_POINT('Ctrl Pts',(26.58649306982,0.8185334799691,0.7959344726286));
#18326=CARTESIAN_POINT('Ctrl Pts',(26.54332093219,1.125516813049,0.1915885348176));
#18327=CARTESIAN_POINT('Ctrl Pts',(26.50014879455,1.035793768396,-0.4802932726369));
#18328=CARTESIAN_POINT('Ctrl Pts',(26.45697665692,0.580844220053,-0.9828667890031));
#18329=CARTESIAN_POINT('Ctrl Pts',(26.42819523183,0.1413369202036,-1.086966246416));
#18330=CARTESIAN_POINT('Ctrl Pts',(26.41380451928,-0.07407881502629,-1.072081423251));
#18331=CARTESIAN_POINT('Ctrl Pts',(27.73369548072,0.4282470181825,-1.101009221761));
#18332=CARTESIAN_POINT('Ctrl Pts',(27.71930476817,0.2070187552385,-1.187057859748));
#18333=CARTESIAN_POINT('Ctrl Pts',(27.69052334308,-0.2883095522085,-1.221486116009));
#18334=CARTESIAN_POINT('Ctrl Pts',(27.64735120545,-0.9301188663785,-0.8427352550292));
#18335=CARTESIAN_POINT('Ctrl Pts',(27.60417906781,-1.24394827246,-0.1668793597454));
#18336=CARTESIAN_POINT('Ctrl Pts',(27.56100693018,-1.119325812087,0.5677880325021));
#18337=CARTESIAN_POINT('Ctrl Pts',(27.51783479254,-0.6001396700441,1.102317124259));
#18338=CARTESIAN_POINT('Ctrl Pts',(27.47466265491,0.1305895501877,1.248285640581));
#18339=CARTESIAN_POINT('Ctrl Pts',(27.43149051727,0.8152874086746,0.9542417488555));
#18340=CARTESIAN_POINT('Ctrl Pts',(27.38831837964,1.212601543456,0.3238337241115));
#18341=CARTESIAN_POINT('Ctrl Pts',(27.345146242,1.182481489992,-0.4207235850609));
#18342=CARTESIAN_POINT('Ctrl Pts',(27.30197410437,0.7355443172465,-1.016978545461));
#18343=CARTESIAN_POINT('Ctrl Pts',(27.25880196673,0.02933251433285,-1.2547551189));
#18344=CARTESIAN_POINT('Ctrl Pts',(27.2156298291,-0.6872188117655,-1.050238596599));
#18345=CARTESIAN_POINT('Ctrl Pts',(27.17245769147,-1.161529933667,-0.475519734719));
#18346=CARTESIAN_POINT('Ctrl Pts',(27.12928555383,-1.226409236781,0.2668167702481));
#18347=CARTESIAN_POINT('Ctrl Pts',(27.0861134162,-0.8589871846457,0.9151020825871));
#18348=CARTESIAN_POINT('Ctrl Pts',(27.04294127856,-0.1887776836649,1.240819806052));
#18349=CARTESIAN_POINT('Ctrl Pts',(26.99976914093,0.5479747346705,1.129156541452));
#18350=CARTESIAN_POINT('Ctrl Pts',(26.95659700329,1.091569589183,0.6194728702036));
#18351=CARTESIAN_POINT('Ctrl Pts',(26.91342486566,1.250393195564,-0.1085709970431));
#18352=CARTESIAN_POINT('Ctrl Pts',(26.87025272802,0.968461255815,-0.7983442872689));
#18353=CARTESIAN_POINT('Ctrl Pts',(26.82708059039,0.3451529621362,-1.206706359282));
#18354=CARTESIAN_POINT('Ctrl Pts',(26.78390845275,-0.3998195262558,-1.189712213514));
#18355=CARTESIAN_POINT('Ctrl Pts',(26.74073631512,-1.003858210731,-0.7533521765727));
#18356=CARTESIAN_POINT('Ctrl Pts',(26.69756417748,-1.254043330314,-0.05144035148188));
#18357=CARTESIAN_POINT('Ctrl Pts',(26.65439203985,-1.062186301859,0.6686038693765));
#18358=CARTESIAN_POINT('Ctrl Pts',(26.61121990221,-0.4959152688394,1.15296952138));
#18359=CARTESIAN_POINT('Ctrl Pts',(26.56804776458,0.2451620450585,1.230920890089));
#18360=CARTESIAN_POINT('Ctrl Pts',(26.52487562694,0.8998237679831,0.8749804055118));
#18361=CARTESIAN_POINT('Ctrl Pts',(26.48170348931,1.237294263986,0.2106155966992));
#18362=CARTESIAN_POINT('Ctrl Pts',(26.43853135168,1.138660634342,-0.5279922115554));
#18363=CARTESIAN_POINT('Ctrl Pts',(26.39535921404,0.6385290858464,-1.080477364884));
#18364=CARTESIAN_POINT('Ctrl Pts',(26.36657778895,0.1553733881448,-1.194915159191));
#18365=CARTESIAN_POINT('Ctrl Pts',(26.35218707641,-0.08143573854449,-1.178552092812));
#18366=CARTESIAN_POINT('Ctrl Pts',(27.67207803784,0.4669349531848,-1.200474650356));
#18367=CARTESIAN_POINT('Ctrl Pts',(27.65768732529,0.2257208776278,-1.294296942268));
#18368=CARTESIAN_POINT('Ctrl Pts',(27.6289059002,-0.3143555040606,-1.33183545519));
#18369=CARTESIAN_POINT('Ctrl Pts',(27.58573376257,-1.014146020612,-0.9188681535349));
#18370=CARTESIAN_POINT('Ctrl Pts',(27.54256162493,-1.356326848067,-0.181955279831));
#18371=CARTESIAN_POINT('Ctrl Pts',(27.4993894873,-1.220445965703,0.6190821351201));
#18372=CARTESIAN_POINT('Ctrl Pts',(27.45621734966,-0.6543564271052,1.20190070907));
#18373=CARTESIAN_POINT('Ctrl Pts',(27.41304521203,0.1423870404564,1.36105605503));
#18374=CARTESIAN_POINT('Ctrl Pts',(27.3698730744,0.888940662371,1.04044816989));
#18375=CARTESIAN_POINT('Ctrl Pts',(27.32670093676,1.32214824829,0.353088937897));
#18376=CARTESIAN_POINT('Ctrl Pts',(27.28352879913,1.289307142206,-0.458731851369));
#18377=CARTESIAN_POINT('Ctrl Pts',(27.24035666149,0.8019935615581,-1.108852623259));
#18378=CARTESIAN_POINT('Ctrl Pts',(27.19718452386,0.03198242048463,-1.368109987522));
#18379=CARTESIAN_POINT('Ctrl Pts',(27.15401238622,-0.7493023186974,-1.145117395135));
#18380=CARTESIAN_POINT('Ctrl Pts',(27.11084024859,-1.266462817421,-0.5184782979033));
#18381=CARTESIAN_POINT('Ctrl Pts',(27.06766811095,-1.337203331834,0.2909210591902));
#18382=CARTESIAN_POINT('Ctrl Pts',(27.02449597332,-0.9365882862444,0.997772617088));
#18383=CARTESIAN_POINT('Ctrl Pts',(26.98132383568,-0.2058319034152,1.352915755277));
#18384=CARTESIAN_POINT('Ctrl Pts',(26.93815169805,0.5974788993645,1.23116480544));
#18385=CARTESIAN_POINT('Ctrl Pts',(26.89497956041,1.190182239181,0.6754361930536));
#18386=CARTESIAN_POINT('Ctrl Pts',(26.85180742278,1.36335400702,-0.1183793261111));
#18387=CARTESIAN_POINT('Ctrl Pts',(26.80863528514,1.055952270408,-0.8704668954457));
#18388=CARTESIAN_POINT('Ctrl Pts',(26.76546314751,0.3763341608323,-1.31572049181));
#18389=CARTESIAN_POINT('Ctrl Pts',(26.72229100988,-0.4359393150405,-1.29719109097));
#18390=CARTESIAN_POINT('Ctrl Pts',(26.67911887224,-1.094546994446,-0.8214101870282));
#18391=CARTESIAN_POINT('Ctrl Pts',(26.63594673461,-1.367333895789,-0.05608748477207));
#18392=CARTESIAN_POINT('Ctrl Pts',(26.59277459697,-1.158144458861,0.7290056980931));
#18393=CARTESIAN_POINT('Ctrl Pts',(26.54960245934,-0.5407163693092,1.257129055501));
#18394=CARTESIAN_POINT('Ctrl Pts',(26.5064303217,0.2673100411017,1.342122568949));
#18395=CARTESIAN_POINT('Ctrl Pts',(26.46325818407,0.9811140559971,0.954026338395));
#18396=CARTESIAN_POINT('Ctrl Pts',(26.42008604643,1.349071714923,0.2296426585807));
#18397=CARTESIAN_POINT('Ctrl Pts',(26.3769139088,1.241527500287,-0.575691150474));
#18398=CARTESIAN_POINT('Ctrl Pts',(26.33374177116,0.6962139516397,-1.178087940765));
#18399=CARTESIAN_POINT('Ctrl Pts',(26.30496034607,0.1694098560859,-1.302864071967));
#18400=CARTESIAN_POINT('Ctrl Pts',(26.29056963353,-0.08879266206269,-1.285022762373));
#18401=CARTESIAN_POINT('',(26.4799750801814,0.957494124951751,0.803490379093413));
#18402=CARTESIAN_POINT('',(26.48,0.30130639050121,-0.959765445450973));
#18403=CARTESIAN_POINT('Ctrl Pts',(26.48,0.957461769231118,0.803461599229706));
#18404=CARTESIAN_POINT('Ctrl Pts',(26.48,1.02085303890837,0.710326903088572));
#18405=CARTESIAN_POINT('Ctrl Pts',(26.4800000000004,1.07146792946953,0.608458766671006));
#18406=CARTESIAN_POINT('Ctrl Pts',(26.4800000000004,1.14222700822191,0.398129979097469));
#18407=CARTESIAN_POINT('Ctrl Pts',(26.48,1.16333891588263,0.289629207331002));
#18408=CARTESIAN_POINT('Ctrl Pts',(26.48,1.17576370208854,0.0291771618104245));
#18409=CARTESIAN_POINT('Ctrl Pts',(26.4799999998511,1.15317936540575,-0.122946830566836));
#18410=CARTESIAN_POINT('Ctrl Pts',(26.4799999998511,1.05339965425113,-0.402142814256775));
#18411=CARTESIAN_POINT('Ctrl Pts',(26.48,0.979092823411478,-0.526892044615511));
#18412=CARTESIAN_POINT('Ctrl Pts',(26.48,0.80319537267829,-0.719709080817574));
#18413=CARTESIAN_POINT('Ctrl Pts',(26.48,0.711886836330681,-0.792651002690939));
#18414=CARTESIAN_POINT('Ctrl Pts',(26.48,0.488721612126881,-0.916845005852681));
#18415=CARTESIAN_POINT('Ctrl Pts',(26.48,0.378913387594024,-0.945604681625937));
#18416=CARTESIAN_POINT('Ctrl Pts',(26.48,0.30130639050121,-0.959765445450973));
#18417=CARTESIAN_POINT('Ctrl Pts',(27.8084936838606,-7.83629518364392E-6,
-1.00548644875247));
#18418=CARTESIAN_POINT('Ctrl Pts',(27.8009336227228,-0.105754067060467,
-1.00565130875726));
#18419=CARTESIAN_POINT('Ctrl Pts',(27.7920355843156,-0.229774370990478,
-0.989890792203826));
#18420=CARTESIAN_POINT('Ctrl Pts',(27.773278015885,-0.47684507127086,-0.893688393002027));
#18421=CARTESIAN_POINT('Ctrl Pts',(27.7647110839715,-0.58323674538791,-0.827893655969334));
#18422=CARTESIAN_POINT('Ctrl Pts',(27.7494978495145,-0.741104731770526,
-0.685814064305951));
#18423=CARTESIAN_POINT('Ctrl Pts',(27.7433408520941,-0.794958590434357,
-0.621862691176406));
#18424=CARTESIAN_POINT('Ctrl Pts',(27.7328730435246,-0.875623640068458,
-0.499430636746069));
#18425=CARTESIAN_POINT('Ctrl Pts',(27.7282665986025,-0.906439891086461,
-0.440457560251828));
#18426=CARTESIAN_POINT('Ctrl Pts',(27.7174007537854,-0.964992524600893,
-0.295815934039164));
#18427=CARTESIAN_POINT('Ctrl Pts',(27.7111175803318,-0.987750306056034,
-0.208040340531976));
#18428=CARTESIAN_POINT('Ctrl Pts',(27.6986095379843,-1.00844004152666,-0.0382152991818625));
#18429=CARTESIAN_POINT('Ctrl Pts',(27.6925773617797,-1.00849881112007,0.0433778302428258));
#18430=CARTESIAN_POINT('Ctrl Pts',(27.6808363100849,-0.987396042424842,
0.209104271202132));
#18431=CARTESIAN_POINT('Ctrl Pts',(27.6750717349432,-0.965801035552071,
0.291998972276148));
#18432=CARTESIAN_POINT('Ctrl Pts',(27.6627065622329,-0.900686289080503,
0.455917110370338));
#18433=CARTESIAN_POINT('Ctrl Pts',(27.6558888426671,-0.855591925828399,
0.536406732927371));
#18434=CARTESIAN_POINT('Ctrl Pts',(27.6426720250847,-0.746938893915059,
0.679824479257801));
#18435=CARTESIAN_POINT('Ctrl Pts',(27.6363904762984,-0.682615856064763,
0.745256780425583));
#18436=CARTESIAN_POINT('Ctrl Pts',(27.6261346961145,-0.562949307185261,
0.834625638450677));
#18437=CARTESIAN_POINT('Ctrl Pts',(27.6226177132574,-0.519867531455672,
0.862024926125074));
#18438=CARTESIAN_POINT('Ctrl Pts',(27.6131419042199,-0.403160023299481,
0.924626544942976));
#18439=CARTESIAN_POINT('Ctrl Pts',(27.6070066010663,-0.326679169221438,
0.954639953302017));
#18440=CARTESIAN_POINT('Ctrl Pts',(27.597120056192,-0.19552463113609,0.988296274420178));
#18441=CARTESIAN_POINT('Ctrl Pts',(27.5933330803712,-0.14272693439211,0.99730913976307));
#18442=CARTESIAN_POINT('Ctrl Pts',(27.5829898392745,0.00664271603791499,
1.01023975061682));
#18443=CARTESIAN_POINT('Ctrl Pts',(27.5764661542004,0.103460129787075,1.0045930441376));
#18444=CARTESIAN_POINT('Ctrl Pts',(27.563773697374,0.274950320035545,0.970307099663595));
#18445=CARTESIAN_POINT('Ctrl Pts',(27.5578955858851,0.350585845332744,0.945917150096465));
#18446=CARTESIAN_POINT('Ctrl Pts',(27.5461449513803,0.498391225782096,0.87796896122679));
#18447=CARTESIAN_POINT('Ctrl Pts',(27.540531079811,0.56887184427116,0.833722867995117));
#18448=CARTESIAN_POINT('Ctrl Pts',(27.5262887031483,0.728308631585911,0.703771282776339));
#18449=CARTESIAN_POINT('Ctrl Pts',(27.5172053338825,0.809402654229873,0.608834343437791));
#18450=CARTESIAN_POINT('Ctrl Pts',(27.4964498235742,0.953372208461222,0.361035812979152));
#18451=CARTESIAN_POINT('Ctrl Pts',(27.4875406304835,0.983506134098712,0.229915481838277));
#18452=CARTESIAN_POINT('Ctrl Pts',(27.4718461172469,1.01312158666829,0.0114826670106345));
#18453=CARTESIAN_POINT('Ctrl Pts',(27.4625850017575,1.00681094283761,-0.117481830530138));
#18454=CARTESIAN_POINT('Ctrl Pts',(27.448890878927,0.961220081906566,-0.30412355893231));
#18455=CARTESIAN_POINT('Ctrl Pts',(27.4443571105972,0.939479882086676,-0.365378803348319));
#18456=CARTESIAN_POINT('Ctrl Pts',(27.4305000744923,0.856277477027791,-0.542967381960826));
#18457=CARTESIAN_POINT('Ctrl Pts',(27.4211503950537,0.777214337805915,-0.651022403982935));
#18458=CARTESIAN_POINT('Ctrl Pts',(27.4072442145789,0.634940248517312,-0.782652594761028));
#18459=CARTESIAN_POINT('Ctrl Pts',(27.4027040017641,0.584921314853706,-0.820976495091213));
#18460=CARTESIAN_POINT('Ctrl Pts',(27.3888085142676,0.419653710460084,-0.923480810164823));
#18461=CARTESIAN_POINT('Ctrl Pts',(27.3797021246236,0.29411315679714,-0.970164097544654));
#18462=CARTESIAN_POINT('Ctrl Pts',(27.3636473871652,0.071521787740989,-1.00750002449848));
#18463=CARTESIAN_POINT('Ctrl Pts',(27.3537095866507,-0.0642830173812026,
-1.017760320162));
#18464=CARTESIAN_POINT('Ctrl Pts',(27.3328121873029,-0.354868943366727,
-0.949954651919668));
#18465=CARTESIAN_POINT('Ctrl Pts',(27.3237113341857,-0.478148457487225,
-0.894231261672206));
#18466=CARTESIAN_POINT('Ctrl Pts',(27.3100724995674,-0.629200057466457,
-0.786558893392617));
#18467=CARTESIAN_POINT('Ctrl Pts',(27.3061262548567,-0.669982979999203,
-0.752350761317609));
#18468=CARTESIAN_POINT('Ctrl Pts',(27.2975937907535,-0.754422366048413,
-0.668679633211809));
#18469=CARTESIAN_POINT('Ctrl Pts',(27.2930682902501,-0.796349974820793,
-0.617739935544105));
#18470=CARTESIAN_POINT('Ctrl Pts',(27.2828415758626,-0.879122103649902,
-0.494677808294302));
#18471=CARTESIAN_POINT('Ctrl Pts',(27.27710540015,-0.916911696347268,-0.420457326220017));
#18472=CARTESIAN_POINT('Ctrl Pts',(27.2642008684414,-0.977418418500146,
-0.254773622903383));
#18473=CARTESIAN_POINT('Ctrl Pts',(27.2545397745644,-1.01089657642268,-0.127082208364601));
#18474=CARTESIAN_POINT('Ctrl Pts',(27.2379084037118,-1.002202109097,0.115191605784107));
#18475=CARTESIAN_POINT('Ctrl Pts',(27.2322586174677,-0.989262746073459,
0.196801934931889));
#18476=CARTESIAN_POINT('Ctrl Pts',(27.2183588117237,-0.937186932251371,
0.380334639660224));
#18477=CARTESIAN_POINT('Ctrl Pts',(27.2086823458243,-0.885524725166168,
0.500766071236578));
#18478=CARTESIAN_POINT('Ctrl Pts',(27.1934790672189,-0.748776202161178,
0.675135895490028));
#18479=CARTESIAN_POINT('Ctrl Pts',(27.1885710133545,-0.698348939271822,
0.726855320763439));
#18480=CARTESIAN_POINT('Ctrl Pts',(27.1787772818171,-0.593528840519058,
0.814013154258869));
#18481=CARTESIAN_POINT('Ctrl Pts',(27.174009726289,-0.540026394969414,0.850601928307751));
#18482=CARTESIAN_POINT('Ctrl Pts',(27.1650329138941,-0.432715409844361,
0.90983782809936));
#18483=CARTESIAN_POINT('Ctrl Pts',(27.1608107122522,-0.379380989376285,
0.93355737677979));
#18484=CARTESIAN_POINT('Ctrl Pts',(27.1525700659823,-0.26797998648047,0.971452041509777));
#18485=CARTESIAN_POINT('Ctrl Pts',(27.1485518003818,-0.209998949928167,
0.985397384558026));
#18486=CARTESIAN_POINT('Ctrl Pts',(27.1397847329914,-0.0856608380001726,
1.00397337165135));
#18487=CARTESIAN_POINT('Ctrl Pts',(27.1350049237552,-0.0191006219463654,
1.00733745497235));
#18488=CARTESIAN_POINT('Ctrl Pts',(27.1253893832093,0.113181376821662,1.00125048035375));
#18489=CARTESIAN_POINT('Ctrl Pts',(27.120551622183,0.17897468945219,0.991827642205074));
#18490=CARTESIAN_POINT('Ctrl Pts',(27.105694488606,0.379768703194086,0.942345165306981));
#18491=CARTESIAN_POINT('Ctrl Pts',(27.0979105674963,0.482056046731077,0.886609333801805));
#18492=CARTESIAN_POINT('Ctrl Pts',(27.0825651562094,0.661963323035827,0.767793898264308));
#18493=CARTESIAN_POINT('Ctrl Pts',(27.0729859011291,0.757757849185879,0.674195878184252));
#18494=CARTESIAN_POINT('Ctrl Pts',(27.054263232748,0.905973775380077,0.457076143509283));
#18495=CARTESIAN_POINT('Ctrl Pts',(27.0455407361517,0.954259556577819,0.339816288159658));
#18496=CARTESIAN_POINT('Ctrl Pts',(27.0320144835362,0.9957262694812,0.154100298030815));
#18497=CARTESIAN_POINT('Ctrl Pts',(27.0272397936893,1.003935703847,0.0873954592435777));
#18498=CARTESIAN_POINT('Ctrl Pts',(27.0177717823106,1.00700302449346,-0.0444843111274326));
#18499=CARTESIAN_POINT('Ctrl Pts',(27.013044895658,1.00221469752981,-0.109729607703128));
#18500=CARTESIAN_POINT('Ctrl Pts',(26.9993758608286,0.968747071973493,-0.298252835788282));
#18501=CARTESIAN_POINT('Ctrl Pts',(26.9906629320194,0.922879088675033,-0.417883691589809));
#18502=CARTESIAN_POINT('Ctrl Pts',(26.9723583139129,0.788667222308375,-0.637735077391912));
#18503=CARTESIAN_POINT('Ctrl Pts',(26.9628426827107,0.701272403080465,-0.733523066314639));
#18504=CARTESIAN_POINT('Ctrl Pts',(26.945029819685,0.495705288711316,-0.883192578930708));
#18505=CARTESIAN_POINT('Ctrl Pts',(26.9367073299812,0.38396161494691,-0.937028583468894));
#18506=CARTESIAN_POINT('Ctrl Pts',(26.9234973859547,0.209548310468475,-0.985462237804072));
#18507=CARTESIAN_POINT('Ctrl Pts',(26.9190729775717,0.151198444492355,-0.996299134478789));
#18508=CARTESIAN_POINT('Ctrl Pts',(26.9107316961501,0.0364449296399151,
-1.00692734940693));
#18509=CARTESIAN_POINT('Ctrl Pts',(26.9068314082864,-0.0197150318892842,
-1.00720593274486));
#18510=CARTESIAN_POINT('Ctrl Pts',(26.8991961895396,-0.129935669177869,
-0.998606009375022));
#18511=CARTESIAN_POINT('Ctrl Pts',(26.8954498587092,-0.184115446692132,
-0.989914924496511));
#18512=CARTESIAN_POINT('Ctrl Pts',(26.8886420806066,-0.27860726670274,-0.966923747560494));
#18513=CARTESIAN_POINT('Ctrl Pts',(26.8856029715941,-0.319348681791324,
-0.954288572120448));
#18514=CARTESIAN_POINT('Ctrl Pts',(26.876278734407,-0.438581322083352,-0.908979279685783));
#18515=CARTESIAN_POINT('Ctrl Pts',(26.8677039954806,-0.542210751803785,
-0.858841061577955));
#18516=CARTESIAN_POINT('Ctrl Pts',(26.8540971674004,-0.692723890886937,
-0.731436714620663));
#18517=CARTESIAN_POINT('Ctrl Pts',(26.8501107762574,-0.734215447107898,
-0.689496080237736));
#18518=CARTESIAN_POINT('Ctrl Pts',(26.8411141794617,-0.816719544410732,
-0.590401558842806));
#18519=CARTESIAN_POINT('Ctrl Pts',(26.8359760088228,-0.856097745748887,
-0.531847235370042));
#18520=CARTESIAN_POINT('Ctrl Pts',(26.8242232810824,-0.930905847823687,
-0.391197353485646));
#18521=CARTESIAN_POINT('Ctrl Pts',(26.8182257784963,-0.959237421582567,
-0.313552337099464));
#18522=CARTESIAN_POINT('Ctrl Pts',(26.8084899505984,-0.9920819207877,-0.176839070096071));
#18523=CARTESIAN_POINT('Ctrl Pts',(26.8043316223949,-1.00083739890212,-0.115589566840668));
#18524=CARTESIAN_POINT('Ctrl Pts',(26.7958733475466,-1.00710165815903,0.00524138072349242));
#18525=CARTESIAN_POINT('Ctrl Pts',(26.791562957255,-1.0050070914625,0.0648276033447589));
#18526=CARTESIAN_POINT('Ctrl Pts',(26.7824246016789,-0.989835609104069,
0.188767362050434));
#18527=CARTESIAN_POINT('Ctrl Pts',(26.7775899504897,-0.975637924444642,
0.253039895424551));
#18528=CARTESIAN_POINT('Ctrl Pts',(26.7675145592988,-0.931932833192986,
0.386377020525932));
#18529=CARTESIAN_POINT('Ctrl Pts',(26.7624848873892,-0.900738489313069,
0.453879427471441));
#18530=CARTESIAN_POINT('Ctrl Pts',(26.7508247859445,-0.813764531387686,
0.597951517757357));
#18531=CARTESIAN_POINT('Ctrl Pts',(26.7439861045199,-0.753768829314911,
0.671792661606329));
#18532=CARTESIAN_POINT('Ctrl Pts',(26.732313158003,-0.63642527740879,0.781414580552255));
#18533=CARTESIAN_POINT('Ctrl Pts',(26.7274836783147,-0.583436919963472,
0.822051017128429));
#18534=CARTESIAN_POINT('Ctrl Pts',(26.7180391551223,-0.47022637164988,0.891900283266709));
#18535=CARTESIAN_POINT('Ctrl Pts',(26.7135120120417,-0.410507019943939,
0.920676426924196));
#18536=CARTESIAN_POINT('Ctrl Pts',(26.6996488614091,-0.225546255409973,
0.988430098645153));
#18537=CARTESIAN_POINT('Ctrl Pts',(26.6901311955291,-0.0935309357609265,
1.00955494059032));
#18538=CARTESIAN_POINT('Ctrl Pts',(26.6688743049094,0.202509412642327,0.999369048917218));
#18539=CARTESIAN_POINT('Ctrl Pts',(26.6595920452875,0.330583752256524,0.954406597362309));
#18540=CARTESIAN_POINT('Ctrl Pts',(26.6481896460982,0.477002107226659,0.88747520526504));
#18541=CARTESIAN_POINT('Ctrl Pts',(26.6434549358668,0.534926394103887,0.85384167615128));
#18542=CARTESIAN_POINT('Ctrl Pts',(26.6317093514896,0.668341736471132,0.757855225867808));
#18543=CARTESIAN_POINT('Ctrl Pts',(26.622097262116,0.769455365185776,0.669034510295732));
#18544=CARTESIAN_POINT('Ctrl Pts',(26.6014636705348,0.9227959351281,0.418879376339033));
#18545=CARTESIAN_POINT('Ctrl Pts',(26.5925615294449,0.969028638283612,0.296941886440832));
#18546=CARTESIAN_POINT('Ctrl Pts',(26.5797404230048,0.999437393194108,0.123541511218597));
#18547=CARTESIAN_POINT('Ctrl Pts',(26.5761718406925,1.00435207811376,0.0754448842792575));
#18548=CARTESIAN_POINT('Ctrl Pts',(26.5679515523816,1.00737329060242,-0.038667420070806));
#18549=CARTESIAN_POINT('Ctrl Pts',(26.5633693507695,1.0024200700062,-0.104585601058802));
#18550=CARTESIAN_POINT('Ctrl Pts',(26.5542249799062,0.979913496597944,-0.234360841833059));
#18551=CARTESIAN_POINT('Ctrl Pts',(26.549658364145,0.962336259399457,-0.298233941414874));
#18552=CARTESIAN_POINT('Ctrl Pts',(26.5393351018499,0.910634045058272,-0.43369640109639));
#18553=CARTESIAN_POINT('Ctrl Pts',(26.5334081765392,0.873884718327807,-0.504322181721031));
#18554=CARTESIAN_POINT('Ctrl Pts',(26.5222539995358,0.787577860226268,-0.630341976828754));
#18555=CARTESIAN_POINT('Ctrl Pts',(26.5171776069107,0.739341679098445,-0.685834840722942));
#18556=CARTESIAN_POINT('Ctrl Pts',(26.5071323384881,0.632397905463546,-0.78503152398032));
#18557=CARTESIAN_POINT('Ctrl Pts',(26.5021274264087,0.573559983600013,-0.828865420537326));
#18558=CARTESIAN_POINT('Ctrl Pts',(26.4913633348382,0.444814130765567,-0.905021459156498));
#18559=CARTESIAN_POINT('Ctrl Pts',(26.4855829862639,0.37441792388143,-0.936673453025792));
#18560=CARTESIAN_POINT('Ctrl Pts',(26.48,0.301306390501208,-0.959765445450967));
#18561=CARTESIAN_POINT('Ctrl Pts',(26.6174876988274,-1.08253756335566,0.624989939058213));
#18562=CARTESIAN_POINT('Ctrl Pts',(26.6118401171573,-1.03277812122718,0.711177670842943));
#18563=CARTESIAN_POINT('Ctrl Pts',(26.6059838000754,-0.972907071838,0.791109058417356));
#18564=CARTESIAN_POINT('Ctrl Pts',(26.5945079327168,-0.836620351594296,
0.93388751221825));
#18565=CARTESIAN_POINT('Ctrl Pts',(26.5889475836508,-0.760956332926198,
0.996507324316406));
#18566=CARTESIAN_POINT('Ctrl Pts',(26.579230377562,-0.615904061961894,1.09030505776182));
#18567=CARTESIAN_POINT('Ctrl Pts',(26.5750586406361,-0.549527520478794,
1.12522083031085));
#18568=CARTESIAN_POINT('Ctrl Pts',(26.5633658017298,-0.361940074516377,
1.2033170497122));
#18569=CARTESIAN_POINT('Ctrl Pts',(26.5557938111644,-0.236556154100087,
1.23410603940934));
#18570=CARTESIAN_POINT('Ctrl Pts',(26.54125785368,0.0171101028460626,1.25624490060463));
#18571=CARTESIAN_POINT('Ctrl Pts',(26.5343477764224,0.143836069469094,1.24810014955365));
#18572=CARTESIAN_POINT('Ctrl Pts',(26.5224569159616,0.345301590116501,1.20401890236638));
#18573=CARTESIAN_POINT('Ctrl Pts',(26.5177537241328,0.42159976540536,1.17946955919645));
#18574=CARTESIAN_POINT('Ctrl Pts',(26.5074861461494,0.583961520950492,1.10944536839998));
#18575=CARTESIAN_POINT('Ctrl Pts',(26.5019955497172,0.668138478073375,1.06088303115606));
#18576=CARTESIAN_POINT('Ctrl Pts',(26.4910936682112,0.823720462037962,0.945196959309205));
#18577=CARTESIAN_POINT('Ctrl Pts',(26.4856504306765,0.894565028502785,0.878444420944619));
#18578=CARTESIAN_POINT('Ctrl Pts',(26.48,0.956976228538287,0.80417442014319));
#18579=CARTESIAN_POINT('Origin',(26.48,0.,0.));
#18580=CARTESIAN_POINT('',(26.48,-1.082531754731,0.625));
#18581=CARTESIAN_POINT('',(26.48,-1.082531754731,0.625));
#18582=CARTESIAN_POINT('',(26.4799263573241,0.299169738002039,-0.960296952971633));
#18583=CARTESIAN_POINT('Ctrl Pts',(26.48,0.299165873930179,-0.960438829681521));
#18584=CARTESIAN_POINT('Ctrl Pts',(26.48,0.28312281539582,-0.965465660736469));
#18585=CARTESIAN_POINT('Ctrl Pts',(26.48,0.266819075223698,-0.970122449195917));
#18586=CARTESIAN_POINT('Ctrl Pts',(26.48,0.250214467165749,-0.974386330169429));
#18587=CARTESIAN_POINT('Ctrl Pts',(26.48,0.22635906714301,-0.980512134880837));
#18588=CARTESIAN_POINT('Ctrl Pts',(26.48,0.201882178115972,-0.985828929023409));
#18589=CARTESIAN_POINT('Ctrl Pts',(26.48,0.176676262857162,-0.990268554781819));
#18590=CARTESIAN_POINT('Ctrl Pts',(26.48,0.159925265242825,-0.993218979700894));
#18591=CARTESIAN_POINT('Ctrl Pts',(26.48,0.142852303253251,-0.995781004584336));
#18592=CARTESIAN_POINT('Ctrl Pts',(26.48,0.1254280189412,-0.997921901144576));
#18593=CARTESIAN_POINT('Ctrl Pts',(26.48,0.106806947823086,-1.00020984516516));
#18594=CARTESIAN_POINT('Ctrl Pts',(26.48,0.087776514520671,-1.0020162271941));
#18595=CARTESIAN_POINT('Ctrl Pts',(26.48,0.0683974909113733,-1.00328531223436));
#18596=CARTESIAN_POINT('Ctrl Pts',(26.48,0.0391293928497931,-1.00520200866632));
#18597=CARTESIAN_POINT('Ctrl Pts',(26.48,0.00906666890656565,-1.00589086154893));
#18598=CARTESIAN_POINT('Ctrl Pts',(26.48,-0.0215437351157509,-1.00519168337061));
#18599=CARTESIAN_POINT('Ctrl Pts',(26.48,-0.0481886343063174,-1.00458308205768));
#18600=CARTESIAN_POINT('Ctrl Pts',(26.48,-0.0752448170259378,-1.00292363113161));
#18601=CARTESIAN_POINT('Ctrl Pts',(26.48,-0.102542009190776,-1.00013317947925));
#18602=CARTESIAN_POINT('Ctrl Pts',(26.48,-0.131219127055196,-0.997201665115199));
#18603=CARTESIAN_POINT('Ctrl Pts',(26.48,-0.160161370119554,-0.993019741605458));
#18604=CARTESIAN_POINT('Ctrl Pts',(26.48,-0.189092775340995,-0.987540095371076));
#18605=CARTESIAN_POINT('Ctrl Pts',(26.48,-0.217536691483223,-0.98215278021003));
#18606=CARTESIAN_POINT('Ctrl Pts',(26.48,-0.245969377079973,-0.975511179037565));
#18607=CARTESIAN_POINT('Ctrl Pts',(26.48,-0.274127555915594,-0.967619521056985));
#18608=CARTESIAN_POINT('Ctrl Pts',(26.48,-0.290036541633927,-0.963160842289444));
#18609=CARTESIAN_POINT('Ctrl Pts',(26.48,-0.305854987209035,-0.958305057016084));
#18610=CARTESIAN_POINT('Ctrl Pts',(26.48,-0.321547816938486,-0.953056006990891));
#18611=CARTESIAN_POINT('Ctrl Pts',(26.48,-0.354061646781041,-0.94218054843456));
#18612=CARTESIAN_POINT('Ctrl Pts',(26.48,-0.386053020747235,-0.929613078171765));
#18613=CARTESIAN_POINT('Ctrl Pts',(26.48,-0.417347274845933,-0.91534542779146));
#18614=CARTESIAN_POINT('Ctrl Pts',(26.48,-0.443935398451674,-0.903223392523304));
#18615=CARTESIAN_POINT('Ctrl Pts',(26.48,-0.470020191345163,-0.889873838305286));
#18616=CARTESIAN_POINT('Ctrl Pts',(26.48,-0.495521901499934,-0.875357685473186));
#18617=CARTESIAN_POINT('Ctrl Pts',(26.48,-0.513450745658883,-0.865152180025328));
#18618=CARTESIAN_POINT('Ctrl Pts',(26.48,-0.531097296304518,-0.854365555490116));
#18619=CARTESIAN_POINT('Ctrl Pts',(26.48,-0.548395974066936,-0.843044270906004));
#18620=CARTESIAN_POINT('Ctrl Pts',(26.48,-0.57349785717507,-0.826616104189026));
#18621=CARTESIAN_POINT('Ctrl Pts',(26.48,-0.597861150258046,-0.809063033772212));
#18622=CARTESIAN_POINT('Ctrl Pts',(26.48,-0.621289762137012,-0.790576020950967));
#18623=CARTESIAN_POINT('Ctrl Pts',(26.48,-0.638271052917386,-0.777176450289253));
#18624=CARTESIAN_POINT('Ctrl Pts',(26.48,-0.654761904303153,-0.763287200299691));
#18625=CARTESIAN_POINT('Ctrl Pts',(26.48,-0.670699818177876,-0.748992955275881));
#18626=CARTESIAN_POINT('Ctrl Pts',(26.48,-0.685159587578794,-0.73602441444744));
#18627=CARTESIAN_POINT('Ctrl Pts',(26.48,-0.699159320961954,-0.722728245271615));
#18628=CARTESIAN_POINT('Ctrl Pts',(26.48,-0.712689959359925,-0.709142457287416));
#18629=CARTESIAN_POINT('Ctrl Pts',(26.48,-0.741675752047894,-0.680038521284534));
#18630=CARTESIAN_POINT('Ctrl Pts',(26.48,-0.768514174430042,-0.649603184718264));
#18631=CARTESIAN_POINT('Ctrl Pts',(26.48,-0.793165072752985,-0.61813614173595));
#18632=CARTESIAN_POINT('Ctrl Pts',(26.48,-0.804848277504714,-0.603222449696109));
#18633=CARTESIAN_POINT('Ctrl Pts',(26.48,-0.816040312388025,-0.588076248214693));
#18634=CARTESIAN_POINT('Ctrl Pts',(26.48,-0.826737803251188,-0.572725579677889));
#18635=CARTESIAN_POINT('Ctrl Pts',(26.48,-0.839252376721775,-0.554767436812069));
#18636=CARTESIAN_POINT('Ctrl Pts',(26.48,-0.851086810827611,-0.536538087002317));
#18637=CARTESIAN_POINT('Ctrl Pts',(26.48,-0.862283582369594,-0.517991203487763));
#18638=CARTESIAN_POINT('Ctrl Pts',(26.48,-0.875652514133851,-0.495846246862011));
#18639=CARTESIAN_POINT('Ctrl Pts',(26.48,-0.888114184637538,-0.473248637986891));
#18640=CARTESIAN_POINT('Ctrl Pts',(26.48,-0.899697335364076,-0.45008966299909));
#18641=CARTESIAN_POINT('Ctrl Pts',(26.48,-0.907516953536694,-0.434455372645004));
#18642=CARTESIAN_POINT('Ctrl Pts',(26.48,-0.914935139614922,-0.418564567576599));
#18643=CARTESIAN_POINT('Ctrl Pts',(26.48,-0.921961425695318,-0.402384956514707));
#18644=CARTESIAN_POINT('Ctrl Pts',(26.48,-0.927972444434527,-0.388543227872672));
#18645=CARTESIAN_POINT('Ctrl Pts',(26.48,-0.933698695491516,-0.374483334307272));
#18646=CARTESIAN_POINT('Ctrl Pts',(26.48,-0.939125947132214,-0.360221022028348));
#18647=CARTESIAN_POINT('Ctrl Pts',(26.48,-0.950750727055155,-0.329672182134602));
#18648=CARTESIAN_POINT('Ctrl Pts',(26.48,-0.960996612202744,-0.298202563482207));
#18649=CARTESIAN_POINT('Ctrl Pts',(26.48,-0.969723021334668,-0.266062967888056));
#18650=CARTESIAN_POINT('Ctrl Pts',(26.48,-0.976571193622196,-0.240840968259932));
#18651=CARTESIAN_POINT('Ctrl Pts',(26.48,-0.982484355231731,-0.215207226664101));
#18652=CARTESIAN_POINT('Ctrl Pts',(26.48,-0.987413304183645,-0.189294788555209));
#18653=CARTESIAN_POINT('Ctrl Pts',(26.48,-0.995623316750138,-0.146133164327012));
#18654=CARTESIAN_POINT('Ctrl Pts',(26.48,-1.00110756323152,-0.102194463140761));
#18655=CARTESIAN_POINT('Ctrl Pts',(26.48,-1.00372609935242,-0.057857128426423));
#18656=CARTESIAN_POINT('Ctrl Pts',(26.48,-1.00518150971684,-0.0332139638893522));
#18657=CARTESIAN_POINT('Ctrl Pts',(26.48,-1.00575153192558,-0.00844851123841294));
#18658=CARTESIAN_POINT('Ctrl Pts',(26.48,-1.00541187048368,0.0163701440036105));
#18659=CARTESIAN_POINT('Ctrl Pts',(26.48,-1.00518113428977,0.0332297616765972));
#18660=CARTESIAN_POINT('Ctrl Pts',(26.48,-1.00453040362454,0.0501168621315424));
#18661=CARTESIAN_POINT('Ctrl Pts',(26.48,-1.00345271164585,0.0669993261012208));
#18662=CARTESIAN_POINT('Ctrl Pts',(26.48,-1.00154962283086,0.0968119525153273));
#18663=CARTESIAN_POINT('Ctrl Pts',(26.48,-0.998312161314223,0.126597561590713));
#18664=CARTESIAN_POINT('Ctrl Pts',(26.48,-0.993741374083221,0.156094322123882));
#18665=CARTESIAN_POINT('Ctrl Pts',(26.48,-0.990679445388345,0.175853933087574));
#18666=CARTESIAN_POINT('Ctrl Pts',(26.48,-0.987020222988573,0.195483943145631));
#18667=CARTESIAN_POINT('Ctrl Pts',(26.48,-0.982776892962407,0.214908302908513));
#18668=CARTESIAN_POINT('Ctrl Pts',(26.48,-0.979330409756623,0.230684999345762));
#18669=CARTESIAN_POINT('Ctrl Pts',(26.48,-0.975498863804595,0.246325981007969));
#18670=CARTESIAN_POINT('Ctrl Pts',(26.48,-0.971306281242836,0.261795413288413));
#18671=CARTESIAN_POINT('Ctrl Pts',(26.48,-0.964182057014329,0.288081766062669));
#18672=CARTESIAN_POINT('Ctrl Pts',(26.48,-0.956018523881081,0.313881868010713));
#18673=CARTESIAN_POINT('Ctrl Pts',(26.48,-0.946844595399094,0.339276864237371));
#18674=CARTESIAN_POINT('Ctrl Pts',(26.48,-0.937561817050851,0.364973175429396));
#18675=CARTESIAN_POINT('Ctrl Pts',(26.48,-0.927244222465897,0.390255339892911));
#18676=CARTESIAN_POINT('Ctrl Pts',(26.48,-0.915871127948933,0.415191450231033));
#18677=CARTESIAN_POINT('Ctrl Pts',(26.48,-0.908944434263715,0.430378591932469));
#18678=CARTESIAN_POINT('Ctrl Pts',(26.48,-0.901625262147177,0.445437023251559));
#18679=CARTESIAN_POINT('Ctrl Pts',(26.48,-0.8939005627167,0.460377710173327));
#18680=CARTESIAN_POINT('Ctrl Pts',(26.48,0.301306390501209,-0.959765445450956));
#18681=CARTESIAN_POINT('Ctrl Pts',(26.4799732521317,0.300594091921396,-0.959942135954256));
#18682=CARTESIAN_POINT('Ctrl Pts',(26.4799465042634,0.299881646280774,-0.960118045048617));
#18683=CARTESIAN_POINT('Ctrl Pts',(26.4799197563952,0.299169055382355,-0.960293172620655));
#18684=CARTESIAN_POINT('Origin',(26.48,0.,0.));
#18685=CARTESIAN_POINT('Origin',(26.48,-1.082531754731,0.625));
#18686=CARTESIAN_POINT('',(26.48,-1.082531754731,0.625));
#18687=CARTESIAN_POINT('Origin',(32.48,0.,0.));
#18688=CARTESIAN_POINT('Ctrl Pts',(28.05053792796,0.4083111129797,-0.9194117875127));
#18689=CARTESIAN_POINT('Ctrl Pts',(28.03432447383,0.2001723500546,-1.011846288678));
#18690=CARTESIAN_POINT('Ctrl Pts',(28.00189756559,-0.2804297640578,-1.049445986524));
#18691=CARTESIAN_POINT('Ctrl Pts',(27.95325720323,-0.8775530509839,-0.6404167031148));
#18692=CARTESIAN_POINT('Ctrl Pts',(27.90461684086,-1.085053538068,0.05289845296993));
#18693=CARTESIAN_POINT('Ctrl Pts',(27.85597647849,-0.8110736778472,0.722716801219));
#18694=CARTESIAN_POINT('Ctrl Pts',(27.80733611613,-0.1771401075638,1.071811347771));
#18695=CARTESIAN_POINT('Ctrl Pts',(27.75869575376,0.5354018004738,0.9452525615612));
#18696=CARTESIAN_POINT('Ctrl Pts',(27.7100553914,1.010342345254,0.3992070424407));
#18697=CARTESIAN_POINT('Ctrl Pts',(27.66141502903,1.036909749886,-0.3239999391312));
#18698=CARTESIAN_POINT('Ctrl Pts',(27.61277466667,0.6033141627449,-0.9034211828672));
#18699=CARTESIAN_POINT('Ctrl Pts',(27.5641343043,-0.09802209198353,-1.081919350877));
#18700=CARTESIAN_POINT('Ctrl Pts',(27.51549394194,-0.7558577907832,-0.7802799567664));
#18701=CARTESIAN_POINT('Ctrl Pts',(27.46685357957,-1.078256551794,-0.1323654788032));
#18702=CARTESIAN_POINT('Ctrl Pts',(27.41821321721,-0.9221432409161,0.5742905662964));
#18703=CARTESIAN_POINT('Ctrl Pts',(27.36957285484,-0.3567983129049,1.026086144158));
#18704=CARTESIAN_POINT('Ctrl Pts',(27.32093249248,0.3668876885504,1.022521997474));
#18705=CARTESIAN_POINT('Ctrl Pts',(27.27229213011,0.9277551218377,0.5651798344144));
#18706=CARTESIAN_POINT('Ctrl Pts',(27.22365176775,1.076900479802,-0.1429796066949));
#18707=CARTESIAN_POINT('Ctrl Pts',(27.17501140538,0.7481355680915,-0.7876871098868));
#18708=CARTESIAN_POINT('Ctrl Pts',(27.12637104301,0.08736070952101,-1.082832359018));
#18709=CARTESIAN_POINT('Ctrl Pts',(27.07773068065,-0.6121833585662,-0.8974348705957));
#18710=CARTESIAN_POINT('Ctrl Pts',(27.02909031828,-1.040050777064,-0.3137709227251));
#18711=CARTESIAN_POINT('Ctrl Pts',(26.98044995592,-1.006361203543,0.4091392676381));
#18712=CARTESIAN_POINT('Ctrl Pts',(26.93180959355,-0.5260654973531,0.9504803549345));
#18713=CARTESIAN_POINT('Ctrl Pts',(26.88316923119,0.1876891886185,1.07001427955));
#18714=CARTESIAN_POINT('Ctrl Pts',(26.83452886882,0.8181506349976,0.7146939595389));
#18715=CARTESIAN_POINT('Ctrl Pts',(26.78588850646,1.08553041707,0.04220434462485));
#18716=CARTESIAN_POINT('Ctrl Pts',(26.73724814409,0.8711708986611,-0.6490142126668));
#18717=CARTESIAN_POINT('Ctrl Pts',(26.68860778173,0.2701974812614,-1.052213574699));
#18718=CARTESIAN_POINT('Ctrl Pts',(26.63996741936,-0.4506740207088,-0.9884494695529));
#18719=CARTESIAN_POINT('Ctrl Pts',(26.591327057,-0.971585047505,-0.4860611138367));
#18720=CARTESIAN_POINT('Ctrl Pts',(26.54268669463,-1.061169801454,0.2321559469013));
#18721=CARTESIAN_POINT('Ctrl Pts',(26.51025978639,-0.8073213367869,0.641976744755));
#18722=CARTESIAN_POINT('Ctrl Pts',(26.49404633227,-0.6297166412204,0.7845335886819));
#18723=CARTESIAN_POINT('Ctrl Pts',(27.96513432978,0.4083111129797,-0.9194117875127));
#18724=CARTESIAN_POINT('Ctrl Pts',(27.94892087565,0.2001723500546,-1.011846288678));
#18725=CARTESIAN_POINT('Ctrl Pts',(27.91649396741,-0.2804297640578,-1.049445986524));
#18726=CARTESIAN_POINT('Ctrl Pts',(27.86785360505,-0.8775530509839,-0.6404167031148));
#18727=CARTESIAN_POINT('Ctrl Pts',(27.81921324268,-1.085053538068,0.05289845296993));
#18728=CARTESIAN_POINT('Ctrl Pts',(27.77057288031,-0.8110736778472,0.722716801219));
#18729=CARTESIAN_POINT('Ctrl Pts',(27.72193251795,-0.1771401075638,1.071811347771));
#18730=CARTESIAN_POINT('Ctrl Pts',(27.67329215558,0.5354018004738,0.9452525615612));
#18731=CARTESIAN_POINT('Ctrl Pts',(27.62465179322,1.010342345254,0.3992070424407));
#18732=CARTESIAN_POINT('Ctrl Pts',(27.57601143085,1.036909749886,-0.3239999391312));
#18733=CARTESIAN_POINT('Ctrl Pts',(27.52737106849,0.6033141627449,-0.9034211828672));
#18734=CARTESIAN_POINT('Ctrl Pts',(27.47873070612,-0.09802209198353,-1.081919350877));
#18735=CARTESIAN_POINT('Ctrl Pts',(27.43009034376,-0.7558577907832,-0.7802799567664));
#18736=CARTESIAN_POINT('Ctrl Pts',(27.38144998139,-1.078256551794,-0.1323654788032));
#18737=CARTESIAN_POINT('Ctrl Pts',(27.33280961903,-0.9221432409161,0.5742905662964));
#18738=CARTESIAN_POINT('Ctrl Pts',(27.28416925666,-0.3567983129049,1.026086144158));
#18739=CARTESIAN_POINT('Ctrl Pts',(27.2355288943,0.3668876885504,1.022521997474));
#18740=CARTESIAN_POINT('Ctrl Pts',(27.18688853193,0.9277551218377,0.5651798344144));
#18741=CARTESIAN_POINT('Ctrl Pts',(27.13824816957,1.076900479802,-0.1429796066949));
#18742=CARTESIAN_POINT('Ctrl Pts',(27.0896078072,0.7481355680915,-0.7876871098868));
#18743=CARTESIAN_POINT('Ctrl Pts',(27.04096744483,0.08736070952101,-1.082832359018));
#18744=CARTESIAN_POINT('Ctrl Pts',(26.99232708247,-0.6121833585662,-0.8974348705957));
#18745=CARTESIAN_POINT('Ctrl Pts',(26.9436867201,-1.040050777064,-0.3137709227251));
#18746=CARTESIAN_POINT('Ctrl Pts',(26.89504635774,-1.006361203543,0.4091392676381));
#18747=CARTESIAN_POINT('Ctrl Pts',(26.84640599537,-0.5260654973531,0.9504803549345));
#18748=CARTESIAN_POINT('Ctrl Pts',(26.79776563301,0.1876891886185,1.07001427955));
#18749=CARTESIAN_POINT('Ctrl Pts',(26.74912527064,0.8181506349976,0.7146939595389));
#18750=CARTESIAN_POINT('Ctrl Pts',(26.70048490828,1.08553041707,0.04220434462485));
#18751=CARTESIAN_POINT('Ctrl Pts',(26.65184454591,0.8711708986611,-0.6490142126668));
#18752=CARTESIAN_POINT('Ctrl Pts',(26.60320418355,0.2701974812614,-1.052213574699));
#18753=CARTESIAN_POINT('Ctrl Pts',(26.55456382118,-0.4506740207088,-0.9884494695529));
#18754=CARTESIAN_POINT('Ctrl Pts',(26.50592345882,-0.971585047505,-0.4860611138367));
#18755=CARTESIAN_POINT('Ctrl Pts',(26.45728309645,-1.061169801454,0.2321559469013));
#18756=CARTESIAN_POINT('Ctrl Pts',(26.42485618821,-0.8073213367869,0.641976744755));
#18757=CARTESIAN_POINT('Ctrl Pts',(26.40864273409,-0.6297166412204,0.7845335886819));
#18758=CARTESIAN_POINT('Ctrl Pts',(27.8797307316,0.4083111129797,-0.9194117875127));
#18759=CARTESIAN_POINT('Ctrl Pts',(27.86351727747,0.2001723500546,-1.011846288678));
#18760=CARTESIAN_POINT('Ctrl Pts',(27.83109036923,-0.2804297640578,-1.049445986524));
#18761=CARTESIAN_POINT('Ctrl Pts',(27.78245000687,-0.8775530509839,-0.6404167031148));
#18762=CARTESIAN_POINT('Ctrl Pts',(27.7338096445,-1.085053538068,0.05289845296993));
#18763=CARTESIAN_POINT('Ctrl Pts',(27.68516928214,-0.8110736778472,0.722716801219));
#18764=CARTESIAN_POINT('Ctrl Pts',(27.63652891977,-0.1771401075638,1.071811347771));
#18765=CARTESIAN_POINT('Ctrl Pts',(27.5878885574,0.5354018004738,0.9452525615612));
#18766=CARTESIAN_POINT('Ctrl Pts',(27.53924819504,1.010342345254,0.3992070424407));
#18767=CARTESIAN_POINT('Ctrl Pts',(27.49060783267,1.036909749886,-0.3239999391312));
#18768=CARTESIAN_POINT('Ctrl Pts',(27.44196747031,0.6033141627449,-0.9034211828672));
#18769=CARTESIAN_POINT('Ctrl Pts',(27.39332710794,-0.09802209198353,-1.081919350877));
#18770=CARTESIAN_POINT('Ctrl Pts',(27.34468674558,-0.7558577907832,-0.7802799567664));
#18771=CARTESIAN_POINT('Ctrl Pts',(27.29604638321,-1.078256551794,-0.1323654788032));
#18772=CARTESIAN_POINT('Ctrl Pts',(27.24740602085,-0.9221432409161,0.5742905662964));
#18773=CARTESIAN_POINT('Ctrl Pts',(27.19876565848,-0.3567983129049,1.026086144158));
#18774=CARTESIAN_POINT('Ctrl Pts',(27.15012529612,0.3668876885504,1.022521997474));
#18775=CARTESIAN_POINT('Ctrl Pts',(27.10148493375,0.9277551218377,0.5651798344144));
#18776=CARTESIAN_POINT('Ctrl Pts',(27.05284457139,1.076900479802,-0.1429796066949));
#18777=CARTESIAN_POINT('Ctrl Pts',(27.00420420902,0.7481355680915,-0.7876871098868));
#18778=CARTESIAN_POINT('Ctrl Pts',(26.95556384666,0.08736070952101,-1.082832359018));
#18779=CARTESIAN_POINT('Ctrl Pts',(26.90692348429,-0.6121833585662,-0.8974348705957));
#18780=CARTESIAN_POINT('Ctrl Pts',(26.85828312192,-1.040050777064,-0.3137709227251));
#18781=CARTESIAN_POINT('Ctrl Pts',(26.80964275956,-1.006361203543,0.4091392676381));
#18782=CARTESIAN_POINT('Ctrl Pts',(26.76100239719,-0.5260654973531,0.9504803549345));
#18783=CARTESIAN_POINT('Ctrl Pts',(26.71236203483,0.1876891886185,1.07001427955));
#18784=CARTESIAN_POINT('Ctrl Pts',(26.66372167246,0.8181506349976,0.7146939595389));
#18785=CARTESIAN_POINT('Ctrl Pts',(26.6150813101,1.08553041707,0.04220434462485));
#18786=CARTESIAN_POINT('Ctrl Pts',(26.56644094773,0.8711708986611,-0.6490142126668));
#18787=CARTESIAN_POINT('Ctrl Pts',(26.51780058537,0.2701974812614,-1.052213574699));
#18788=CARTESIAN_POINT('Ctrl Pts',(26.469160223,-0.4506740207088,-0.9884494695529));
#18789=CARTESIAN_POINT('Ctrl Pts',(26.42051986064,-0.971585047505,-0.4860611138367));
#18790=CARTESIAN_POINT('Ctrl Pts',(26.37187949827,-1.061169801454,0.2321559469013));
#18791=CARTESIAN_POINT('Ctrl Pts',(26.33945259003,-0.8073213367869,0.641976744755));
#18792=CARTESIAN_POINT('Ctrl Pts',(26.32323913591,-0.6297166412204,0.7845335886819));
#18793=CARTESIAN_POINT('Ctrl Pts',(27.79432713342,0.4083111129797,-0.9194117875127));
#18794=CARTESIAN_POINT('Ctrl Pts',(27.7781136793,0.2001723500546,-1.011846288678));
#18795=CARTESIAN_POINT('Ctrl Pts',(27.74568677105,-0.2804297640578,-1.049445986524));
#18796=CARTESIAN_POINT('Ctrl Pts',(27.69704640869,-0.8775530509839,-0.6404167031148));
#18797=CARTESIAN_POINT('Ctrl Pts',(27.64840604632,-1.085053538068,0.05289845296993));
#18798=CARTESIAN_POINT('Ctrl Pts',(27.59976568396,-0.8110736778472,0.722716801219));
#18799=CARTESIAN_POINT('Ctrl Pts',(27.55112532159,-0.1771401075638,1.071811347771));
#18800=CARTESIAN_POINT('Ctrl Pts',(27.50248495923,0.5354018004738,0.9452525615612));
#18801=CARTESIAN_POINT('Ctrl Pts',(27.45384459686,1.010342345254,0.3992070424407));
#18802=CARTESIAN_POINT('Ctrl Pts',(27.40520423449,1.036909749886,-0.3239999391312));
#18803=CARTESIAN_POINT('Ctrl Pts',(27.35656387213,0.6033141627449,-0.9034211828672));
#18804=CARTESIAN_POINT('Ctrl Pts',(27.30792350976,-0.09802209198353,-1.081919350877));
#18805=CARTESIAN_POINT('Ctrl Pts',(27.2592831474,-0.7558577907832,-0.7802799567664));
#18806=CARTESIAN_POINT('Ctrl Pts',(27.21064278503,-1.078256551794,-0.1323654788032));
#18807=CARTESIAN_POINT('Ctrl Pts',(27.16200242267,-0.9221432409161,0.5742905662964));
#18808=CARTESIAN_POINT('Ctrl Pts',(27.1133620603,-0.3567983129049,1.026086144158));
#18809=CARTESIAN_POINT('Ctrl Pts',(27.06472169794,0.3668876885504,1.022521997474));
#18810=CARTESIAN_POINT('Ctrl Pts',(27.01608133557,0.9277551218377,0.5651798344144));
#18811=CARTESIAN_POINT('Ctrl Pts',(26.96744097321,1.076900479802,-0.1429796066949));
#18812=CARTESIAN_POINT('Ctrl Pts',(26.91880061084,0.7481355680915,-0.7876871098868));
#18813=CARTESIAN_POINT('Ctrl Pts',(26.87016024848,0.08736070952101,-1.082832359018));
#18814=CARTESIAN_POINT('Ctrl Pts',(26.82151988611,-0.6121833585662,-0.8974348705957));
#18815=CARTESIAN_POINT('Ctrl Pts',(26.77287952375,-1.040050777064,-0.3137709227251));
#18816=CARTESIAN_POINT('Ctrl Pts',(26.72423916138,-1.006361203543,0.4091392676381));
#18817=CARTESIAN_POINT('Ctrl Pts',(26.67559879901,-0.5260654973531,0.9504803549345));
#18818=CARTESIAN_POINT('Ctrl Pts',(26.62695843665,0.1876891886185,1.07001427955));
#18819=CARTESIAN_POINT('Ctrl Pts',(26.57831807428,0.8181506349976,0.7146939595389));
#18820=CARTESIAN_POINT('Ctrl Pts',(26.52967771192,1.08553041707,0.04220434462485));
#18821=CARTESIAN_POINT('Ctrl Pts',(26.48103734955,0.8711708986611,-0.6490142126668));
#18822=CARTESIAN_POINT('Ctrl Pts',(26.43239698719,0.2701974812614,-1.052213574699));
#18823=CARTESIAN_POINT('Ctrl Pts',(26.38375662482,-0.4506740207088,-0.9884494695529));
#18824=CARTESIAN_POINT('Ctrl Pts',(26.33511626246,-0.971585047505,-0.4860611138367));
#18825=CARTESIAN_POINT('Ctrl Pts',(26.28647590009,-1.061169801454,0.2321559469013));
#18826=CARTESIAN_POINT('Ctrl Pts',(26.25404899185,-0.8073213367869,0.641976744755));
#18827=CARTESIAN_POINT('Ctrl Pts',(26.23783553773,-0.6297166412204,0.7845335886819));
#18828=CARTESIAN_POINT('',(27.97662653432,-3.364114380046E-14,-1.006));
#18829=CARTESIAN_POINT('Ctrl Pts',(29.55060539727,0.5913119638062,0.8138710963412));
#18830=CARTESIAN_POINT('Ctrl Pts',(29.53435539727,0.7759734579399,0.6797066675681));
#18831=CARTESIAN_POINT('Ctrl Pts',(29.50185539727,1.049589852444,0.2813441556141));
#18832=CARTESIAN_POINT('Ctrl Pts',(29.45310539727,0.9928036170159,-0.4420327897627));
#18833=CARTESIAN_POINT('Ctrl Pts',(29.40435539727,0.4933560618227,-0.9682753741689));
#18834=CARTESIAN_POINT('Ctrl Pts',(29.35560539727,-0.2259412078788,-1.062981093563));
#18835=CARTESIAN_POINT('Ctrl Pts',(29.30685539727,-0.8445461960836,-0.6838991696093));
#18836=CARTESIAN_POINT('Ctrl Pts',(29.25810539727,-1.086727031141,-1.08376590563E-7));
#18837=CARTESIAN_POINT('Ctrl Pts',(29.20935539727,-0.8445456793518,0.6838996031158));
#18838=CARTESIAN_POINT('Ctrl Pts',(29.16060539727,-0.2259432748058,1.06297957629));
#18839=CARTESIAN_POINT('Ctrl Pts',(29.11185539727,0.4933638127993,0.9682810097529));
#18840=CARTESIAN_POINT('Ctrl Pts',(29.06310539727,0.9927746800368,0.4420117646993));
#18841=CARTESIAN_POINT('Ctrl Pts',(29.01435539727,1.049697849384,-0.2812656909448));
#18842=CARTESIAN_POINT('Ctrl Pts',(28.96560539727,0.6387622099061,-0.8791807571591));
#18843=CARTESIAN_POINT('Ctrl Pts',(28.91685539727,-0.05687490617148,-1.085237858466));
#18844=CARTESIAN_POINT('Ctrl Pts',(28.86810539727,-0.7271624171027,-0.807595680755));
#18845=CARTESIAN_POINT('Ctrl Pts',(28.81935539727,-1.0733477654,-0.1700015850954));
#18846=CARTESIAN_POINT('Ctrl Pts',(28.77060539727,-0.9411333451298,0.5433635901541));
#18847=CARTESIAN_POINT('Ctrl Pts',(28.72185539727,-0.3894481913236,1.014547224479));
#18848=CARTESIAN_POINT('Ctrl Pts',(28.67310539727,0.3358171669691,1.033538966266));
#18849=CARTESIAN_POINT('Ctrl Pts',(28.62435539727,0.9114061014946,0.5918740428154));
#18850=CARTESIAN_POINT('Ctrl Pts',(28.57560539727,1.080773975171,-0.1135939221767));
#18851=CARTESIAN_POINT('Ctrl Pts',(28.52685539727,0.7684321582634,-0.7684321583925));
#18852=CARTESIAN_POINT('Ctrl Pts',(28.47810539727,0.1135939230171,-1.080773975495));
#18853=CARTESIAN_POINT('Ctrl Pts',(28.42935539727,-0.5918740460484,-0.9114061000685));
#18854=CARTESIAN_POINT('Ctrl Pts',(28.38060539727,-1.033538954174,-0.3358171723489));
#18855=CARTESIAN_POINT('Ctrl Pts',(28.33185539727,-1.014547269612,0.3894482114172));
#18856=CARTESIAN_POINT('Ctrl Pts',(28.28310539727,-0.5433634217136,0.9411332701358));
#18857=CARTESIAN_POINT('Ctrl Pts',(28.23435539727,0.170000956467,1.073348045283));
#18858=CARTESIAN_POINT('Ctrl Pts',(28.18560539727,0.8075980268285,0.7271613725661));
#18859=CARTESIAN_POINT('Ctrl Pts',(28.13685539727,1.0852291028,0.05687880443492));
#18860=CARTESIAN_POINT('Ctrl Pts',(28.08810539727,0.8792134337481,-0.6387767584236));
#18861=CARTESIAN_POINT('Ctrl Pts',(28.03935539727,0.281143740254,-1.049643553578));
#18862=CARTESIAN_POINT('Ctrl Pts',(28.00685539727,-0.2006565122658,-1.011866061022));
#18863=CARTESIAN_POINT('Ctrl Pts',(27.99060539727,-0.4091770629343,-0.9190267303884));
#18864=CARTESIAN_POINT('Ctrl Pts',(29.46520179909,0.5913119638062,0.8138710963412));
#18865=CARTESIAN_POINT('Ctrl Pts',(29.44895179909,0.7759734579399,0.6797066675681));
#18866=CARTESIAN_POINT('Ctrl Pts',(29.41645179909,1.049589852444,0.2813441556141));
#18867=CARTESIAN_POINT('Ctrl Pts',(29.36770179909,0.9928036170159,-0.4420327897627));
#18868=CARTESIAN_POINT('Ctrl Pts',(29.31895179909,0.4933560618227,-0.9682753741689));
#18869=CARTESIAN_POINT('Ctrl Pts',(29.27020179909,-0.2259412078788,-1.062981093563));
#18870=CARTESIAN_POINT('Ctrl Pts',(29.22145179909,-0.8445461960836,-0.6838991696093));
#18871=CARTESIAN_POINT('Ctrl Pts',(29.17270179909,-1.086727031141,-1.08376590563E-7));
#18872=CARTESIAN_POINT('Ctrl Pts',(29.12395179909,-0.8445456793518,0.6838996031158));
#18873=CARTESIAN_POINT('Ctrl Pts',(29.07520179909,-0.2259432748058,1.06297957629));
#18874=CARTESIAN_POINT('Ctrl Pts',(29.02645179909,0.4933638127993,0.9682810097529));
#18875=CARTESIAN_POINT('Ctrl Pts',(28.97770179909,0.9927746800368,0.4420117646993));
#18876=CARTESIAN_POINT('Ctrl Pts',(28.92895179909,1.049697849384,-0.2812656909448));
#18877=CARTESIAN_POINT('Ctrl Pts',(28.88020179909,0.6387622099061,-0.8791807571591));
#18878=CARTESIAN_POINT('Ctrl Pts',(28.83145179909,-0.05687490617148,-1.085237858466));
#18879=CARTESIAN_POINT('Ctrl Pts',(28.78270179909,-0.7271624171027,-0.807595680755));
#18880=CARTESIAN_POINT('Ctrl Pts',(28.73395179909,-1.0733477654,-0.1700015850954));
#18881=CARTESIAN_POINT('Ctrl Pts',(28.68520179909,-0.9411333451298,0.5433635901541));
#18882=CARTESIAN_POINT('Ctrl Pts',(28.63645179909,-0.3894481913236,1.014547224479));
#18883=CARTESIAN_POINT('Ctrl Pts',(28.58770179909,0.3358171669691,1.033538966266));
#18884=CARTESIAN_POINT('Ctrl Pts',(28.53895179909,0.9114061014946,0.5918740428154));
#18885=CARTESIAN_POINT('Ctrl Pts',(28.49020179909,1.080773975171,-0.1135939221767));
#18886=CARTESIAN_POINT('Ctrl Pts',(28.44145179909,0.7684321582634,-0.7684321583925));
#18887=CARTESIAN_POINT('Ctrl Pts',(28.39270179909,0.1135939230171,-1.080773975495));
#18888=CARTESIAN_POINT('Ctrl Pts',(28.34395179909,-0.5918740460484,-0.9114061000685));
#18889=CARTESIAN_POINT('Ctrl Pts',(28.29520179909,-1.033538954174,-0.3358171723489));
#18890=CARTESIAN_POINT('Ctrl Pts',(28.24645179909,-1.014547269612,0.3894482114172));
#18891=CARTESIAN_POINT('Ctrl Pts',(28.19770179909,-0.5433634217136,0.9411332701358));
#18892=CARTESIAN_POINT('Ctrl Pts',(28.14895179909,0.170000956467,1.073348045283));
#18893=CARTESIAN_POINT('Ctrl Pts',(28.10020179909,0.8075980268285,0.7271613725661));
#18894=CARTESIAN_POINT('Ctrl Pts',(28.05145179909,1.0852291028,0.05687880443492));
#18895=CARTESIAN_POINT('Ctrl Pts',(28.00270179909,0.8792134337481,-0.6387767584236));
#18896=CARTESIAN_POINT('Ctrl Pts',(27.95395179909,0.281143740254,-1.049643553578));
#18897=CARTESIAN_POINT('Ctrl Pts',(27.92145179909,-0.2006565122658,-1.011866061022));
#18898=CARTESIAN_POINT('Ctrl Pts',(27.90520179909,-0.4091770629343,-0.9190267303884));
#18899=CARTESIAN_POINT('Ctrl Pts',(29.37979820091,0.5913119638062,0.8138710963412));
#18900=CARTESIAN_POINT('Ctrl Pts',(29.36354820091,0.7759734579399,0.6797066675681));
#18901=CARTESIAN_POINT('Ctrl Pts',(29.33104820091,1.049589852444,0.2813441556141));
#18902=CARTESIAN_POINT('Ctrl Pts',(29.28229820091,0.9928036170159,-0.4420327897627));
#18903=CARTESIAN_POINT('Ctrl Pts',(29.23354820091,0.4933560618227,-0.9682753741689));
#18904=CARTESIAN_POINT('Ctrl Pts',(29.18479820091,-0.2259412078788,-1.062981093563));
#18905=CARTESIAN_POINT('Ctrl Pts',(29.13604820091,-0.8445461960836,-0.6838991696093));
#18906=CARTESIAN_POINT('Ctrl Pts',(29.08729820091,-1.086727031141,-1.083765901744E-7));
#18907=CARTESIAN_POINT('Ctrl Pts',(29.03854820091,-0.8445456793518,0.6838996031158));
#18908=CARTESIAN_POINT('Ctrl Pts',(28.98979820091,-0.2259432748058,1.06297957629));
#18909=CARTESIAN_POINT('Ctrl Pts',(28.94104820091,0.4933638127993,0.9682810097529));
#18910=CARTESIAN_POINT('Ctrl Pts',(28.89229820091,0.9927746800368,0.4420117646993));
#18911=CARTESIAN_POINT('Ctrl Pts',(28.84354820091,1.049697849384,-0.2812656909448));
#18912=CARTESIAN_POINT('Ctrl Pts',(28.79479820091,0.6387622099061,-0.8791807571591));
#18913=CARTESIAN_POINT('Ctrl Pts',(28.74604820091,-0.05687490617148,-1.085237858466));
#18914=CARTESIAN_POINT('Ctrl Pts',(28.69729820091,-0.7271624171027,-0.807595680755));
#18915=CARTESIAN_POINT('Ctrl Pts',(28.64854820091,-1.0733477654,-0.1700015850954));
#18916=CARTESIAN_POINT('Ctrl Pts',(28.59979820091,-0.9411333451298,0.5433635901541));
#18917=CARTESIAN_POINT('Ctrl Pts',(28.55104820091,-0.3894481913236,1.014547224479));
#18918=CARTESIAN_POINT('Ctrl Pts',(28.50229820091,0.3358171669691,1.033538966266));
#18919=CARTESIAN_POINT('Ctrl Pts',(28.45354820091,0.9114061014946,0.5918740428154));
#18920=CARTESIAN_POINT('Ctrl Pts',(28.40479820091,1.080773975171,-0.1135939221767));
#18921=CARTESIAN_POINT('Ctrl Pts',(28.35604820091,0.7684321582634,-0.7684321583925));
#18922=CARTESIAN_POINT('Ctrl Pts',(28.30729820091,0.1135939230171,-1.080773975495));
#18923=CARTESIAN_POINT('Ctrl Pts',(28.25854820091,-0.5918740460484,-0.9114061000685));
#18924=CARTESIAN_POINT('Ctrl Pts',(28.20979820091,-1.033538954174,-0.3358171723489));
#18925=CARTESIAN_POINT('Ctrl Pts',(28.16104820091,-1.014547269612,0.3894482114172));
#18926=CARTESIAN_POINT('Ctrl Pts',(28.11229820091,-0.5433634217136,0.9411332701358));
#18927=CARTESIAN_POINT('Ctrl Pts',(28.06354820091,0.170000956467,1.073348045283));
#18928=CARTESIAN_POINT('Ctrl Pts',(28.01479820091,0.8075980268285,0.7271613725661));
#18929=CARTESIAN_POINT('Ctrl Pts',(27.96604820091,1.0852291028,0.05687880443492));
#18930=CARTESIAN_POINT('Ctrl Pts',(27.91729820091,0.8792134337481,-0.6387767584236));
#18931=CARTESIAN_POINT('Ctrl Pts',(27.86854820091,0.281143740254,-1.049643553578));
#18932=CARTESIAN_POINT('Ctrl Pts',(27.83604820091,-0.2006565122658,-1.011866061022));
#18933=CARTESIAN_POINT('Ctrl Pts',(27.81979820091,-0.4091770629343,-0.9190267303884));
#18934=CARTESIAN_POINT('Ctrl Pts',(29.29439460273,0.5913119638062,0.8138710963412));
#18935=CARTESIAN_POINT('Ctrl Pts',(29.27814460273,0.7759734579399,0.6797066675681));
#18936=CARTESIAN_POINT('Ctrl Pts',(29.24564460273,1.049589852444,0.2813441556141));
#18937=CARTESIAN_POINT('Ctrl Pts',(29.19689460273,0.9928036170159,-0.4420327897627));
#18938=CARTESIAN_POINT('Ctrl Pts',(29.14814460273,0.4933560618227,-0.9682753741689));
#18939=CARTESIAN_POINT('Ctrl Pts',(29.09939460273,-0.2259412078788,-1.062981093563));
#18940=CARTESIAN_POINT('Ctrl Pts',(29.05064460273,-0.8445461960836,-0.6838991696093));
#18941=CARTESIAN_POINT('Ctrl Pts',(29.00189460273,-1.086727031141,-1.083765901744E-7));
#18942=CARTESIAN_POINT('Ctrl Pts',(28.95314460273,-0.8445456793518,0.6838996031158));
#18943=CARTESIAN_POINT('Ctrl Pts',(28.90439460273,-0.2259432748058,1.06297957629));
#18944=CARTESIAN_POINT('Ctrl Pts',(28.85564460273,0.4933638127993,0.9682810097529));
#18945=CARTESIAN_POINT('Ctrl Pts',(28.80689460273,0.9927746800368,0.4420117646993));
#18946=CARTESIAN_POINT('Ctrl Pts',(28.75814460273,1.049697849384,-0.2812656909448));
#18947=CARTESIAN_POINT('Ctrl Pts',(28.70939460273,0.6387622099061,-0.8791807571591));
#18948=CARTESIAN_POINT('Ctrl Pts',(28.66064460273,-0.05687490617148,-1.085237858466));
#18949=CARTESIAN_POINT('Ctrl Pts',(28.61189460273,-0.7271624171027,-0.807595680755));
#18950=CARTESIAN_POINT('Ctrl Pts',(28.56314460273,-1.0733477654,-0.1700015850954));
#18951=CARTESIAN_POINT('Ctrl Pts',(28.51439460273,-0.9411333451298,0.5433635901541));
#18952=CARTESIAN_POINT('Ctrl Pts',(28.46564460273,-0.3894481913236,1.014547224479));
#18953=CARTESIAN_POINT('Ctrl Pts',(28.41689460273,0.3358171669691,1.033538966266));
#18954=CARTESIAN_POINT('Ctrl Pts',(28.36814460273,0.9114061014946,0.5918740428154));
#18955=CARTESIAN_POINT('Ctrl Pts',(28.31939460273,1.080773975171,-0.1135939221767));
#18956=CARTESIAN_POINT('Ctrl Pts',(28.27064460273,0.7684321582634,-0.7684321583925));
#18957=CARTESIAN_POINT('Ctrl Pts',(28.22189460273,0.1135939230171,-1.080773975495));
#18958=CARTESIAN_POINT('Ctrl Pts',(28.17314460273,-0.5918740460484,-0.9114061000685));
#18959=CARTESIAN_POINT('Ctrl Pts',(28.12439460273,-1.033538954174,-0.3358171723489));
#18960=CARTESIAN_POINT('Ctrl Pts',(28.07564460273,-1.014547269612,0.3894482114172));
#18961=CARTESIAN_POINT('Ctrl Pts',(28.02689460273,-0.5433634217136,0.9411332701358));
#18962=CARTESIAN_POINT('Ctrl Pts',(27.97814460273,0.170000956467,1.073348045283));
#18963=CARTESIAN_POINT('Ctrl Pts',(27.92939460273,0.8075980268285,0.7271613725661));
#18964=CARTESIAN_POINT('Ctrl Pts',(27.88064460273,1.0852291028,0.05687880443492));
#18965=CARTESIAN_POINT('Ctrl Pts',(27.83189460273,0.8792134337481,-0.6387767584236));
#18966=CARTESIAN_POINT('Ctrl Pts',(27.78314460273,0.281143740254,-1.049643553578));
#18967=CARTESIAN_POINT('Ctrl Pts',(27.75064460273,-0.2006565122658,-1.011866061022));
#18968=CARTESIAN_POINT('Ctrl Pts',(27.73439460273,-0.4091770629343,-0.9190267303884));
#18969=CARTESIAN_POINT('Origin',(-1.12,0.,0.));
#18970=CARTESIAN_POINT('',(-1.12,3.5,0.));
#18971=CARTESIAN_POINT('Origin',(-1.12,0.,0.));
#18972=CARTESIAN_POINT('Origin',(-1.12,0.,0.));
#18973=CARTESIAN_POINT('',(-2.12,0.,3.5));
#18974=CARTESIAN_POINT('',(-2.12,3.5,-4.28626379701574E-16));
#18975=CARTESIAN_POINT('Origin',(-2.12,0.,0.));
#18976=CARTESIAN_POINT('Origin',(-2.12,0.,0.));
#18977=CARTESIAN_POINT('',(-1.12,3.5,-4.28626379701574E-16));
#18978=CARTESIAN_POINT('Origin',(9.88,0.,0.));
#18979=CARTESIAN_POINT('',(-2.62,9.37349864163661E-32,7.65404249467096E-16));
#18980=CARTESIAN_POINT('Origin',(9.88,0.,0.));
#52136=UNCERTAINTY_MEASURE_WITH_UNIT(LENGTH_MEASURE(0.01),#52165,
'DISTANCE_ACCURACY_VALUE',
'Maximum model space distance between geometric entities at asserted c
onnectivities');
#52149=UNCERTAINTY_MEASURE_WITH_UNIT(LENGTH_MEASURE(0.01),#52165,
'DISTANCE_ACCURACY_VALUE',
'Maximum model space distance between geometric entities at asserted c
onnectivities');
#52151=(
GEOMETRIC_REPRESENTATION_CONTEXT(3)
GLOBAL_UNCERTAINTY_ASSIGNED_CONTEXT((#52136))
GLOBAL_UNIT_ASSIGNED_CONTEXT((#52165,#52167,#52168))
REPRESENTATION_CONTEXT('','3D')
);
#52164=(
GEOMETRIC_REPRESENTATION_CONTEXT(3)
GLOBAL_UNCERTAINTY_ASSIGNED_CONTEXT((#52149))
GLOBAL_UNIT_ASSIGNED_CONTEXT((#52165,#52167,#52168))
REPRESENTATION_CONTEXT('','3D')
);
#52165=(
LENGTH_UNIT()
NAMED_UNIT(*)
SI_UNIT(.MILLI.,.METRE.)
);
#52167=(
NAMED_UNIT(*)
PLANE_ANGLE_UNIT()
SI_UNIT($,.RADIAN.)
);
#52168=(
NAMED_UNIT(*)
SI_UNIT($,.STERADIAN.)
SOLID_ANGLE_UNIT()
);
#52170=SHAPE_DEFINITION_REPRESENTATION(#52184,#52211);
#52184=PRODUCT_DEFINITION_SHAPE('',$,#52226);
#52211=SHAPE_REPRESENTATION('',(#9276),#52151);
#52224=PRODUCT_DEFINITION_CONTEXT('part definition',#52268,'design');
#52226=PRODUCT_DEFINITION('Worm Shaft / Tuning Worm',
'Worm Shaft / Tuning Worm',#52240,#52224);
#52240=PRODUCT_DEFINITION_FORMATION('',$,#52271);
#52268=APPLICATION_CONTEXT('Managed model based 3d engineering');
#52269=PRODUCT_CONTEXT('part definition',#52268,'mechanical');
#52271=PRODUCT('Worm Shaft / Tuning Worm','Worm Shaft / Tuning Worm',
'NOT SPECIFIED',(#52269));
#52312=COLOUR_RGB('Grey',0.48,0.52,0.57);
#52313=FILL_AREA_STYLE_COLOUR('',#52312);
#52314=FILL_AREA_STYLE('',(#52313));
#52315=SURFACE_STYLE_FILL_AREA(#52314);
#52316=SURFACE_SIDE_STYLE('',(#52315));
#52317=SURFACE_STYLE_USAGE(.BOTH.,#52316);
#52318=PRESENTATION_STYLE_ASSIGNMENT((#52317));
ENDSEC;
END-ISO-10303-21;
